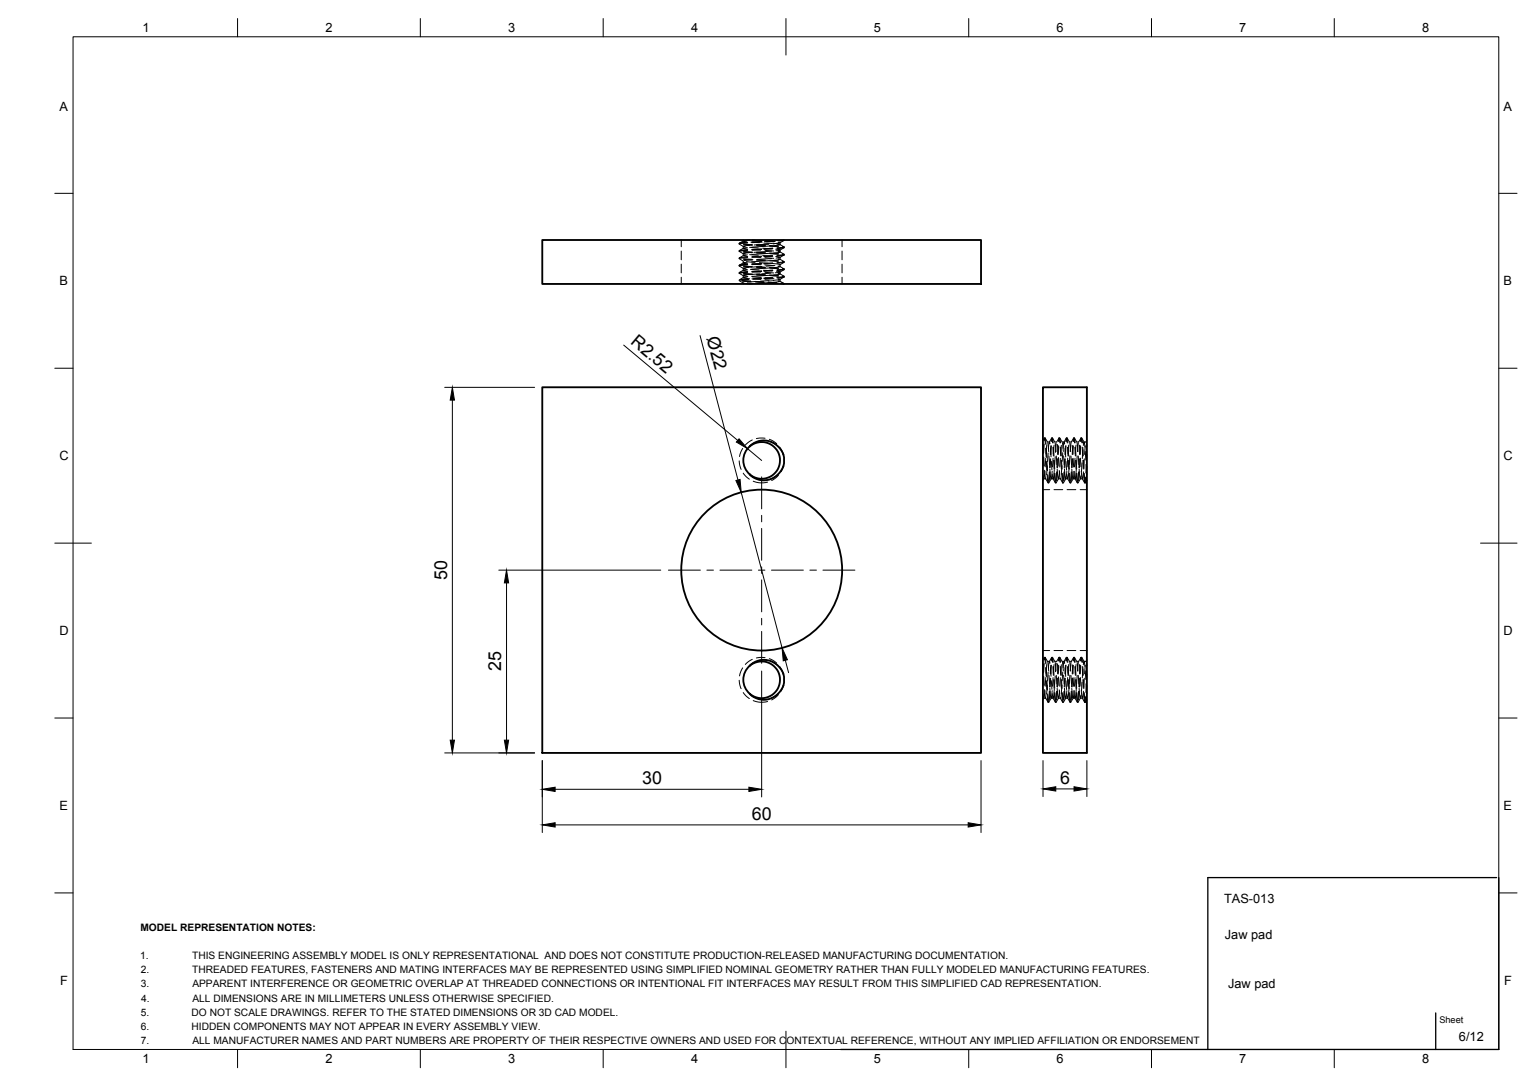
ISO-10303-21;
HEADER;
/* Generated by software containing ST-Developer
 * from STEP Tools, Inc. (www.steptools.com) 
 */

FILE_DESCRIPTION(
/* description */ (
'Independent guided parallel-jaw bracket clamp. Two12mm guide rods, re
placeable bronze sleeves, captured swiveling spindle, replaceable jaw 
pads and modeled M16x2 screw. Native slider/revolute joints linked2mm 
per revolution. Nominal opening0..122 with initial28mm. Base and two i
dentical supports welded. Standard fits, weld details and clamp load r
equire engineering selection.'),
/* implementation_level */ '2;1');

FILE_NAME(
/* name */ 'Jaw pad.step',
/* time_stamp */ '2026-11-14T09:15:44-08:00',
/* author */ (''),
/* organization */ (''),
/* preprocessor_version */ 'ST-DEVELOPER v20.2',
/* originating_system */ 'Autodesk Translation Framework v15.17.0.0',
/* authorisation */ '');

FILE_SCHEMA (('AUTOMOTIVE_DESIGN { 1 0 10303 214 3 1 1 }'));
ENDSEC;

DATA;
#10=MECHANICAL_DESIGN_GEOMETRIC_PRESENTATION_REPRESENTATION('',(#921),#105806);
#99=B_SPLINE_SURFACE_WITH_KNOTS('',3,3,((#87313,#87314,#87315,#87316,#87317,
#87318,#87319,#87320,#87321,#87322,#87323,#87324,#87325,#87326,#87327,#87328,
#87329,#87330,#87331,#87332,#87333,#87334,#87335,#87336,#87337,#87338,#87339,
#87340,#87341,#87342,#87343,#87344,#87345,#87346,#87347,#87348,#87349,#87350,
#87351,#87352,#87353,#87354,#87355),(#87356,#87357,#87358,#87359,#87360,
#87361,#87362,#87363,#87364,#87365,#87366,#87367,#87368,#87369,#87370,#87371,
#87372,#87373,#87374,#87375,#87376,#87377,#87378,#87379,#87380,#87381,#87382,
#87383,#87384,#87385,#87386,#87387,#87388,#87389,#87390,#87391,#87392,#87393,
#87394,#87395,#87396,#87397,#87398),(#87399,#87400,#87401,#87402,#87403,
#87404,#87405,#87406,#87407,#87408,#87409,#87410,#87411,#87412,#87413,#87414,
#87415,#87416,#87417,#87418,#87419,#87420,#87421,#87422,#87423,#87424,#87425,
#87426,#87427,#87428,#87429,#87430,#87431,#87432,#87433,#87434,#87435,#87436,
#87437,#87438,#87439,#87440,#87441),(#87442,#87443,#87444,#87445,#87446,
#87447,#87448,#87449,#87450,#87451,#87452,#87453,#87454,#87455,#87456,#87457,
#87458,#87459,#87460,#87461,#87462,#87463,#87464,#87465,#87466,#87467,#87468,
#87469,#87470,#87471,#87472,#87473,#87474,#87475,#87476,#87477,#87478,#87479,
#87480,#87481,#87482,#87483,#87484)),.UNSPECIFIED.,.F.,.F.,.F.,(4,4),(4,
1,1,1,1,1,1,1,1,1,1,1,1,1,1,1,1,1,1,1,1,1,1,1,1,1,1,1,1,1,1,1,1,1,1,1,1,
1,1,1,4),(-0.00051259176634298,0.0646339630657592),(11.8584762705415,12.8518902807105,
13.8447916991131,14.8376931175158,15.8305945359184,16.8234959543211,17.8163973727237,
18.8092987911264,19.802200209529,20.7951016279317,21.7880030463343,22.780904464737,
23.7738058831396,24.7667073015423,25.7596087199449,26.7525101383476,27.7454115567502,
28.7383129751529,29.7312143935555,30.7241158119582,31.7170172303608,32.7099186487635,
33.7028200671661,34.6957214855688,35.6886229039714,36.6815243223741,37.6744257407767,
38.6673271591794,39.660228577582,40.6531299959847,41.6460314143873,42.63893283279,
43.6318342511926,44.6247356695953,45.6176370879979,46.6105385064006,47.6034399248032,
48.5963413432059,49.5892427616085,50.5821441800112,51.5750455984138),
 .UNSPECIFIED.);
#100=B_SPLINE_SURFACE_WITH_KNOTS('',3,3,((#87669,#87670,#87671,#87672,#87673,
#87674,#87675,#87676,#87677,#87678,#87679,#87680,#87681,#87682,#87683,#87684,
#87685,#87686,#87687,#87688,#87689,#87690,#87691,#87692,#87693,#87694,#87695,
#87696,#87697,#87698,#87699,#87700,#87701,#87702,#87703,#87704,#87705,#87706,
#87707,#87708,#87709,#87710,#87711),(#87712,#87713,#87714,#87715,#87716,
#87717,#87718,#87719,#87720,#87721,#87722,#87723,#87724,#87725,#87726,#87727,
#87728,#87729,#87730,#87731,#87732,#87733,#87734,#87735,#87736,#87737,#87738,
#87739,#87740,#87741,#87742,#87743,#87744,#87745,#87746,#87747,#87748,#87749,
#87750,#87751,#87752,#87753,#87754),(#87755,#87756,#87757,#87758,#87759,
#87760,#87761,#87762,#87763,#87764,#87765,#87766,#87767,#87768,#87769,#87770,
#87771,#87772,#87773,#87774,#87775,#87776,#87777,#87778,#87779,#87780,#87781,
#87782,#87783,#87784,#87785,#87786,#87787,#87788,#87789,#87790,#87791,#87792,
#87793,#87794,#87795,#87796,#87797),(#87798,#87799,#87800,#87801,#87802,
#87803,#87804,#87805,#87806,#87807,#87808,#87809,#87810,#87811,#87812,#87813,
#87814,#87815,#87816,#87817,#87818,#87819,#87820,#87821,#87822,#87823,#87824,
#87825,#87826,#87827,#87828,#87829,#87830,#87831,#87832,#87833,#87834,#87835,
#87836,#87837,#87838,#87839,#87840)),.UNSPECIFIED.,.F.,.F.,.F.,(4,4),(4,
1,1,1,1,1,1,1,1,1,1,1,1,1,1,1,1,1,1,1,1,1,1,1,1,1,1,1,1,1,1,1,1,1,1,1,1,
1,1,1,4),(-0.000452026491598011,0.0646067404509306),(14.3984001269719,15.3913015453745,
16.3842029637772,17.3771043821798,18.3700058005825,19.3629072189851,20.3558086373878,
21.3487100557904,22.3416114741931,23.3345128925957,24.3274143109984,25.320315729401,
26.3132171478037,27.3061185662063,28.299019984609,29.2919214030116,30.2848228214142,
31.2777242398169,32.2706256582195,33.2635270766222,34.2564284950248,35.2493299134275,
36.2422313318301,37.2351327502328,38.2280341686354,39.2209355870381,40.2138370054407,
41.2067384238434,42.199639842246,43.1925412606487,44.1854426790513,45.178344097454,
46.1712455158566,47.1641469342593,48.1570483526619,49.1499497710646,50.1428511894672,
51.1357526078699,52.1286540262725,53.1215554446752,54.1144568630778),
 .UNSPECIFIED.);
#101=B_SPLINE_SURFACE_WITH_KNOTS('',3,3,((#88213,#88214,#88215,#88216,#88217,
#88218,#88219,#88220,#88221,#88222,#88223,#88224,#88225,#88226,#88227,#88228,
#88229,#88230,#88231,#88232,#88233,#88234,#88235,#88236,#88237,#88238,#88239,
#88240,#88241,#88242,#88243,#88244,#88245,#88246,#88247,#88248,#88249,#88250,
#88251,#88252,#88253,#88254,#88255),(#88256,#88257,#88258,#88259,#88260,
#88261,#88262,#88263,#88264,#88265,#88266,#88267,#88268,#88269,#88270,#88271,
#88272,#88273,#88274,#88275,#88276,#88277,#88278,#88279,#88280,#88281,#88282,
#88283,#88284,#88285,#88286,#88287,#88288,#88289,#88290,#88291,#88292,#88293,
#88294,#88295,#88296,#88297,#88298),(#88299,#88300,#88301,#88302,#88303,
#88304,#88305,#88306,#88307,#88308,#88309,#88310,#88311,#88312,#88313,#88314,
#88315,#88316,#88317,#88318,#88319,#88320,#88321,#88322,#88323,#88324,#88325,
#88326,#88327,#88328,#88329,#88330,#88331,#88332,#88333,#88334,#88335,#88336,
#88337,#88338,#88339,#88340,#88341),(#88342,#88343,#88344,#88345,#88346,
#88347,#88348,#88349,#88350,#88351,#88352,#88353,#88354,#88355,#88356,#88357,
#88358,#88359,#88360,#88361,#88362,#88363,#88364,#88365,#88366,#88367,#88368,
#88369,#88370,#88371,#88372,#88373,#88374,#88375,#88376,#88377,#88378,#88379,
#88380,#88381,#88382,#88383,#88384)),.UNSPECIFIED.,.F.,.F.,.F.,(4,4),(4,
1,1,1,1,1,1,1,1,1,1,1,1,1,1,1,1,1,1,1,1,1,1,1,1,1,1,1,1,1,1,1,1,1,1,1,1,
1,1,1,4),(-0.000512482261750268,0.0646339207422172),(11.858476380046,12.8518902807105,
13.8447916991131,14.8376931175158,15.8305945359184,16.8234959543211,17.8163973727237,
18.8092987911264,19.802200209529,20.7951016279317,21.7880030463343,22.780904464737,
23.7738058831396,24.7667073015423,25.7596087199449,26.7525101383476,27.7454115567502,
28.7383129751529,29.7312143935555,30.7241158119582,31.7170172303608,32.7099186487635,
33.7028200671661,34.6957214855688,35.6886229039714,36.6815243223741,37.6744257407767,
38.6673271591794,39.660228577582,40.6531299959847,41.6460314143873,42.63893283279,
43.6318342511926,44.6247356695953,45.6176370879979,46.6105385064006,47.6034399248032,
48.5963413432059,49.5892427616085,50.5821441800112,51.5750455984138),
 .UNSPECIFIED.);
#102=B_SPLINE_SURFACE_WITH_KNOTS('',3,3,((#88481,#88482,#88483,#88484,#88485,
#88486,#88487,#88488,#88489,#88490,#88491,#88492,#88493,#88494,#88495,#88496,
#88497,#88498,#88499,#88500,#88501,#88502,#88503,#88504,#88505,#88506,#88507,
#88508,#88509,#88510,#88511,#88512,#88513,#88514,#88515,#88516,#88517,#88518,
#88519,#88520,#88521,#88522,#88523),(#88524,#88525,#88526,#88527,#88528,
#88529,#88530,#88531,#88532,#88533,#88534,#88535,#88536,#88537,#88538,#88539,
#88540,#88541,#88542,#88543,#88544,#88545,#88546,#88547,#88548,#88549,#88550,
#88551,#88552,#88553,#88554,#88555,#88556,#88557,#88558,#88559,#88560,#88561,
#88562,#88563,#88564,#88565,#88566),(#88567,#88568,#88569,#88570,#88571,
#88572,#88573,#88574,#88575,#88576,#88577,#88578,#88579,#88580,#88581,#88582,
#88583,#88584,#88585,#88586,#88587,#88588,#88589,#88590,#88591,#88592,#88593,
#88594,#88595,#88596,#88597,#88598,#88599,#88600,#88601,#88602,#88603,#88604,
#88605,#88606,#88607,#88608,#88609),(#88610,#88611,#88612,#88613,#88614,
#88615,#88616,#88617,#88618,#88619,#88620,#88621,#88622,#88623,#88624,#88625,
#88626,#88627,#88628,#88629,#88630,#88631,#88632,#88633,#88634,#88635,#88636,
#88637,#88638,#88639,#88640,#88641,#88642,#88643,#88644,#88645,#88646,#88647,
#88648,#88649,#88650,#88651,#88652)),.UNSPECIFIED.,.F.,.F.,.F.,(4,4),(4,
1,1,1,1,1,1,1,1,1,1,1,1,1,1,1,1,1,1,1,1,1,1,1,1,1,1,1,1,1,1,1,1,1,1,1,1,
1,1,1,4),(-0.000452057026596796,0.0646067341429239),(14.3984001269719,15.3913015453745,
16.3842029637772,17.3771043821798,18.3700058005825,19.3629072189851,20.3558086373878,
21.3487100557904,22.3416114741931,23.3345128925957,24.3274143109984,25.320315729401,
26.3132171478037,27.3061185662063,28.299019984609,29.2919214030116,30.2848228214143,
31.2777242398169,32.2706256582196,33.2635270766222,34.2564284950248,35.2493299134275,
36.2422313318302,37.2351327502328,38.2280341686354,39.2209355870381,40.2138370054408,
41.2067384238434,42.199639842246,43.1925412606487,44.1854426790513,45.178344097454,
46.1712455158566,47.1641469342593,48.1570483526619,49.1499497710646,50.1428511894672,
51.1357526078699,52.1286540262725,53.1215554446752,54.1144568630778),
 .UNSPECIFIED.);
#646=B_SPLINE_CURVE_WITH_KNOTS('',3,(#79848,#79849,#79850,#79851,#79852,
#79853),.UNSPECIFIED.,.F.,.F.,(4,1,1,4),(49.3488291411432,49.5892427616085,
50.5821441800112,51.5750455984138),.UNSPECIFIED.);
#647=B_SPLINE_CURVE_WITH_KNOTS('',3,(#79856,#79857,#79858,#79859,#79860,
#79861,#79862,#79863,#79864,#79865,#79866,#79867,#79868,#79869,#79870,#79871,
#79872,#79873,#79874,#79875,#79876,#79877,#79878,#79879,#79880,#79881,#79882,
#79883,#79884,#79885,#79886,#79887,#79888,#79889,#79890,#79891,#79892,#79893,
#79894,#79895,#79896,#79897,#79898,#79899,#79900,#79901,#79902,#79903,#79904,
#79905,#79906,#79907,#79908,#79909,#79910,#79911,#79912,#79913,#79914,#79915,
#79916,#79917,#79918,#79919,#79920,#79921,#79922,#79923,#79924,#79925,#79926,
#79927,#79928,#79929,#79930,#79931,#79932,#79933,#79934,#79935,#79936,#79937,
#79938,#79939,#79940,#79941,#79942,#79943,#79944,#79945,#79946,#79947,#79948,
#79949),.UNSPECIFIED.,.F.,.F.,(4,3,3,3,3,3,3,3,3,3,3,3,3,3,3,3,3,3,3,3,
3,3,3,3,3,3,3,3,3,3,3,4),(49.3502889463907,49.4441975015053,49.5380445228534,
49.6318612588435,49.7256734628368,49.8195068771829,49.913444511682,50.0074415682785,
50.1015879207077,50.1428511894672,50.2372867432903,50.3315945427791,50.4258028696877,
50.5199427300037,50.6140476054246,50.7081429068457,50.8022540299028,50.896462754224,
50.9907255754947,51.0851349132109,51.1357526078699,51.2296146641935,51.3233516059659,
51.4201041343669,51.513680825887,51.6072278995691,51.700771432585,51.7943374920094,
51.888005499378,51.9817348168191,52.0756045098968,52.0973718331741),
 .UNSPECIFIED.);
#648=B_SPLINE_CURVE_WITH_KNOTS('',3,(#79955,#79956,#79957,#79958,#79959,
#79960,#79961,#79962,#79963,#79964,#79965,#79966,#79967,#79968,#79969,#79970,
#79971,#79972,#79973,#79974,#79975,#79976,#79977,#79978,#79979,#79980,#79981,
#79982,#79983,#79984,#79985,#79986,#79987,#79988,#79989,#79990,#79991,#79992,
#79993,#79994,#79995,#79996,#79997,#79998,#79999,#80000,#80001,#80002,#80003,
#80004,#80005,#80006,#80007,#80008,#80009,#80010,#80011,#80012,#80013,#80014,
#80015,#80016,#80017,#80018,#80019,#80020,#80021,#80022,#80023,#80024,#80025,
#80026,#80027,#80028,#80029,#80030,#80031,#80032,#80033,#80034,#80035,#80036,
#80037,#80038,#80039,#80040,#80041,#80042,#80043,#80044,#80045,#80046,#80047,
#80048,#80049,#80050,#80051,#80052,#80053,#80054,#80055,#80056,#80057,#80058,
#80059,#80060,#80061,#80062,#80063,#80064,#80065,#80066,#80067,#80068,#80069,
#80070,#80071,#80072,#80073,#80074,#80075,#80076,#80077,#80078,#80079,#80080,
#80081,#80082,#80083,#80084,#80085,#80086,#80087,#80088,#80089,#80090),
 .UNSPECIFIED.,.F.,.F.,(4,3,3,3,3,3,3,3,3,3,3,3,3,3,3,3,3,3,3,3,3,3,3,3,
3,3,3,3,3,3,3,3,3,3,3,3,3,3,3,3,3,3,3,3,3,4),(43.0667307346193,43.1606648282567,
43.2546046786335,43.3489120717733,43.4429916665771,43.5374129588849,43.6318342511926,
43.7260822914796,43.8202029945269,43.914224891448,44.0081800799522,44.1021014472809,
44.196014628203,44.2899452434255,44.3839769975109,44.4780646004317,44.5723031556115,
44.6247356695953,44.7190190327073,44.8131750079831,44.9072320802411,45.0012221569066,
45.0951782216785,45.1891258678985,45.2830906746415,45.3771559987717,45.4712768690749,
45.5655478938942,45.6176370879979,45.711922765816,45.806081403107,45.9001414759278,
45.9941350390331,46.0880948887982,46.1820466118188,46.2760157806679,46.3700858699236,
46.4642117401044,46.5584880801834,46.6105385064006,46.7087956950124,46.8068761968379,
46.9047435082123,47.0024820457555,47.1000741433132,47.1238898038469),
 .UNSPECIFIED.);
#649=B_SPLINE_CURVE_WITH_KNOTS('',3,(#80091,#80092,#80093,#80094,#80095,
#80096),.UNSPECIFIED.,.F.,.F.,(4,1,1,4),(47.1238910225188,47.6034399248032,
48.5963413432059,49.3488291411432),.UNSPECIFIED.);
#650=B_SPLINE_CURVE_WITH_KNOTS('',3,(#80098,#80099,#80100,#80101,#80102,
#80103,#80104,#80105,#80106,#80107,#80108,#80109,#80110,#80111,#80112,#80113,
#80114,#80115,#80116,#80117,#80118,#80119,#80120,#80121,#80122,#80123,#80124,
#80125,#80126,#80127,#80128,#80129,#80130,#80131,#80132,#80133,#80134,#80135,
#80136,#80137,#80138,#80139,#80140,#80141,#80142,#80143,#80144,#80145,#80146,
#80147,#80148,#80149,#80150,#80151,#80152,#80153,#80154,#80155,#80156,#80157,
#80158,#80159,#80160,#80161,#80162,#80163,#80164,#80165,#80166,#80167,#80168,
#80169,#80170,#80171,#80172,#80173,#80174,#80175,#80176),.UNSPECIFIED.,
 .F.,.F.,(4,3,3,3,3,3,3,3,3,3,3,3,3,3,3,3,3,3,3,3,3,3,3,3,3,3,4),(47.1238898038469,
47.1641469342593,47.2584303658851,47.3525864090342,47.4466435484464,47.5406336909398,
47.634589820696,47.728537530985,47.822502400809,47.9165677861539,48.010688716705,
48.104959799685,48.1570483526619,48.2513343067316,48.3454932219898,48.4395535740984,
48.5335474172898,48.6275075475247,48.7214595510516,48.8154290000951,48.9094993673677,
49.003625514735,49.0979021279899,49.1499497710646,49.2441083896016,49.3381288760954,
49.3502889463907),.UNSPECIFIED.);
#651=B_SPLINE_CURVE_WITH_KNOTS('',3,(#80177,#80178,#80179,#80180,#80181,
#80182,#80183,#80184,#80185,#80186,#80187,#80188,#80189,#80190,#80191,#80192,
#80193,#80194,#80195,#80196,#80197,#80198,#80199,#80200,#80201,#80202,#80203,
#80204,#80205,#80206,#80207,#80208,#80209,#80210,#80211,#80212,#80213,#80214,
#80215,#80216,#80217,#80218,#80219,#80220,#80221,#80222,#80223,#80224,#80225,
#80226,#80227,#80228,#80229,#80230,#80231,#80232,#80233,#80234,#80235,#80236,
#80237,#80238,#80239,#80240,#80241,#80242,#80243,#80244,#80245,#80246,#80247,
#80248,#80249,#80250,#80251,#80252,#80253,#80254,#80255,#80256,#80257,#80258,
#80259,#80260,#80261,#80262,#80263,#80264,#80265,#80266,#80267,#80268,#80269,
#80270,#80271,#80272,#80273,#80274,#80275,#80276,#80277,#80278,#80279,#80280,
#80281,#80282,#80283,#80284,#80285,#80286,#80287,#80288,#80289,#80290,#80291,
#80292,#80293,#80294,#80295,#80296,#80297,#80298,#80299,#80300,#80301,#80302,
#80303,#80304,#80305,#80306,#80307,#80308,#80309,#80310,#80311,#80312,#80313,
#80314,#80315),.UNSPECIFIED.,.F.,.F.,(4,3,3,3,3,3,3,3,3,3,3,3,3,3,3,3,3,
3,3,3,3,3,3,3,3,3,3,3,3,3,3,3,3,3,3,3,3,3,3,3,3,3,3,3,3,3,4),(43.066026510645,
43.1602903327225,43.1925412606487,43.2868033581566,43.3809381432706,43.474974128012,
43.5689433550273,43.6628787250892,43.7568058560264,43.8507503515564,43.9447957961315,
44.0388970021702,44.1331488907006,44.1854426790513,44.2797089639737,44.3738479257847,
44.4678880710968,44.5618614178521,44.6558008808659,44.7497320731119,44.8436805934253,
44.9377299831535,45.0318350950528,45.1260907899365,45.178344097454,45.2726125610302,
45.3667537503311,45.460796168269,45.5547718447446,45.6487136718209,45.7426472593229,
45.8365982029629,45.9306500434892,46.0247576252696,46.1190157953705,46.1712455158566,
46.2648963642522,46.3584203227472,46.4541040078507,46.5474647315296,46.6407947083202,
46.7341202531852,46.8315626407827,46.9250123202102,47.0185242448006,47.1121721912856,
47.1238898035752),.UNSPECIFIED.);
#652=B_SPLINE_CURVE_WITH_KNOTS('',3,(#80321,#80322,#80323,#80324,#80325,
#80326,#80327,#80328),.UNSPECIFIED.,.F.,.F.,(4,1,1,1,1,4),(36.7839151923342,
37.6744257407767,38.6673271591794,39.660228577582,40.6531299959847,40.8407044966673),
 .UNSPECIFIED.);
#653=B_SPLINE_CURVE_WITH_KNOTS('',3,(#80329,#80330,#80331,#80332,#80333,
#80334,#80335,#80336,#80337,#80338,#80339,#80340,#80341,#80342,#80343,#80344,
#80345,#80346,#80347,#80348,#80349,#80350,#80351,#80352,#80353,#80354,#80355,
#80356,#80357,#80358,#80359,#80360,#80361,#80362,#80363,#80364,#80365,#80366,
#80367,#80368,#80369,#80370,#80371,#80372,#80373,#80374,#80375,#80376,#80377,
#80378,#80379,#80380,#80381,#80382,#80383,#80384,#80385,#80386,#80387,#80388,
#80389,#80390,#80391,#80392,#80393,#80394,#80395,#80396,#80397,#80398,#80399,
#80400,#80401,#80402,#80403,#80404),.UNSPECIFIED.,.F.,.F.,(4,3,3,3,3,3,
3,3,3,3,3,3,3,3,3,3,3,3,3,3,3,3,3,3,3,4),(40.8407044966673,40.9334408145624,
41.0260857744486,41.1186819489494,41.2112563620308,41.3038360103078,41.3965054992974,
41.4892224724316,41.5820894658992,41.6460314143873,41.7402976892404,41.8344366411228,
41.9284767766575,42.0224501138978,42.1163895675618,42.2103207506336,42.3042692619587,
42.3983186430323,42.4924237464531,42.5866794332149,42.63893283279,42.7332102399409,
42.8273362432537,42.9213747388378,43.0153461234074,43.0667307346193),
 .UNSPECIFIED.);
#654=B_SPLINE_CURVE_WITH_KNOTS('',3,(#80406,#80407,#80408,#80409,#80410,
#80411,#80412,#80413,#80414,#80415,#80416,#80417,#80418,#80419,#80420,#80421,
#80422,#80423,#80424,#80425,#80426,#80427,#80428,#80429,#80430,#80431,#80432,
#80433,#80434,#80435,#80436,#80437,#80438,#80439,#80440,#80441,#80442,#80443,
#80444,#80445,#80446,#80447,#80448,#80449,#80450,#80451,#80452,#80453,#80454,
#80455,#80456,#80457,#80458,#80459,#80460,#80461,#80462,#80463,#80464,#80465,
#80466,#80467,#80468,#80469,#80470,#80471,#80472,#80473,#80474,#80475,#80476,
#80477,#80478,#80479,#80480,#80481),.UNSPECIFIED.,.F.,.F.,(4,3,3,3,3,3,
3,3,3,3,3,3,3,3,3,3,3,3,3,3,3,3,3,3,3,4),(40.8407044968899,40.9467955495431,
41.0533560438878,41.1605004844307,41.2067384238434,41.3010029060945,41.3951400761373,
41.4891784428115,41.5831500375655,41.6770877656947,41.7710172421922,41.8649640679288,
41.9590118053357,42.0531152864055,42.1473693999084,42.199639842246,42.2939131189821,
42.39042729294,42.4844558453375,42.57842255729,42.6723530801146,42.7707714377472,
42.8647438450981,42.9587494742861,43.0528504703067,43.066026510645),
 .UNSPECIFIED.);
#655=B_SPLINE_CURVE_WITH_KNOTS('',3,(#80482,#80483,#80484,#80485,#80486,
#80487,#80488,#80489,#80490,#80491,#80492,#80493,#80494,#80495,#80496,#80497,
#80498,#80499,#80500,#80501,#80502,#80503,#80504,#80505,#80506,#80507,#80508,
#80509,#80510,#80511,#80512,#80513,#80514,#80515,#80516,#80517,#80518,#80519,
#80520,#80521,#80522,#80523,#80524,#80525,#80526,#80527,#80528,#80529,#80530,
#80531,#80532,#80533,#80534,#80535,#80536,#80537,#80538,#80539,#80540,#80541,
#80542,#80543,#80544,#80545,#80546,#80547,#80548,#80549,#80550,#80551,#80552,
#80553,#80554,#80555,#80556,#80557,#80558,#80559,#80560,#80561,#80562,#80563,
#80564,#80565,#80566,#80567,#80568,#80569,#80570,#80571,#80572,#80573,#80574,
#80575,#80576,#80577,#80578,#80579,#80580,#80581,#80582,#80583,#80584,#80585,
#80586,#80587,#80588,#80589,#80590,#80591,#80592,#80593,#80594,#80595,#80596,
#80597,#80598,#80599,#80600,#80601,#80602,#80603,#80604,#80605,#80606,#80607,
#80608,#80609,#80610,#80611,#80612,#80613,#80614,#80615,#80616,#80617),
 .UNSPECIFIED.,.F.,.F.,(4,3,3,3,3,3,3,3,3,3,3,3,3,3,3,3,3,3,3,3,3,3,3,3,
3,3,3,3,3,3,3,3,3,3,3,3,3,3,3,3,3,3,3,3,3,4),(36.7832060675778,36.8771460542011,
36.9711833912529,37.0652707662042,37.159515690071,37.2351327502328,37.3293970162946,
37.423533972185,37.5175721269988,37.6115435141369,37.7054810373499,37.7994103118647,
37.8933569387886,37.987404483374,38.0815077747294,38.1757617052137,38.2280341686354,
38.3222984827916,38.4164354864537,38.5104736886573,38.6044451224285,38.6983826917895,
38.7923120119137,38.8862586838546,38.980306272289,39.0744096068966,39.1686635792801,
39.2209355870381,39.3152000037845,39.4093371109173,39.5033754173212,39.5973469559382,
39.6912846305034,39.785214056058,39.8791608335229,39.9732085269791,40.0673119664767,
40.1615660425125,40.2138370054407,40.3087260587235,40.4034841190128,40.498136016373,
40.5927004180163,40.6872130009825,40.7817120507751,40.8407044966673),
 .UNSPECIFIED.);
#656=B_SPLINE_CURVE_WITH_KNOTS('',3,(#80623,#80624,#80625,#80626,#80627,
#80628,#80629,#80630,#80631,#80632,#80633,#80634,#80635,#80636,#80637,#80638,
#80639,#80640,#80641,#80642,#80643,#80644,#80645,#80646,#80647,#80648,#80649,
#80650,#80651,#80652,#80653,#80654,#80655,#80656,#80657,#80658,#80659,#80660,
#80661,#80662,#80663,#80664,#80665,#80666,#80667,#80668,#80669,#80670,#80671,
#80672,#80673,#80674,#80675,#80676,#80677,#80678,#80679,#80680,#80681,#80682,
#80683,#80684,#80685,#80686,#80687,#80688,#80689,#80690,#80691,#80692,#80693,
#80694,#80695,#80696,#80697,#80698,#80699,#80700,#80701,#80702,#80703,#80704,
#80705,#80706,#80707,#80708,#80709,#80710,#80711,#80712,#80713,#80714,#80715,
#80716,#80717,#80718,#80719,#80720,#80721,#80722,#80723,#80724,#80725,#80726,
#80727,#80728,#80729,#80730,#80731,#80732,#80733,#80734,#80735,#80736,#80737,
#80738,#80739,#80740,#80741,#80742,#80743,#80744,#80745,#80746,#80747,#80748,
#80749,#80750,#80751,#80752,#80753,#80754,#80755,#80756,#80757,#80758,#80759,
#80760,#80761),.UNSPECIFIED.,.F.,.F.,(4,3,3,3,3,3,3,3,3,3,3,3,3,3,3,3,3,
3,3,3,3,3,3,3,3,3,3,3,3,3,3,3,3,3,3,3,3,3,3,3,3,3,3,3,3,3,4),(30.4995771796439,
30.5936923469732,30.6879535757028,30.7241158119582,30.8183801128246,30.9125171034347,
31.0065552928383,31.1005267142311,31.1944642714788,31.2883935797674,31.382340240163,
31.4763878175595,31.5704911414002,31.6647451035425,31.7170172303608,31.8112815307376,
31.9054185209583,31.999456710072,32.0934281313241,32.1873656885236,32.2812949968564,
32.3752416573885,32.4692892350613,32.5633925592575,32.6576465218765,32.7099186487635,
32.8041829508008,32.8983199426043,32.9923581332224,33.0863295558569,33.1802671143628,
33.2741964239248,33.3681430856079,33.4621906643065,33.5562939894593,33.6505479529175,
33.7028200671661,33.7957345289545,33.8909576115212,33.983639100071,34.0762648437623,
34.1688618579209,34.2660261908126,34.358690879243,34.4513987244999,34.5442184709287,
34.5575191894877),.UNSPECIFIED.);
#657=B_SPLINE_CURVE_WITH_KNOTS('',3,(#80762,#80763,#80764,#80765,#80766,
#80767,#80768),.UNSPECIFIED.,.F.,.F.,(4,1,1,1,4),(34.5575191894877,34.6957214855688,
35.6886229039714,36.6815243223741,36.7839151923342),.UNSPECIFIED.);
#658=B_SPLINE_CURVE_WITH_KNOTS('',3,(#80770,#80771,#80772,#80773,#80774,
#80775,#80776,#80777,#80778,#80779,#80780,#80781,#80782,#80783,#80784,#80785,
#80786,#80787,#80788,#80789,#80790,#80791,#80792,#80793,#80794,#80795,#80796,
#80797,#80798,#80799,#80800,#80801,#80802,#80803,#80804,#80805,#80806,#80807,
#80808,#80809,#80810,#80811,#80812,#80813,#80814,#80815,#80816,#80817,#80818,
#80819,#80820,#80821,#80822,#80823,#80824,#80825,#80826,#80827,#80828,#80829,
#80830,#80831,#80832,#80833,#80834,#80835,#80836,#80837,#80838,#80839,#80840,
#80841,#80842,#80843,#80844,#80845),.UNSPECIFIED.,.F.,.F.,(4,3,3,3,3,3,
3,3,3,3,3,3,3,3,3,3,3,3,3,3,3,3,3,3,3,4),(34.5575191894877,34.6509762726237,
34.7444023855498,34.8378236978267,34.9312663680164,35.024813540936,35.1184210075462,
35.2121773967878,35.2493299134275,35.3435942154267,35.4377312071913,35.5317693977697,
35.6257408203635,35.7196783788279,35.8136076883481,35.907554349989,36.0016019286447,
36.0957052537543,36.1899592171693,36.2422313318301,36.3364903162625,36.4306275703372,
36.5246573126976,36.6186236502166,36.7125643032859,36.7832060675778),
 .UNSPECIFIED.);
#659=B_SPLINE_CURVE_WITH_KNOTS('',3,(#80846,#80847,#80848,#80849,#80850,
#80851,#80852,#80853,#80854,#80855,#80856,#80857,#80858,#80859,#80860,#80861,
#80862,#80863,#80864,#80865,#80866,#80867,#80868,#80869,#80870,#80871,#80872,
#80873,#80874,#80875,#80876,#80877,#80878,#80879,#80880,#80881,#80882,#80883,
#80884,#80885,#80886,#80887,#80888,#80889,#80890,#80891,#80892,#80893,#80894,
#80895,#80896,#80897,#80898,#80899,#80900,#80901,#80902,#80903,#80904,#80905,
#80906,#80907,#80908,#80909,#80910,#80911,#80912,#80913,#80914,#80915,#80916,
#80917,#80918,#80919,#80920,#80921,#80922,#80923,#80924,#80925,#80926,#80927,
#80928,#80929,#80930,#80931,#80932,#80933,#80934,#80935,#80936,#80937,#80938,
#80939,#80940,#80941,#80942,#80943,#80944,#80945,#80946,#80947,#80948,#80949,
#80950,#80951,#80952,#80953,#80954,#80955,#80956,#80957,#80958,#80959,#80960,
#80961,#80962,#80963,#80964,#80965,#80966,#80967,#80968,#80969,#80970,#80971,
#80972,#80973,#80974,#80975,#80976,#80977,#80978,#80979,#80980,#80981),
 .UNSPECIFIED.,.F.,.F.,(4,3,3,3,3,3,3,3,3,3,3,3,3,3,3,3,3,3,3,3,3,3,3,3,
3,3,3,3,3,3,3,3,3,3,3,3,3,3,3,3,3,3,3,3,3,4),(30.5007342570418,30.5978580048887,
30.6918155551803,30.7857475823672,30.8796796947812,30.9736374934577,31.0677006444832,
31.1618270355242,31.2560954931774,31.2777242398169,31.37198855852,31.4661255672314,
31.5601637749738,31.6541352149827,31.748072791011,31.8420021182216,31.9359487976573,
32.0299963941584,32.1240997371679,32.2183537183927,32.2706256582195,32.3648899598653,
32.4590269513488,32.5530651417179,32.6470365642101,32.7409741226399,32.834903432192,
32.9288500939313,33.0228976727864,33.1170009981526,33.2112549619117,33.2635270766222,
33.3577913774699,33.4519283680602,33.5459665574427,33.6399379788128,33.733875536037,
33.8278048443011,33.9217515046713,34.0157990820411,34.1099024058543,34.2041563679683,
34.2564284950248,34.3705294643042,34.483246885964,34.5575191893194),
 .UNSPECIFIED.);
#660=B_SPLINE_CURVE_WITH_KNOTS('',3,(#80987,#80988,#80989,#80990,#80991,
#80992,#80993,#80994,#80995,#80996,#80997,#80998,#80999,#81000,#81001,#81002,
#81003,#81004,#81005,#81006,#81007,#81008,#81009,#81010,#81011,#81012,#81013,
#81014,#81015,#81016,#81017,#81018,#81019,#81020,#81021,#81022,#81023,#81024,
#81025,#81026,#81027,#81028,#81029,#81030,#81031,#81032,#81033,#81034,#81035,
#81036,#81037,#81038,#81039,#81040,#81041,#81042,#81043,#81044,#81045,#81046,
#81047,#81048,#81049,#81050,#81051,#81052,#81053,#81054,#81055,#81056,#81057,
#81058,#81059,#81060,#81061,#81062,#81063,#81064,#81065,#81066,#81067,#81068,
#81069,#81070,#81071,#81072,#81073,#81074,#81075,#81076,#81077,#81078,#81079,
#81080,#81081,#81082,#81083,#81084,#81085,#81086,#81087,#81088,#81089,#81090,
#81091,#81092,#81093,#81094,#81095,#81096,#81097,#81098,#81099,#81100,#81101,
#81102,#81103,#81104,#81105,#81106,#81107,#81108,#81109,#81110,#81111,#81112,
#81113,#81114,#81115,#81116,#81117,#81118,#81119,#81120,#81121,#81122),
 .UNSPECIFIED.,.F.,.F.,(4,3,3,3,3,3,3,3,3,3,3,3,3,3,3,3,3,3,3,3,3,3,3,3,
3,3,3,3,3,3,3,3,3,3,3,3,3,3,3,3,3,3,3,3,3,4),(24.2171287697742,24.3110579972788,
24.4049972141539,24.4990332006161,24.5931183154433,24.6873621161442,24.7667073015423,
24.8609713392762,24.9551080626337,25.0491459810612,25.1431171270508,25.2370544062596,
25.3309834342141,25.4249298123192,25.5189771061484,25.6130801452853,25.7073338237151,
25.7596087199449,25.8538731317554,25.948010234554,26.0420485372264,26.1360200730218,
26.2299577453297,26.3238871691935,26.4178339455366,26.5118816387426,26.605985078483,
26.7002391555322,26.7525101383476,26.8467744489231,26.9409114497427,27.0349496498394,
27.1289210826045,27.2228586516417,27.3167879721236,27.4107346451031,27.5047822356061,
27.598885572868,27.6931395487985,27.7454115567502,27.8431501300116,27.9407221181963,
28.0380986592781,28.1353586621332,28.2324911809566,28.2743338823081),
 .UNSPECIFIED.);
#661=B_SPLINE_CURVE_WITH_KNOTS('',3,(#81123,#81124,#81125,#81126,#81127,
#81128,#81129,#81130,#81131,#81132,#81133,#81134,#81135,#81136,#81137,#81138,
#81139,#81140,#81141,#81142,#81143,#81144,#81145,#81146,#81147,#81148,#81149,
#81150,#81151,#81152,#81153,#81154,#81155,#81156,#81157,#81158,#81159,#81160,
#81161,#81162,#81163,#81164,#81165,#81166,#81167,#81168,#81169,#81170,#81171,
#81172,#81173,#81174,#81175,#81176,#81177,#81178,#81179,#81180,#81181,#81182,
#81183,#81184,#81185,#81186,#81187,#81188,#81189,#81190,#81191,#81192,#81193,
#81194,#81195,#81196,#81197,#81198),.UNSPECIFIED.,.F.,.F.,(4,3,3,3,3,3,
3,3,3,3,3,3,3,3,3,3,3,3,3,3,3,3,3,3,3,4),(28.2743338824719,28.3741025974733,
28.4742017672452,28.5744720132341,28.6750305538962,28.7383129751529,28.8325772935425,
28.9267143019364,29.0207525093578,29.1147239490417,29.2086615247428,29.3025908516243,
29.3965375307294,29.4905851268997,29.5846884695777,29.6789424504733,29.7312143935555,
29.8272597418166,29.9213793242568,30.0154088681281,30.1093740916754,30.2069248636675,
30.3008613502571,30.3948068071614,30.4888131270942,30.4995771796439),
 .UNSPECIFIED.);
#662=B_SPLINE_CURVE_WITH_KNOTS('',3,(#81200,#81201,#81202,#81203,#81204,
#81205,#81206,#81207,#81208,#81209,#81210,#81211,#81212,#81213,#81214,#81215,
#81216,#81217,#81218,#81219,#81220,#81221,#81222,#81223,#81224,#81225,#81226,
#81227,#81228,#81229,#81230,#81231,#81232,#81233,#81234,#81235,#81236,#81237,
#81238,#81239,#81240,#81241,#81242,#81243,#81244,#81245,#81246,#81247,#81248,
#81249,#81250,#81251,#81252,#81253,#81254,#81255,#81256,#81257,#81258,#81259,
#81260,#81261,#81262,#81263,#81264,#81265,#81266,#81267,#81268,#81269,#81270,
#81271,#81272,#81273,#81274,#81275,#81276,#81277,#81278),.UNSPECIFIED.,
 .F.,.F.,(4,3,3,3,3,3,3,3,3,3,3,3,3,3,3,3,3,3,3,3,3,3,3,3,3,3,4),(28.2743338823081,
28.299019984609,28.3932843983051,28.4874215030106,28.5814598076082,28.675431345349,
28.7693690196139,28.8632984454436,28.9572452237596,29.0512929189365,29.1453963606499,
29.2396504396559,29.2919214030116,29.386185713534,29.4803227143046,29.5743609143565,
29.6683323470838,29.7622699160872,29.8561992365394,29.9501459094934,30.0441934999777,
30.138296837225,30.2325508131468,30.2848228214142,30.3790955387993,30.4732292275596,
30.5007342570418),.UNSPECIFIED.);
#663=B_SPLINE_CURVE_WITH_KNOTS('',3,(#81279,#81280,#81281,#81282,#81283,
#81284,#81285,#81286),.UNSPECIFIED.,.F.,.F.,(4,1,1,1,1,4),(24.2163565526082,
24.3274143109984,25.320315729401,26.3132171478037,27.3061185662063,28.2743305212408),
 .UNSPECIFIED.);
#664=B_SPLINE_CURVE_WITH_KNOTS('',3,(#81292,#81293,#81294,#81295,#81296,
#81297,#81298,#81299,#81300,#81301,#81302,#81303,#81304,#81305,#81306,#81307,
#81308,#81309,#81310,#81311,#81312,#81313,#81314,#81315,#81316,#81317,#81318,
#81319,#81320,#81321,#81322,#81323,#81324,#81325,#81326,#81327,#81328,#81329,
#81330,#81331,#81332,#81333,#81334,#81335,#81336,#81337,#81338,#81339,#81340,
#81341,#81342,#81343,#81344,#81345,#81346,#81347,#81348,#81349,#81350,#81351,
#81352,#81353,#81354,#81355,#81356,#81357,#81358,#81359,#81360,#81361,#81362,
#81363,#81364,#81365,#81366,#81367),.UNSPECIFIED.,.F.,.F.,(4,3,3,3,3,3,
3,3,3,3,3,3,3,3,3,3,3,3,3,3,3,3,3,3,3,4),(15.7079632679489,15.8009237578477,
15.893857092563,15.9867898679795,16.0797486734675,16.1728168231926,16.2659501333692,
16.3592325081837,16.3842029637772,16.4785800153725,16.5728296354092,16.6669801677573,
16.7610630054697,16.8551113545885,16.9491506824622,17.0432064416485,17.1373610257028,
17.2315703227792,17.3259275836065,17.3771043821798,17.4715162278345,17.5658095311508,
17.6600005887434,17.7541304460648,17.8482419729085,17.9335626655157),
 .UNSPECIFIED.);
#665=B_SPLINE_CURVE_WITH_KNOTS('',3,(#81369,#81370,#81371,#81372,#81373),
 .UNSPECIFIED.,.F.,.F.,(4,1,4),(14.3984001269719,15.3913015453745,15.7079549076759),
 .UNSPECIFIED.);
#666=B_SPLINE_CURVE_WITH_KNOTS('',3,(#81377,#81378,#81379,#81380,#81381,
#81382,#81383,#81384,#81385,#81386,#81387,#81388,#81389,#81390,#81391,#81392,
#81393,#81394,#81395,#81396,#81397,#81398,#81399,#81400,#81401,#81402,#81403,
#81404,#81405,#81406,#81407,#81408,#81409,#81410,#81411,#81412,#81413,#81414,
#81415,#81416,#81417,#81418,#81419,#81420,#81421,#81422,#81423,#81424,#81425,
#81426,#81427,#81428,#81429,#81430,#81431,#81432,#81433,#81434,#81435,#81436,
#81437,#81438,#81439,#81440),.UNSPECIFIED.,.F.,.F.,(4,3,3,3,3,3,3,3,3,3,
3,3,3,3,3,3,3,3,3,3,3,4),(13.8759339789434,13.969800122518,14.0635399756423,
14.1603091183765,14.2538857926958,14.3474317737851,14.4409731412004,14.5345359634685,
14.6281992027686,14.721922831302,14.8157856207819,14.8376931175158,14.9307866091373,
15.0279336914888,15.1207996479157,15.213612609684,15.306399441868,15.3991869778596,
15.4920484539258,15.5849536355179,15.6779807201868,15.7079632679489),
 .UNSPECIFIED.);
#667=B_SPLINE_CURVE_WITH_KNOTS('',3,(#81441,#81442,#81443,#81444,#81445,
#81446,#81447),.UNSPECIFIED.,.F.,.F.,(4,1,1,1,4),(15.7079632679489,15.8305945359184,
16.8234959543211,17.8163973727237,17.9344169320433),.UNSPECIFIED.);
#668=B_SPLINE_CURVE_WITH_KNOTS('',3,(#81453,#81454,#81455,#81456,#81457,
#81458),.UNSPECIFIED.,.F.,.F.,(4,1,1,4),(49.348829680871,49.5892427616085,
50.5821441800112,51.5750455984138),.UNSPECIFIED.);
#669=B_SPLINE_CURVE_WITH_KNOTS('',3,(#81461,#81462,#81463,#81464,#81465,
#81466,#81467,#81468,#81469,#81470,#81471,#81472,#81473,#81474,#81475,#81476,
#81477,#81478,#81479,#81480,#81481,#81482,#81483,#81484,#81485,#81486,#81487,
#81488,#81489,#81490,#81491,#81492,#81493,#81494,#81495,#81496,#81497,#81498,
#81499,#81500,#81501,#81502,#81503,#81504,#81505,#81506,#81507,#81508,#81509,
#81510,#81511,#81512,#81513,#81514,#81515,#81516,#81517,#81518,#81519,#81520,
#81521,#81522,#81523,#81524,#81525,#81526,#81527,#81528,#81529,#81530,#81531,
#81532,#81533,#81534,#81535,#81536,#81537,#81538,#81539,#81540,#81541,#81542,
#81543,#81544,#81545,#81546,#81547,#81548,#81549,#81550,#81551,#81552,#81553,
#81554),.UNSPECIFIED.,.F.,.F.,(4,3,3,3,3,3,3,3,3,3,3,3,3,3,3,3,3,3,3,3,
3,3,3,3,3,3,3,3,3,3,3,4),(49.3502890643105,49.4441980075936,49.5380454154391,
49.6318625367458,49.7256751244353,49.8195089204159,49.9134469314248,50.0074443620431,
50.1015910816633,50.1428511894672,50.2372865866975,50.3315942311916,50.4258024048822,
50.5199421152025,50.6140468426817,50.7081419983793,50.8022529780978,50.8964615635168,
50.9907242482063,51.0851334542348,51.1357526078699,51.2296137933982,51.3233498604106,
51.4201025481234,51.513678360408,51.6072245547518,51.7007672092646,51.7943323919603,
51.8879995295073,51.9817279801555,52.0755968171824,52.0973713621133),
 .UNSPECIFIED.);
#670=B_SPLINE_CURVE_WITH_KNOTS('',3,(#81560,#81561,#81562,#81563,#81564,
#81565,#81566,#81567,#81568,#81569,#81570,#81571,#81572,#81573,#81574,#81575,
#81576,#81577,#81578,#81579,#81580,#81581,#81582,#81583,#81584,#81585,#81586,
#81587,#81588,#81589,#81590,#81591,#81592,#81593,#81594,#81595,#81596,#81597,
#81598,#81599,#81600,#81601,#81602,#81603,#81604,#81605,#81606,#81607,#81608,
#81609,#81610,#81611,#81612,#81613,#81614,#81615,#81616,#81617,#81618,#81619,
#81620,#81621,#81622,#81623,#81624,#81625,#81626,#81627,#81628,#81629,#81630,
#81631,#81632,#81633,#81634,#81635,#81636,#81637,#81638,#81639,#81640,#81641,
#81642,#81643,#81644,#81645,#81646,#81647,#81648,#81649,#81650,#81651,#81652,
#81653,#81654,#81655,#81656,#81657,#81658,#81659,#81660,#81661,#81662,#81663,
#81664,#81665,#81666,#81667,#81668,#81669,#81670,#81671,#81672,#81673,#81674,
#81675,#81676,#81677,#81678,#81679,#81680,#81681,#81682,#81683,#81684,#81685,
#81686,#81687,#81688,#81689,#81690,#81691,#81692,#81693,#81694,#81695),
 .UNSPECIFIED.,.F.,.F.,(4,3,3,3,3,3,3,3,3,3,3,3,3,3,3,3,3,3,3,3,3,3,3,3,
3,3,3,3,3,3,3,3,3,3,3,3,3,3,3,3,3,3,3,3,3,4),(43.0667308900299,43.1606650120045,
43.2546048907049,43.3489122308268,43.4429918536228,43.5374130524077,43.6318342511926,
43.7260822246237,43.820202860722,43.9142246906894,44.0081798125043,44.102101113331,
44.1960142280177,44.2899447773498,44.3839764664652,44.4780640048411,44.5723024967692,
44.6247356695953,44.7190190673005,44.8131750768461,44.9072321830112,45.0012222929145,
45.0951783904985,45.1891260690686,45.2830909076629,45.3771562627026,45.4712771634273,
45.5655482176145,45.6176370879979,45.7119229052218,45.8060816827838,45.9001418965429,
45.994135600988,46.0880955922864,46.1820474568586,46.2760167671013,46.3700869966516,
46.4642130067074,46.5584894846377,46.6105385064006,46.708795281591,46.8068753700284,
46.9047422712377,47.0024804016383,47.1000720984711,47.1238898038469),
 .UNSPECIFIED.);
#671=B_SPLINE_CURVE_WITH_KNOTS('',3,(#81696,#81697,#81698,#81699,#81700,
#81701),.UNSPECIFIED.,.F.,.F.,(4,1,1,4),(47.1238910227372,47.6034399248032,
48.5963413432059,49.348829680871),.UNSPECIFIED.);
#672=B_SPLINE_CURVE_WITH_KNOTS('',3,(#81703,#81704,#81705,#81706,#81707,
#81708,#81709,#81710,#81711,#81712,#81713,#81714,#81715,#81716,#81717,#81718,
#81719,#81720,#81721,#81722,#81723,#81724,#81725,#81726,#81727,#81728,#81729,
#81730,#81731,#81732,#81733,#81734,#81735,#81736,#81737,#81738,#81739,#81740,
#81741,#81742,#81743,#81744,#81745,#81746,#81747,#81748,#81749,#81750,#81751,
#81752,#81753,#81754,#81755,#81756,#81757,#81758,#81759,#81760,#81761,#81762,
#81763,#81764,#81765,#81766,#81767,#81768,#81769,#81770,#81771,#81772,#81773,
#81774,#81775,#81776,#81777,#81778,#81779,#81780,#81781),.UNSPECIFIED.,
 .F.,.F.,(4,3,3,3,3,3,3,3,3,3,3,3,3,3,3,3,3,3,3,3,3,3,3,3,3,3,4),(47.1238898038469,
47.1641469342593,47.2584303255499,47.3525863287413,47.4466434286191,47.5406335323594,
47.6345896238593,47.728537296431,47.8225021291195,47.9165674784281,48.010688373512,
48.1049594222539,48.1570483526619,48.2513341440243,48.3454928955643,48.439553083177,
48.5335467614017,48.6275067264437,48.721458564756,48.8154278487685,48.9094980522921,
49.0036240363993,49.097900488756,49.1499497710646,49.2441087762897,49.3381296503042,
49.3502890643105),.UNSPECIFIED.);
#673=B_SPLINE_CURVE_WITH_KNOTS('',3,(#81782,#81783,#81784,#81785,#81786,
#81787,#81788,#81789,#81790,#81791,#81792,#81793,#81794,#81795,#81796,#81797,
#81798,#81799,#81800,#81801,#81802,#81803,#81804,#81805,#81806,#81807,#81808,
#81809,#81810,#81811,#81812,#81813,#81814,#81815,#81816,#81817,#81818,#81819,
#81820,#81821,#81822,#81823,#81824,#81825,#81826,#81827,#81828,#81829,#81830,
#81831,#81832,#81833,#81834,#81835,#81836,#81837,#81838,#81839,#81840,#81841,
#81842,#81843,#81844,#81845,#81846,#81847,#81848,#81849,#81850,#81851,#81852,
#81853,#81854,#81855,#81856,#81857,#81858,#81859,#81860,#81861,#81862,#81863,
#81864,#81865,#81866,#81867,#81868,#81869,#81870,#81871,#81872,#81873,#81874,
#81875,#81876,#81877,#81878,#81879,#81880,#81881,#81882,#81883,#81884,#81885,
#81886,#81887,#81888,#81889,#81890,#81891,#81892,#81893,#81894,#81895,#81896,
#81897,#81898,#81899,#81900,#81901,#81902,#81903,#81904,#81905,#81906,#81907,
#81908,#81909,#81910,#81911,#81912,#81913,#81914,#81915,#81916,#81917,#81918,
#81919,#81920),.UNSPECIFIED.,.F.,.F.,(4,3,3,3,3,3,3,3,3,3,3,3,3,3,3,3,3,
3,3,3,3,3,3,3,3,3,3,3,3,3,3,3,3,3,3,3,3,3,3,3,3,3,3,3,3,3,4),(43.0660266561136,
43.1602904721168,43.1925412606487,43.2868033719875,43.3809381709436,43.4749741695202,
43.5689434103037,43.6628787940877,43.7568059386841,43.8507504477941,43.9447959057476,
44.0388971250699,44.1331490266067,44.1854426790513,44.2797089580453,44.3738479140106,
44.4678880535664,44.56186139472,44.6558008522294,44.7497320390745,44.8436805540964,
44.9377299387299,45.0318350456382,45.1260907357409,45.178344097454,45.2726125283646,
45.3667536848057,45.4607960697361,45.5547717131217,45.6487135070695,45.7426470614455,
45.8365979720026,45.9306497797122,46.0247573287788,46.1190154666471,46.1712455158566,
46.2648964418328,46.3584204779971,46.4541041436943,46.5474649448372,46.6407949988889,
46.7341206207388,46.8315629164479,46.9250126715277,47.0185246713068,47.1121726918931,
47.1238898035752),.UNSPECIFIED.);
#674=B_SPLINE_CURVE_WITH_KNOTS('',3,(#81926,#81927,#81928,#81929,#81930,
#81931,#81932,#81933),.UNSPECIFIED.,.F.,.F.,(4,1,1,1,1,4),(36.7839153402381,
37.6744257407767,38.6673271591794,39.660228577582,40.6531299959847,40.8407044966673),
 .UNSPECIFIED.);
#675=B_SPLINE_CURVE_WITH_KNOTS('',3,(#81934,#81935,#81936,#81937,#81938,
#81939,#81940,#81941,#81942,#81943,#81944,#81945,#81946,#81947,#81948,#81949,
#81950,#81951,#81952,#81953,#81954,#81955,#81956,#81957,#81958,#81959,#81960,
#81961,#81962,#81963,#81964,#81965,#81966,#81967,#81968,#81969,#81970,#81971,
#81972,#81973,#81974,#81975,#81976,#81977,#81978,#81979,#81980,#81981,#81982,
#81983,#81984,#81985,#81986,#81987,#81988,#81989,#81990,#81991,#81992,#81993,
#81994,#81995,#81996,#81997,#81998,#81999,#82000,#82001,#82002,#82003,#82004,
#82005,#82006,#82007,#82008,#82009),.UNSPECIFIED.,.F.,.F.,(4,3,3,3,3,3,
3,3,3,3,3,3,3,3,3,3,3,3,3,3,3,3,3,3,3,4),(40.8407044966673,40.9334408037622,
41.0260857529454,41.1186819168029,41.2112563193078,41.3038359570828,41.3965054357324,
41.4892223986014,41.5820893820075,41.6460314143873,41.740297694324,41.8344366512188,
41.9284767916903,42.0224501337347,42.1163895921195,42.2103207798235,42.3042692956868,
42.3983186811306,42.4924237888327,42.5866794796959,42.63893283279,42.7332102678453,
42.8273362992733,42.9213748230855,43.0153462359771,43.0667308900299),
 .UNSPECIFIED.);
#676=B_SPLINE_CURVE_WITH_KNOTS('',3,(#82011,#82012,#82013,#82014,#82015,
#82016,#82017,#82018,#82019,#82020,#82021,#82022,#82023,#82024,#82025,#82026,
#82027,#82028,#82029,#82030,#82031,#82032,#82033,#82034,#82035,#82036,#82037,
#82038,#82039,#82040,#82041,#82042,#82043,#82044,#82045,#82046,#82047,#82048,
#82049,#82050,#82051,#82052,#82053,#82054,#82055,#82056,#82057,#82058,#82059,
#82060,#82061,#82062,#82063,#82064,#82065,#82066,#82067,#82068,#82069,#82070,
#82071,#82072,#82073,#82074,#82075,#82076,#82077,#82078,#82079,#82080,#82081,
#82082,#82083,#82084,#82085,#82086),.UNSPECIFIED.,.F.,.F.,(4,3,3,3,3,3,
3,3,3,3,3,3,3,3,3,3,3,3,3,3,3,3,3,3,3,4),(40.8407044968899,40.9467955512976,
41.0533560472971,41.1605004892804,41.2067384238434,41.3010029055445,41.3951400750534,
41.4891784412107,41.5831500354742,41.6770877631296,41.7710172391702,41.8649640644675,
41.9590118014643,42.0531152821399,42.147369395277,42.199639842246,42.2939131126729,
42.390427305603,42.4844558516208,42.5784225571918,42.6723530736409,42.7707714692591,
42.8647438703345,42.9587494932815,43.0528504831882,43.0660266561136),
 .UNSPECIFIED.);
#677=B_SPLINE_CURVE_WITH_KNOTS('',3,(#82087,#82088,#82089,#82090,#82091,
#82092,#82093,#82094,#82095,#82096,#82097,#82098,#82099,#82100,#82101,#82102,
#82103,#82104,#82105,#82106,#82107,#82108,#82109,#82110,#82111,#82112,#82113,
#82114,#82115,#82116,#82117,#82118,#82119,#82120,#82121,#82122,#82123,#82124,
#82125,#82126,#82127,#82128,#82129,#82130,#82131,#82132,#82133,#82134,#82135,
#82136,#82137,#82138,#82139,#82140,#82141,#82142,#82143,#82144,#82145,#82146,
#82147,#82148,#82149,#82150,#82151,#82152,#82153,#82154,#82155,#82156,#82157,
#82158,#82159,#82160,#82161,#82162,#82163,#82164,#82165,#82166,#82167,#82168,
#82169,#82170,#82171,#82172,#82173,#82174,#82175,#82176,#82177,#82178,#82179,
#82180,#82181,#82182,#82183,#82184,#82185,#82186,#82187,#82188,#82189,#82190,
#82191,#82192,#82193,#82194,#82195,#82196,#82197,#82198,#82199,#82200,#82201,
#82202,#82203,#82204,#82205,#82206,#82207,#82208,#82209,#82210,#82211,#82212,
#82213,#82214,#82215,#82216,#82217,#82218,#82219,#82220,#82221,#82222),
 .UNSPECIFIED.,.F.,.F.,(4,3,3,3,3,3,3,3,3,3,3,3,3,3,3,3,3,3,3,3,3,3,3,3,
3,3,3,3,3,3,3,3,3,3,3,3,3,3,3,3,3,3,3,3,3,4),(36.7832062156987,36.8771462021669,
36.9711835390891,37.0652709139485,37.1595158376815,37.2351327502328,37.3293970166289,
37.4235339728533,37.5175721280006,37.6115435154695,37.7054810390119,37.7994103138541,
37.8933569411026,37.9874044860071,38.0815077776789,38.1757617084725,38.2280341686354,
38.3222984827967,38.4164354864664,38.5104736886812,38.6044451224672,38.6983826918458,
38.7923120119903,38.8862586839539,38.9803062724145,39.0744096070503,39.1686635794652,
39.2209355870381,39.3152000026346,39.4093371086122,39.5033754138575,39.5973469513155,
39.691284624722,39.7852140491199,39.8791608254314,39.9732085177452,40.0673119561054,
40.1615660310226,40.2138370054408,40.3087260615032,40.4034841245682,40.4981360246953,
40.5927004290814,40.6872130147763,40.7817120672609,40.8407044966673),
 .UNSPECIFIED.);
#678=B_SPLINE_CURVE_WITH_KNOTS('',3,(#82228,#82229,#82230,#82231,#82232,
#82233,#82234,#82235,#82236,#82237,#82238,#82239,#82240,#82241,#82242,#82243,
#82244,#82245,#82246,#82247,#82248,#82249,#82250,#82251,#82252,#82253,#82254,
#82255,#82256,#82257,#82258,#82259,#82260,#82261,#82262,#82263,#82264,#82265,
#82266,#82267,#82268,#82269,#82270,#82271,#82272,#82273,#82274,#82275,#82276,
#82277,#82278,#82279,#82280,#82281,#82282,#82283,#82284,#82285,#82286,#82287,
#82288,#82289,#82290,#82291,#82292,#82293,#82294,#82295,#82296,#82297,#82298,
#82299,#82300,#82301,#82302,#82303,#82304,#82305,#82306,#82307,#82308,#82309,
#82310,#82311,#82312,#82313,#82314,#82315,#82316,#82317,#82318,#82319,#82320,
#82321,#82322,#82323,#82324,#82325,#82326,#82327,#82328,#82329,#82330,#82331,
#82332,#82333,#82334,#82335,#82336,#82337,#82338,#82339,#82340,#82341,#82342,
#82343,#82344,#82345,#82346,#82347,#82348,#82349,#82350,#82351,#82352,#82353,
#82354,#82355,#82356,#82357,#82358,#82359,#82360,#82361,#82362,#82363,#82364,
#82365,#82366),.UNSPECIFIED.,.F.,.F.,(4,3,3,3,3,3,3,3,3,3,3,3,3,3,3,3,3,
3,3,3,3,3,3,3,3,3,3,3,3,3,3,3,3,3,3,3,3,3,3,3,3,3,3,3,3,3,4),(30.4995773282354,
30.5936924956574,30.6879537244389,30.7241158119582,30.8183801128151,30.9125171034153,
31.0065552928083,31.1005267141897,31.1944642714255,31.2883935797018,31.3823402400845,
31.4763878174676,31.5704911412944,31.6647451034225,31.7170172303608,31.8112815307233,
31.90541852093,31.9994567100302,32.0934281312696,32.1873656884567,32.2812949967776,
32.3752416572982,32.4692892349602,32.5633925591461,32.6576465217556,32.7099186487635,
32.8041829507817,32.8983199425657,32.9923581331637,33.0863295557777,33.1802671142629,
33.274196423804,33.368143085466,33.462190664143,33.5562939892742,33.6505479527108,
33.7028200671661,33.7957345290918,33.8909576116413,33.9836391003293,34.0762648441589,
34.1688618584558,34.2660261912138,34.3586908797819,34.4513987251761,34.544218471741,
34.5575191894877),.UNSPECIFIED.);
#679=B_SPLINE_CURVE_WITH_KNOTS('',3,(#82367,#82368,#82369,#82370,#82371,
#82372,#82373),.UNSPECIFIED.,.F.,.F.,(4,1,1,1,4),(34.5575191894877,34.6957214855688,
35.6886229039714,36.6815243223741,36.7839153402381),.UNSPECIFIED.);
#680=B_SPLINE_CURVE_WITH_KNOTS('',3,(#82375,#82376,#82377,#82378,#82379,
#82380,#82381,#82382,#82383,#82384,#82385,#82386,#82387,#82388,#82389,#82390,
#82391,#82392,#82393,#82394,#82395,#82396,#82397,#82398,#82399,#82400,#82401,
#82402,#82403,#82404,#82405,#82406,#82407,#82408,#82409,#82410,#82411,#82412,
#82413,#82414,#82415,#82416,#82417,#82418,#82419,#82420,#82421,#82422,#82423,
#82424,#82425,#82426,#82427,#82428,#82429,#82430,#82431,#82432,#82433,#82434,
#82435,#82436,#82437,#82438,#82439,#82440,#82441,#82442,#82443,#82444,#82445,
#82446,#82447,#82448,#82449,#82450),.UNSPECIFIED.,.F.,.F.,(4,3,3,3,3,3,
3,3,3,3,3,3,3,3,3,3,3,3,3,3,3,3,3,3,3,4),(34.5575191894877,34.6509762726285,
34.7444023855589,34.8378236978393,34.9312663680321,35.0248135409537,35.1184210075654,
35.2121773968077,35.2493299134275,35.3435942154491,35.4377312072367,35.5317693978386,
35.6257408204563,35.7196783789453,35.8136076884902,35.9075543501558,36.0016019288369,
36.0957052539719,36.1899592174124,36.2422313318302,36.3364903160518,36.4306275699184,
36.5246573120852,36.618623649412,36.7125643023337,36.7832062156987),
 .UNSPECIFIED.);
#681=B_SPLINE_CURVE_WITH_KNOTS('',3,(#82451,#82452,#82453,#82454,#82455,
#82456,#82457,#82458,#82459,#82460,#82461,#82462,#82463,#82464,#82465,#82466,
#82467,#82468,#82469,#82470,#82471,#82472,#82473,#82474,#82475,#82476,#82477,
#82478,#82479,#82480,#82481,#82482,#82483,#82484,#82485,#82486,#82487,#82488,
#82489,#82490,#82491,#82492,#82493,#82494,#82495,#82496,#82497,#82498,#82499,
#82500,#82501,#82502,#82503,#82504,#82505,#82506,#82507,#82508,#82509,#82510,
#82511,#82512,#82513,#82514,#82515,#82516,#82517,#82518,#82519,#82520,#82521,
#82522,#82523,#82524,#82525,#82526,#82527,#82528,#82529,#82530,#82531,#82532,
#82533,#82534,#82535,#82536,#82537,#82538,#82539,#82540,#82541,#82542,#82543,
#82544,#82545,#82546,#82547,#82548,#82549,#82550,#82551,#82552,#82553,#82554,
#82555,#82556,#82557,#82558,#82559,#82560,#82561,#82562,#82563,#82564,#82565,
#82566,#82567,#82568,#82569,#82570,#82571,#82572,#82573,#82574,#82575,#82576,
#82577,#82578,#82579,#82580,#82581,#82582,#82583,#82584,#82585,#82586),
 .UNSPECIFIED.,.F.,.F.,(4,3,3,3,3,3,3,3,3,3,3,3,3,3,3,3,3,3,3,3,3,3,3,3,
3,3,3,3,3,3,3,3,3,3,3,3,3,3,3,3,3,3,3,3,3,4),(30.5007344054827,30.5978581347745,
30.6918156853378,30.7857477128349,30.8796798255972,30.9736376246596,31.067700776091,
31.161827167571,31.2560956256276,31.2777242398169,31.3719885583348,31.4661255668587,
31.5601637744116,31.6541352142286,31.7480727900637,31.8420021170799,31.9359487963204,
32.0299963926262,32.1240997354399,32.2183537164704,32.2706256582196,32.3648899598909,
32.4590269513998,32.5530651417941,32.6470365643113,32.7409741227658,32.8349034323424,
32.928850094106,33.0228976729848,33.1170009983745,33.2112549621563,33.2635270766222,
33.3577913774809,33.4519283680829,33.5459665574779,33.6399379788614,33.7338755360994,
33.8278048443779,33.9217515047631,34.0157990821487,34.109902405978,34.2041563681087,
34.2564284950248,34.3705294643833,34.48324688611,34.5575191893195),
 .UNSPECIFIED.);
#682=B_SPLINE_CURVE_WITH_KNOTS('',3,(#82592,#82593,#82594,#82595,#82596,
#82597,#82598,#82599,#82600,#82601,#82602,#82603,#82604,#82605,#82606,#82607,
#82608,#82609,#82610,#82611,#82612,#82613,#82614,#82615,#82616,#82617,#82618,
#82619,#82620,#82621,#82622,#82623,#82624,#82625,#82626,#82627,#82628,#82629,
#82630,#82631,#82632,#82633,#82634,#82635,#82636,#82637,#82638,#82639,#82640,
#82641,#82642,#82643,#82644,#82645,#82646,#82647,#82648,#82649,#82650,#82651,
#82652,#82653,#82654,#82655,#82656,#82657,#82658,#82659,#82660,#82661,#82662,
#82663,#82664,#82665,#82666,#82667,#82668,#82669,#82670,#82671,#82672,#82673,
#82674,#82675,#82676,#82677,#82678,#82679,#82680,#82681,#82682,#82683,#82684,
#82685,#82686,#82687,#82688,#82689,#82690,#82691,#82692,#82693,#82694,#82695,
#82696,#82697,#82698,#82699,#82700,#82701,#82702,#82703,#82704,#82705,#82706,
#82707,#82708,#82709,#82710,#82711,#82712,#82713,#82714,#82715,#82716,#82717,
#82718,#82719,#82720,#82721,#82722,#82723,#82724,#82725,#82726,#82727),
 .UNSPECIFIED.,.F.,.F.,(4,3,3,3,3,3,3,3,3,3,3,3,3,3,3,3,3,3,3,3,3,3,3,3,
3,3,3,3,3,3,3,3,3,3,3,3,3,3,3,3,3,3,3,3,3,4),(24.2171289178558,24.3110581457589,
24.4049973630879,24.4990333500489,24.5931184654238,24.687362266644,24.7667073015423,
24.8609713374983,24.9551080590497,25.0491459756451,25.1431171197724,25.2370543971007,
25.3309834231588,25.4249297993533,25.5189770912628,25.6130801284721,25.7073338049799,
25.7596087199449,25.8538731327047,25.9480102364635,26.042048540105,26.1360200768798,
26.2299577501729,26.3238871750263,26.4178339523628,26.511881646561,26.6059850872946,
26.7002391653289,26.7525101383476,26.8467744488966,26.9409114496918,27.0349496497661,
27.1289210825126,27.2228586515332,27.3167879720004,27.4107346449676,27.5047822354614,
27.5988855727163,27.6931395486428,27.7454115567502,27.8431501298669,27.9407221178994,
28.0380986588194,28.135358661508,28.2324911801573,28.2743338823081),
 .UNSPECIFIED.);
#683=B_SPLINE_CURVE_WITH_KNOTS('',3,(#82728,#82729,#82730,#82731,#82732,
#82733,#82734,#82735,#82736,#82737,#82738,#82739,#82740,#82741,#82742,#82743,
#82744,#82745,#82746,#82747,#82748,#82749,#82750,#82751,#82752,#82753,#82754,
#82755,#82756,#82757,#82758,#82759,#82760,#82761,#82762,#82763,#82764,#82765,
#82766,#82767,#82768,#82769,#82770,#82771,#82772,#82773,#82774,#82775,#82776,
#82777,#82778,#82779,#82780,#82781,#82782,#82783,#82784,#82785,#82786,#82787,
#82788,#82789,#82790,#82791,#82792,#82793,#82794,#82795,#82796,#82797,#82798,
#82799,#82800,#82801,#82802,#82803),.UNSPECIFIED.,.F.,.F.,(4,3,3,3,3,3,
3,3,3,3,3,3,3,3,3,3,3,3,3,3,3,3,3,3,3,4),(28.2743338824719,28.3741025969876,
28.4742017662569,28.574472011735,28.6750305518817,28.7383129751529,28.8325772937002,
28.9267143022538,29.0207525098367,29.1147239496841,29.2086615255499,29.3025908525969,
29.3965375318683,29.490585128205,29.5846884710498,29.678942452111,29.7312143935555,
29.8272597603905,29.9213793427822,30.0154088866135,30.1093741101295,30.2069249146559,
30.3008614012555,30.3948068581838,30.4888131781989,30.4995773282354),
 .UNSPECIFIED.);
#684=B_SPLINE_CURVE_WITH_KNOTS('',3,(#82805,#82806,#82807,#82808,#82809,
#82810,#82811,#82812,#82813,#82814,#82815,#82816,#82817,#82818,#82819,#82820,
#82821,#82822,#82823,#82824,#82825,#82826,#82827,#82828,#82829,#82830,#82831,
#82832,#82833,#82834,#82835,#82836,#82837,#82838,#82839,#82840,#82841,#82842,
#82843,#82844,#82845,#82846,#82847,#82848,#82849,#82850,#82851,#82852,#82853,
#82854,#82855,#82856,#82857,#82858,#82859,#82860,#82861,#82862,#82863,#82864,
#82865,#82866,#82867,#82868,#82869,#82870,#82871,#82872,#82873,#82874,#82875,
#82876,#82877,#82878,#82879,#82880,#82881,#82882,#82883),.UNSPECIFIED.,
 .F.,.F.,(4,3,3,3,3,3,3,3,3,3,3,3,3,3,3,3,3,3,3,3,3,3,3,3,3,3,4),(28.2743338823081,
28.299019984609,28.3932843971923,28.4874215007725,28.5814598042337,28.6754313408263,
28.7693690139363,28.8632984386057,28.9572452157574,29.0512929097711,29.14539635032,
29.2396504281712,29.2919214030116,29.3861857135655,29.4803227143652,29.5743609144437,
29.6683323471937,29.7622699162173,29.8561992366871,29.9501459096564,30.044193500152,
30.1382968374083,30.2325508133356,30.2848228214143,30.3790955390654,30.4732292280887,
30.5007344054827),.UNSPECIFIED.);
#685=B_SPLINE_CURVE_WITH_KNOTS('',3,(#82884,#82885,#82886,#82887,#82888,
#82889,#82890,#82891),.UNSPECIFIED.,.F.,.F.,(4,1,1,1,1,4),(24.2163566964775,
24.3274143109984,25.320315729401,26.3132171478037,27.3061185662063,28.2743305207902),
 .UNSPECIFIED.);
#686=B_SPLINE_CURVE_WITH_KNOTS('',3,(#82897,#82898,#82899,#82900,#82901,
#82902,#82903,#82904,#82905,#82906,#82907,#82908,#82909,#82910,#82911,#82912,
#82913,#82914,#82915,#82916,#82917,#82918,#82919,#82920,#82921,#82922,#82923,
#82924,#82925,#82926,#82927,#82928,#82929,#82930,#82931,#82932,#82933,#82934,
#82935,#82936,#82937,#82938,#82939,#82940,#82941,#82942,#82943,#82944,#82945,
#82946,#82947,#82948,#82949,#82950,#82951,#82952,#82953,#82954,#82955,#82956,
#82957,#82958,#82959,#82960,#82961,#82962,#82963,#82964,#82965,#82966,#82967,
#82968,#82969,#82970,#82971,#82972),.UNSPECIFIED.,.F.,.F.,(4,3,3,3,3,3,
3,3,3,3,3,3,3,3,3,3,3,3,3,3,3,3,3,3,3,4),(15.707963267949,15.8009257619914,
15.8938611105031,15.9867959077331,16.0797567414188,16.1728269203555,16.2659622627033,
16.3592466607815,16.3842029637772,16.4785791144072,16.5728278228513,16.66697743437,
16.7610593414545,16.8551067542938,16.9491451414462,17.043199956675,17.1373535976475,
17.2315619508221,17.3259182756567,17.3771043821798,17.4715160967997,17.565809265615,
17.6600001838905,17.7541298992212,17.8482412804839,17.933562797591),
 .UNSPECIFIED.);
#687=B_SPLINE_CURVE_WITH_KNOTS('',3,(#82974,#82975,#82976,#82977,#82978),
 .UNSPECIFIED.,.F.,.F.,(4,1,4),(14.3984001269719,15.3913015453745,15.7079549083771),
 .UNSPECIFIED.);
#688=B_SPLINE_CURVE_WITH_KNOTS('',3,(#82982,#82983,#82984,#82985,#82986,
#82987,#82988,#82989,#82990,#82991,#82992,#82993,#82994,#82995,#82996,#82997,
#82998,#82999,#83000,#83001,#83002,#83003,#83004,#83005,#83006,#83007,#83008,
#83009,#83010,#83011,#83012,#83013,#83014,#83015,#83016,#83017,#83018,#83019,
#83020,#83021,#83022,#83023,#83024,#83025,#83026,#83027,#83028,#83029,#83030,
#83031,#83032,#83033,#83034,#83035,#83036,#83037,#83038,#83039,#83040,#83041,
#83042,#83043,#83044,#83045),.UNSPECIFIED.,.F.,.F.,(4,3,3,3,3,3,3,3,3,3,
3,3,3,3,3,3,3,3,3,3,3,4),(13.8759339770166,13.969800853008,14.063541445323,
14.1603104043471,14.2538878301271,14.3474345658592,14.4409766902909,14.534540271142,
14.6282042675365,14.7219286532259,14.8157921941949,14.8376931175158,14.9307866091952,
15.0279336915394,15.1207996554847,15.2136126275113,15.3063994726962,15.3991870244372,
15.4920485203054,15.5849537240745,15.677980834301,15.707963267949),
 .UNSPECIFIED.);
#689=B_SPLINE_CURVE_WITH_KNOTS('',3,(#83046,#83047,#83048,#83049,#83050,
#83051,#83052),.UNSPECIFIED.,.F.,.F.,(4,1,1,1,4),(15.707963267949,15.8305945359184,
16.8234959543211,17.8163973727237,17.934417062947),.UNSPECIFIED.);
#690=B_SPLINE_CURVE_WITH_KNOTS('',3,(#83058,#83059,#83060,#83061,#83062,
#83063,#83064,#83065,#83066,#83067),.UNSPECIFIED.,.F.,.F.,(4,2,2,2,4),(-0.0891794197387037,
-0.0404384534220769,-0.012183279177373,-0.0054070073603356,0.),
 .UNSPECIFIED.);
#691=B_SPLINE_CURVE_WITH_KNOTS('',3,(#83070,#83071,#83072,#83073,#83074,
#83075,#83076,#83077,#83078,#83079,#83080,#83081,#83082,#83083,#83084,#83085,
#83086,#83087,#83088,#83089,#83090,#83091,#83092,#83093,#83094,#83095,#83096,
#83097,#83098,#83099,#83100,#83101,#83102,#83103,#83104,#83105,#83106,#83107,
#83108,#83109,#83110,#83111,#83112,#83113,#83114,#83115,#83116,#83117,#83118,
#83119,#83120,#83121,#83122,#83123,#83124,#83125),.UNSPECIFIED.,.F.,.F.,
(4,2,2,2,2,2,2,2,2,2,2,2,2,2,2,2,2,2,2,2,2,2,2,2,2,2,2,4),(-2.19718104682751,
-2.19645858152794,-2.18932165309502,-2.15032845111742,-2.11832204261695,
-2.09604578914239,-2.08390596653947,-2.07287258854925,-2.05759738399719,
-2.01446578143502,-1.98527138501252,-1.96806044418142,-1.96043522719183,
-1.95409249138337,-1.94439702344743,-1.89993652966697,-1.86954642289234,
-1.8480399631896,-1.83610215377107,-1.82515811572939,-1.80990179286441,
-1.75224698036085,-1.73058071279881,-1.71614874303442,-1.70904218146749,
-1.70280042621923,-1.69271885646605,-1.67608637462986),.UNSPECIFIED.);
#692=B_SPLINE_CURVE_WITH_KNOTS('',3,(#83131,#83132,#83133,#83134,#83135,
#83136,#83137,#83138,#83139,#83140,#83141,#83142,#83143,#83144,#83145,#83146,
#83147,#83148,#83149,#83150,#83151,#83152,#83153,#83154,#83155,#83156,#83157,
#83158,#83159,#83160,#83161,#83162,#83163,#83164,#83165,#83166,#83167,#83168,
#83169,#83170,#83171,#83172,#83173,#83174,#83175,#83176,#83177,#83178,#83179,
#83180,#83181,#83182,#83183,#83184,#83185,#83186,#83187,#83188,#83189,#83190,
#83191,#83192,#83193,#83194,#83195,#83196,#83197,#83198,#83199,#83200,#83201,
#83202,#83203,#83204,#83205,#83206,#83207,#83208,#83209,#83210,#83211,#83212,
#83213,#83214,#83215,#83216,#83217,#83218,#83219,#83220,#83221,#83222,#83223,
#83224,#83225,#83226,#83227,#83228,#83229,#83230,#83231,#83232,#83233,#83234,
#83235,#83236,#83237,#83238,#83239,#83240,#83241,#83242,#83243,#83244,#83245,
#83246,#83247,#83248,#83249,#83250,#83251,#83252,#83253,#83254,#83255,#83256,
#83257,#83258,#83259,#83260,#83261,#83262,#83263,#83264,#83265,#83266,#83267,
#83268,#83269,#83270,#83271,#83272,#83273,#83274,#83275,#83276,#83277,#83278,
#83279,#83280,#83281,#83282,#83283,#83284,#83285,#83286,#83287,#83288,#83289,
#83290,#83291,#83292,#83293,#83294,#83295,#83296,#83297,#83298,#83299,#83300,
#83301,#83302,#83303,#83304,#83305,#83306,#83307,#83308,#83309,#83310,#83311),
 .UNSPECIFIED.,.F.,.F.,(4,3,3,3,3,3,3,3,3,3,3,3,3,3,3,3,3,3,3,3,3,3,3,3,
3,3,3,3,3,3,3,3,3,3,3,3,3,3,3,3,3,3,3,3,3,3,3,3,3,3,3,3,3,3,3,3,3,3,3,3,
4),(33.079934870469,33.1787177894596,33.2774733872199,33.3762313802265,
33.4750880185667,33.5739937416401,33.6730724278617,33.7586482256901,33.8577570182368,
33.9567262428988,34.0560791680481,34.1548734814301,34.253635757772,34.3523957095728,
34.4521841932028,34.5510854562345,34.6513175501636,34.7515496440927,34.8505116619609,
34.9493335207729,35.0487232134882,35.1473697968322,35.2459845308404,35.3445973248064,
35.4445607592287,35.5433172973594,35.6438841799274,35.7444510624954,35.8437171136992,
35.9428428037689,36.0421565134101,36.1411042244635,36.2400184017015,36.3389285537144,
36.4385345355103,36.5375803171594,36.6374663990287,36.737352480898,36.83654561436,
36.9356010198157,37.0349326297513,37.1338168838387,37.2326702948661,37.3315224367231,
37.4312053023675,37.5302003418486,37.6302271205746,37.7302538993007,37.8283438241589,
37.9262933983847,38.0259011382996,38.1236806968838,38.2214320150539,38.3191859967539,
38.4201783269913,38.518095715075,38.6206255163892,38.7231553177033,38.8550550269612,
38.9837128251521,39.0086643481542),.UNSPECIFIED.);
#693=B_SPLINE_CURVE_WITH_KNOTS('',3,(#83312,#83313,#83314,#83315,#83316,
#83317,#83318,#83319,#83320,#83321,#83322,#83323,#83324,#83325),
 .UNSPECIFIED.,.F.,.F.,(4,2,2,2,2,2,4),(-0.178828740417439,-0.148696555674604,
-0.131054670705411,-0.117602908728372,-0.105711018511371,-0.0894577948770551,
-0.0891794197387037),.UNSPECIFIED.);
#694=B_SPLINE_CURVE_WITH_KNOTS('',3,(#83326,#83327,#83328,#83329,#83330,
#83331,#83332,#83333,#83334,#83335,#83336,#83337,#83338,#83339,#83340,#83341,
#83342,#83343,#83344,#83345,#83346,#83347,#83348,#83349,#83350,#83351,#83352,
#83353,#83354,#83355,#83356,#83357,#83358,#83359,#83360,#83361,#83362,#83363,
#83364,#83365,#83366,#83367,#83368,#83369,#83370,#83371,#83372,#83373,#83374,
#83375,#83376,#83377,#83378,#83379,#83380,#83381,#83382,#83383,#83384,#83385,
#83386,#83387,#83388,#83389,#83390,#83391,#83392,#83393,#83394,#83395,#83396,
#83397,#83398,#83399,#83400,#83401,#83402,#83403,#83404,#83405,#83406,#83407,
#83408,#83409,#83410,#83411,#83412,#83413,#83414,#83415,#83416,#83417,#83418,
#83419,#83420,#83421,#83422,#83423,#83424,#83425,#83426,#83427,#83428,#83429,
#83430,#83431,#83432,#83433,#83434,#83435,#83436,#83437,#83438,#83439,#83440,
#83441,#83442,#83443,#83444,#83445,#83446,#83447,#83448,#83449,#83450,#83451,
#83452,#83453,#83454,#83455,#83456,#83457,#83458,#83459,#83460,#83461,#83462,
#83463,#83464,#83465,#83466,#83467,#83468,#83469,#83470,#83471,#83472,#83473,
#83474,#83475,#83476,#83477),.UNSPECIFIED.,.F.,.F.,(4,2,2,2,2,2,2,2,2,2,
2,2,2,2,2,2,2,2,2,2,2,2,2,2,2,2,2,2,2,2,2,2,2,2,2,2,2,2,2,2,2,2,2,2,2,2,
2,2,2,2,2,2,2,2,2,2,2,2,2,2,2,2,2,2,2,2,2,2,2,2,2,2,2,2,2,4),(-1.67608637462986,
-1.65687732929873,-1.62150669571193,-1.59809880019172,-1.58595568834587,
-1.57523193825967,-1.56120312823587,-1.50340369105419,-1.4804032775575,
-1.46544522879122,-1.45828994231978,-1.45207772281957,-1.44223763959186,
-1.39973102571514,-1.36815220530213,-1.3461400200849,-1.33414089633424,
-1.32325608559398,-1.30827425353094,-1.27361347699094,-1.24298186377057,
-1.22589234207498,-1.21355300420792,-1.20681156948572,-1.20020487396986,
-1.18853404833856,-1.13693688228772,-1.10104754529816,-1.08748866548457,
-1.07675204196991,-1.06397420315739,-1.03626793101884,-0.985730691755481,
-0.96646465694695,-0.9585409114734,-0.95239260804874,-0.943735945622945,
-0.914830519314583,-0.852511535606085,-0.839536044514228,-0.828619201443956,
-0.816856476100891,-0.796170252696613,-0.767688481950534,-0.718690361686391,
-0.70950920017578,-0.703315870755706,-0.695744660943167,-0.678234129685828,
-0.648195237002004,-0.604153246978942,-0.588788611265734,-0.577871755610879,
-0.566061605072287,-0.545134452920513,-0.516104985097223,-0.468429542707585,
-0.459108393407661,-0.45289439172849,-0.445391289165089,-0.428359750747527,
-0.399772116764656,-0.353548048375749,-0.338224087500789,-0.32731626767606,
-0.315499073747651,-0.294510667550791,-0.265342259784795,-0.217920436646892,
-0.208570811893949,-0.202356109969582,-0.194876006641539,-0.177994331427986,
-0.149845137636229,-0.102902361229971,-0.0902464959671978),
 .UNSPECIFIED.);
#695=B_SPLINE_CURVE_WITH_KNOTS('',3,(#83483,#83484,#83485,#83486,#83487,
#83488,#83489,#83490,#83491,#83492,#83493,#83494,#83495,#83496,#83497,#83498,
#83499,#83500,#83501,#83502,#83503,#83504,#83505,#83506,#83507,#83508,#83509,
#83510,#83511,#83512,#83513,#83514,#83515,#83516,#83517,#83518,#83519,#83520,
#83521,#83522,#83523,#83524,#83525,#83526,#83527,#83528,#83529,#83530,#83531,
#83532,#83533,#83534,#83535,#83536,#83537,#83538,#83539,#83540,#83541,#83542,
#83543,#83544,#83545,#83546,#83547,#83548,#83549,#83550,#83551,#83552,#83553,
#83554,#83555,#83556,#83557,#83558,#83559,#83560,#83561,#83562,#83563,#83564,
#83565,#83566,#83567,#83568,#83569,#83570,#83571,#83572,#83573,#83574,#83575,
#83576,#83577,#83578,#83579,#83580,#83581,#83582,#83583,#83584,#83585,#83586,
#83587,#83588,#83589,#83590,#83591,#83592,#83593,#83594,#83595,#83596,#83597,
#83598,#83599,#83600,#83601,#83602,#83603,#83604,#83605,#83606,#83607,#83608,
#83609,#83610,#83611,#83612,#83613,#83614,#83615,#83616,#83617,#83618,#83619,
#83620,#83621,#83622,#83623,#83624,#83625,#83626,#83627,#83628,#83629,#83630,
#83631,#83632,#83633,#83634,#83635,#83636,#83637,#83638,#83639,#83640,#83641,
#83642,#83643,#83644,#83645,#83646,#83647,#83648,#83649,#83650,#83651,#83652,
#83653,#83654,#83655,#83656,#83657,#83658,#83659,#83660,#83661,#83662,#83663,
#83664,#83665,#83666),.UNSPECIFIED.,.F.,.F.,(4,3,3,3,3,3,3,3,3,3,3,3,3,
3,3,3,3,3,3,3,3,3,3,3,3,3,3,3,3,3,3,3,3,3,3,3,3,3,3,3,3,3,3,3,3,3,3,3,3,
3,3,3,3,3,3,3,3,3,3,3,3,4),(26.7961971418499,26.8083382968715,26.9074246897037,
27.0063712146189,27.1057297772008,27.2045008356489,27.3032397020132,27.4019761219099,
27.501792020251,27.6006696972515,27.7009547062628,27.8012397152742,27.9003266636363,
27.9992737513498,28.0986321741407,28.1974038087594,28.296143254997,28.3948802576534,
28.4946954766592,28.5935737374497,28.6938574355633,28.7941411336768,28.8932250348956,
28.9921690680764,29.0915282535767,29.1902968380783,29.2890332426283,29.3877672161178,
29.4875860501082,29.5864613431686,29.6867519476241,29.7870425520795,29.8861308341416,
29.9850792362496,30.0844373280286,30.1832102211334,30.2819509022162,30.3806891145515,
30.4805028285342,30.5793822255267,30.6796630980044,30.7799439704821,30.8790345145378,
30.977985232193,31.0773427517795,31.1761180722291,31.2748612169249,31.3736019255314,
31.4734127913698,31.5722947382858,31.6725700635853,31.7728453888848,31.8712868407757,
31.9695889139027,32.0677797276253,32.1659104762213,32.2640117568114,32.3621141291314,
32.4603109955813,32.558557434612,32.6569676584442,32.7254896765486),
 .UNSPECIFIED.);
#696=B_SPLINE_CURVE_WITH_KNOTS('',3,(#83667,#83668,#83669,#83670,#83671,
#83672,#83673,#83674,#83675,#83676,#83677,#83678,#83679,#83680,#83681,#83682),
 .UNSPECIFIED.,.F.,.F.,(4,3,3,3,3,4),(32.725489676875,32.7657468072874,
32.8648376513885,32.9638055933405,33.0626616366559,33.079934870469),
 .UNSPECIFIED.);
#697=B_SPLINE_CURVE_WITH_KNOTS('',3,(#83684,#83685,#83686,#83687,#83688,
#83689,#83690,#83691,#83692,#83693,#83694,#83695),.UNSPECIFIED.,.F.,.F.,
(4,2,2,2,2,4),(-0.0902464959671978,-0.0876094181756293,-0.0767074401332747,
-0.0648824535281501,-0.0438358835002987,-0.000729091238856221),
 .UNSPECIFIED.);
#698=B_SPLINE_CURVE_WITH_KNOTS('',3,(#83696,#83697,#83698,#83699,#83700,
#83701,#83702,#83703,#83704,#83705,#83706,#83707,#83708,#83709,#83710,#83711,
#83712,#83713,#83714,#83715,#83716,#83717,#83718,#83719,#83720,#83721,#83722,
#83723,#83724,#83725,#83726,#83727,#83728,#83729,#83730,#83731,#83732,#83733,
#83734,#83735,#83736,#83737,#83738,#83739,#83740,#83741,#83742,#83743,#83744,
#83745,#83746,#83747,#83748,#83749,#83750,#83751,#83752,#83753,#83754,#83755,
#83756,#83757,#83758,#83759,#83760,#83761,#83762,#83763,#83764,#83765,#83766,
#83767,#83768,#83769,#83770,#83771,#83772,#83773,#83774,#83775,#83776,#83777,
#83778,#83779,#83780,#83781,#83782,#83783,#83784,#83785,#83786,#83787,#83788,
#83789,#83790,#83791,#83792,#83793,#83794,#83795,#83796,#83797,#83798,#83799,
#83800,#83801,#83802,#83803,#83804,#83805,#83806,#83807,#83808,#83809,#83810,
#83811,#83812,#83813,#83814,#83815,#83816,#83817,#83818,#83819,#83820,#83821,
#83822,#83823,#83824,#83825,#83826,#83827,#83828,#83829,#83830,#83831,#83832,
#83833,#83834,#83835,#83836,#83837,#83838,#83839,#83840,#83841,#83842,#83843),
 .UNSPECIFIED.,.F.,.F.,(4,2,2,2,2,2,2,2,2,2,2,2,2,2,2,2,2,2,2,2,2,2,2,2,
2,2,2,2,2,2,2,2,2,2,2,2,2,2,2,2,2,2,2,2,2,2,2,2,2,2,2,2,2,2,2,2,2,2,2,2,
2,2,2,2,2,2,2,2,2,2,2,2,2,4),(-3.17275100264301,-3.14186154461218,-3.13391409134658,
-3.12678168783638,-3.12052738437692,-3.11046928271894,-3.0731019603304,
-3.03864936246736,-3.01554524537885,-3.00339627109982,-2.99258199427153,
-2.97803186410277,-2.92311059284616,-2.89904747261095,-2.88365703590017,
-2.87640159181438,-2.87019111156838,-2.86042990399181,-2.81692426495564,
-2.78589648558406,-2.76412306997584,-2.75217855489811,-2.74131031810344,
-2.72630553692097,-2.69124774359334,-2.65418066394503,-2.63464265155557,
-2.62680585721525,-2.62064554179685,-2.61185961982967,-2.58205337124216,
-2.54078613948644,-2.51542872926686,-2.50295632111094,-2.49219628449891,
-2.47845711696807,-2.41843773622056,-2.39648021659992,-2.38193940820278,
-2.37482226251611,-2.3685595639494,-2.35845362519604,-2.32212341401948,
-2.28705579500856,-2.26372576792335,-2.25154177326307,-2.24073318534329,
-2.22624767424738,-2.17077305608563,-2.14694101379957,-2.13163998576844,
-2.12439815366644,-2.11818188436821,-2.10838569704584,-2.06526937981979,
-2.01895781217817,-2.00479172184713,-1.99401417590832,-1.98165464286044,
-1.95711580672057,-1.94344505849879,-1.90317670897896,-1.88285251345712,
-1.8749212517719,-1.86876804610265,-1.86010430858303,-1.83300238482102,
-1.7958737414637,-1.7653517346366,-1.75225782536403,-1.74153208370379,-1.72833682184749,
-1.69978587912751,-1.67614713822004),.UNSPECIFIED.);
#699=B_SPLINE_CURVE_WITH_KNOTS('',3,(#83849,#83850,#83851,#83852,#83853,
#83854,#83855,#83856,#83857,#83858),.UNSPECIFIED.,.F.,.F.,(4,1,1,1,1,1,
1,4),(20.5123630354388,20.8509297864556,21.8438312048583,22.8367326232609,
23.8296340416636,24.8225354600662,25.8154368784689,26.4423043696954),
 .UNSPECIFIED.);
#700=B_SPLINE_CURVE_WITH_KNOTS('',3,(#83859,#83860,#83861,#83862,#83863,
#83864,#83865,#83866,#83867,#83868,#83869,#83870,#83871),.UNSPECIFIED.,
 .F.,.F.,(4,3,3,3,4),(26.4423043696954,26.5538023218569,26.665819695498,
26.778442329872,26.7961971418499),.UNSPECIFIED.);
#701=B_SPLINE_CURVE_WITH_KNOTS('',3,(#83872,#83873,#83874,#83875,#83876,
#83877,#83878,#83879,#83880,#83881,#83882,#83883,#83884,#83885,#83886,#83887,
#83888,#83889,#83890,#83891,#83892,#83893,#83894,#83895,#83896,#83897,#83898,
#83899,#83900,#83901,#83902,#83903,#83904,#83905,#83906,#83907,#83908,#83909,
#83910,#83911,#83912,#83913,#83914,#83915,#83916,#83917,#83918,#83919,#83920,
#83921,#83922,#83923,#83924,#83925,#83926,#83927,#83928,#83929,#83930,#83931,
#83932,#83933,#83934,#83935,#83936,#83937,#83938,#83939,#83940,#83941,#83942,
#83943,#83944,#83945,#83946,#83947,#83948,#83949,#83950,#83951,#83952,#83953,
#83954,#83955,#83956,#83957,#83958,#83959,#83960,#83961,#83962,#83963,#83964,
#83965,#83966,#83967,#83968,#83969,#83970,#83971,#83972,#83973,#83974,#83975,
#83976,#83977,#83978,#83979,#83980,#83981,#83982,#83983,#83984,#83985,#83986,
#83987,#83988,#83989,#83990,#83991,#83992,#83993,#83994,#83995,#83996,#83997,
#83998,#83999,#84000,#84001,#84002,#84003,#84004,#84005,#84006,#84007,#84008,
#84009,#84010,#84011,#84012,#84013,#84014,#84015,#84016,#84017,#84018,#84019,
#84020,#84021,#84022,#84023,#84024,#84025,#84026,#84027,#84028,#84029,#84030,
#84031),.UNSPECIFIED.,.F.,.F.,(4,2,2,2,2,2,2,2,2,2,2,2,2,2,2,2,2,2,2,2,
2,2,2,2,2,2,2,2,2,2,2,2,2,2,2,2,2,2,2,2,2,2,2,2,2,2,2,2,2,2,2,2,2,2,2,2,
2,2,2,2,2,2,2,2,2,2,2,2,2,2,2,2,2,2,2,2,2,2,2,4),(-1.67614713822004,-1.65401491148783,
-1.63251175695329,-1.62444928224132,-1.61830360713468,-1.60979944321575,
-1.58696249204113,-1.52960393139486,-1.50957186701517,-1.49790654268451,
-1.48692695737201,-1.47112058969116,-1.45223197297707,-1.40489495726156,
-1.38255085293624,-1.37499654555521,-1.36881635347511,-1.3611306407341,
-1.34278704356159,-1.31005547939534,-1.26959246473498,-1.25432849237837,
-1.24342545598734,-1.23157987920752,-1.2104338861163,-1.18090569021946,
-1.1342505763082,-1.1248144059171,-1.11858647777933,-1.1111452773009,-1.09454553617311,
-1.0672186360059,-1.01882421882921,-1.00360804187264,-0.99271197540947,
-0.980849747096349,-0.959596069961657,-0.929814359854932,-0.883722915131605,
-0.874227544364716,-0.867992282891039,-0.860581824198139,-0.844186378574769,
-0.817434397532054,-0.767999114531816,-0.752862232035203,-0.741977246487827,
-0.730085985061274,-0.708646138072557,-0.678422330470221,-0.633297614617569,
-0.623701010386046,-0.617452516392324,-0.61009212944287,-0.594025323639252,
-0.568177210783094,-0.517003661116067,-0.502025530146775,-0.491161609799766,
-0.479208204462634,-0.45737031425613,-0.426182182130144,-0.38306916999317,
-0.373281596103964,-0.367068071226507,-0.359826373340644,-0.344516644135123,
-0.32065728539347,-0.265219811356024,-0.250729590978973,-0.239923545802512,
-0.227748504194372,-0.204456692528434,-0.169482548134206,-0.133092781942825,
-0.122991718627395,-0.116731300983826,-0.109616022657332,-0.0950772289438299,
-0.0900798583104094),.UNSPECIFIED.);
#702=B_SPLINE_CURVE_WITH_KNOTS('',3,(#84037,#84038,#84039,#84040,#84041,
#84042,#84043,#84044,#84045,#84046,#84047,#84048,#84049,#84050,#84051,#84052,
#84053,#84054,#84055,#84056,#84057,#84058,#84059,#84060,#84061,#84062,#84063,
#84064,#84065,#84066,#84067,#84068,#84069,#84070,#84071,#84072,#84073,#84074,
#84075,#84076,#84077,#84078,#84079,#84080,#84081,#84082,#84083,#84084,#84085,
#84086,#84087,#84088,#84089,#84090,#84091,#84092,#84093,#84094,#84095,#84096,
#84097,#84098,#84099,#84100,#84101,#84102,#84103,#84104,#84105,#84106,#84107,
#84108,#84109,#84110,#84111,#84112,#84113,#84114,#84115,#84116,#84117,#84118,
#84119,#84120,#84121,#84122,#84123,#84124,#84125,#84126,#84127,#84128,#84129,
#84130,#84131,#84132,#84133,#84134,#84135,#84136,#84137,#84138,#84139,#84140,
#84141,#84142,#84143,#84144,#84145,#84146,#84147,#84148,#84149,#84150,#84151,
#84152,#84153,#84154,#84155,#84156,#84157,#84158,#84159,#84160,#84161,#84162,
#84163,#84164,#84165,#84166,#84167,#84168,#84169,#84170,#84171,#84172,#84173,
#84174,#84175,#84176,#84177,#84178,#84179,#84180,#84181,#84182,#84183,#84184,
#84185,#84186,#84187,#84188,#84189,#84190,#84191,#84192,#84193,#84194,#84195,
#84196,#84197,#84198,#84199,#84200,#84201,#84202,#84203,#84204,#84205,#84206,
#84207,#84208,#84209,#84210,#84211,#84212,#84213,#84214,#84215,#84216,#84217),
 .UNSPECIFIED.,.F.,.F.,(4,3,3,3,3,3,3,3,3,3,3,3,3,3,3,3,3,3,3,3,3,3,3,3,
3,3,3,3,3,3,3,3,3,3,3,3,3,3,3,3,3,3,3,3,3,3,3,3,3,3,3,3,3,3,3,3,3,3,3,3,
4),(14.2303478778739,14.329105063061,14.4278397994346,14.5265818258258,
14.6254258105938,14.7243233111684,14.8233894932032,14.8935212760397,14.9926074889702,
15.091553836683,15.1909124439029,15.2896833329404,15.3884220331809,15.487158290449,
15.5869743914473,15.6858519159895,15.7861373052159,15.8864226944424,15.9855088639308,
16.0844551671027,16.1838137853205,16.2825846274612,16.3813232800216,16.4800594888892,
16.5798756448781,16.6787531197307,16.7790386162878,16.879324112845,16.9784103341468,
17.0773566899656,17.1767152951259,17.2754861915545,17.3742248988989,17.4729611629723,
17.5727772550412,17.6716547855774,17.7719401584125,17.8722255312477,17.9713117348412,
18.0702580727662,18.1696166823767,18.2683875605948,18.3671262496506,18.4658624953827,
18.5656786089496,18.6645561212032,18.7648415354267,18.8651269496503,18.9642131523896,
19.0631594893563,19.1625180991934,19.2612889762052,19.3600276639639,19.4587639083096,
19.5585800232454,19.6574575339053,19.7577429509792,19.858028368053,19.9779659444179,
20.0964128676089,20.1591190625158),.UNSPECIFIED.);
#703=B_SPLINE_CURVE_WITH_KNOTS('',3,(#84218,#84219,#84220,#84221),
 .UNSPECIFIED.,.F.,.F.,(4,4),(20.1591190625158,20.5123630354388),
 .UNSPECIFIED.);
#704=B_SPLINE_CURVE_WITH_KNOTS('',3,(#84223,#84224,#84225,#84226,#84227,
#84228,#84229,#84230,#84231,#84232),.UNSPECIFIED.,.F.,.F.,(4,2,2,2,4),(-0.0900798583104094,
-0.0731194009899147,-0.0178332553777174,-0.0079637246705691,-0.000765186884287919),
 .UNSPECIFIED.);
#705=B_SPLINE_CURVE_WITH_KNOTS('',3,(#84233,#84234,#84235,#84236,#84237,
#84238,#84239,#84240,#84241,#84242),.UNSPECIFIED.,.F.,.F.,(4,1,1,1,1,1,
1,4),(-16.4153450200003,-15.8864226944424,-14.8935212760397,-13.9006198576371,
-12.9077184392344,-11.9148170208318,-10.9219156024291,-10.4858135521078),
 .UNSPECIFIED.);
#706=B_SPLINE_CURVE_WITH_KNOTS('',3,(#84248,#84249,#84250,#84251,#84252,
#84253,#84254,#84255,#84256,#84257,#84258,#84259,#84260),.UNSPECIFIED.,
 .F.,.F.,(4,3,3,3,4),(-4.20357440982612,-4.10477081863081,-4.00580716021436,
-3.9716056736106,-3.84897440564112),.UNSPECIFIED.);
#707=B_SPLINE_CURVE_WITH_KNOTS('',3,(#84262,#84263,#84264,#84265,#84266,
#84267,#84268,#84269,#84270,#84271,#84272,#84273,#84274,#84275,#84276,#84277,
#84278,#84279,#84280,#84281,#84282,#84283,#84284,#84285,#84286,#84287,#84288,
#84289,#84290,#84291,#84292,#84293,#84294,#84295,#84296,#84297,#84298,#84299,
#84300,#84301,#84302,#84303,#84304,#84305,#84306,#84307,#84308,#84309,#84310,
#84311,#84312,#84313,#84314,#84315,#84316,#84317,#84318,#84319,#84320,#84321,
#84322,#84323,#84324,#84325,#84326,#84327,#84328,#84329,#84330,#84331,#84332,
#84333,#84334,#84335,#84336,#84337,#84338,#84339,#84340,#84341,#84342,#84343,
#84344,#84345,#84346,#84347,#84348,#84349,#84350,#84351,#84352,#84353,#84354,
#84355,#84356,#84357,#84358,#84359,#84360,#84361,#84362,#84363,#84364,#84365,
#84366,#84367,#84368,#84369,#84370,#84371,#84372,#84373,#84374,#84375,#84376,
#84377,#84378,#84379),.UNSPECIFIED.,.F.,.F.,(4,3,3,3,3,3,3,3,3,3,3,3,3,
3,3,3,3,3,3,3,3,3,3,3,3,3,3,3,3,3,3,3,3,3,3,3,3,3,3,4),(-3.84897440539012,
-3.75118261568908,-3.65352307956186,-3.55593660581752,-3.45839196281045,
-3.36085797170509,-3.26323988314662,-3.16558158777684,-3.06775694336586,
-2.97870425520795,-2.87951096573215,-2.78045540351959,-2.6811238326803,
-2.58223942123546,-2.48338585298897,-2.38453355427412,-2.28485087490691,
-2.18585568108901,-2.08582925894716,-1.9858028368053,-1.88771322941384,
-1.78976397356157,-1.6901561541667,-1.59237691450442,-1.49462591498151,
-1.39687225137187,-1.29587954312957,-1.19796246900829,-1.09543194370547,
-0.992901418402649,-0.89112328419197,-0.789504516915043,-0.688044984898128,
-0.586679197074179,-0.485382845519511,-0.384131701056394,-0.282872156371267,
-0.181614269833575,-0.0802834070124286,0.),.UNSPECIFIED.);
#708=B_SPLINE_CURVE_WITH_KNOTS('',3,(#84383,#84384,#84385,#84386,#84387,
#84388,#84389,#84390,#84391,#84392,#84393,#84394,#84395,#84396,#84397,#84398,
#84399,#84400,#84401,#84402,#84403,#84404,#84405,#84406,#84407,#84408,#84409,
#84410,#84411,#84412,#84413,#84414,#84415,#84416,#84417,#84418,#84419,#84420,
#84421,#84422,#84423,#84424,#84425,#84426,#84427,#84428,#84429,#84430,#84431,
#84432,#84433,#84434,#84435,#84436,#84437,#84438,#84439,#84440,#84441,#84442,
#84443,#84444,#84445,#84446,#84447,#84448,#84449,#84450,#84451,#84452,#84453,
#84454,#84455,#84456,#84457,#84458,#84459,#84460,#84461,#84462,#84463,#84464,
#84465,#84466,#84467,#84468,#84469,#84470,#84471,#84472,#84473,#84474,#84475,
#84476,#84477,#84478,#84479,#84480,#84481,#84482,#84483,#84484,#84485,#84486,
#84487,#84488,#84489,#84490,#84491,#84492,#84493,#84494,#84495,#84496,#84497,
#84498,#84499,#84500,#84501,#84502,#84503,#84504,#84505,#84506,#84507,#84508,
#84509,#84510,#84511,#84512,#84513,#84514,#84515,#84516,#84517,#84518,#84519,
#84520,#84521,#84522,#84523,#84524,#84525,#84526,#84527,#84528,#84529,#84530,
#84531,#84532,#84533,#84534,#84535,#84536,#84537,#84538,#84539,#84540,#84541,
#84542,#84543,#84544,#84545,#84546,#84547,#84548,#84549,#84550,#84551,#84552,
#84553,#84554),.UNSPECIFIED.,.F.,.F.,(4,3,3,3,3,3,3,3,3,3,3,3,3,3,3,3,3,
3,3,3,3,3,3,3,3,3,3,3,3,3,3,3,3,3,3,3,3,3,3,3,3,3,3,3,3,3,3,3,3,3,3,3,3,
3,3,3,3,4),(2.01695736539979,2.11562565186726,2.21415522447183,2.3125739720312,
2.41093268850728,2.50926169686093,2.60759128292761,2.70601567817816,2.80448866800834,
2.90312821026225,2.97870425520795,3.07795262354351,3.1770644355191,3.27638209028053,
3.3753252578773,3.47423841070976,3.57315105478647,3.6727647094925,3.77182156828368,
3.87171362094714,3.9716056736106,4.07057405953448,4.16940092002274,4.26878919152156,
4.36743741751875,4.46605253078176,4.56466444154242,4.66462510416012,4.76337766491379,
4.86394237846352,4.96450709201325,5.06361683813577,5.1625868114871,5.2619395238532,
5.36073408273825,5.45949641510771,5.55825623360058,5.65804430280441,5.75694496937577,
5.85717673989584,5.9574085104159,6.05651255527721,6.15547712567804,6.25483122607061,
6.35362115696554,6.45237916506658,6.55113497045899,6.65092871004888,6.74982617701673,
6.85006805291764,6.95030992881855,7.04969433302994,7.14893807815273,7.24807060895532,
7.34712014750351,7.44612108226041,7.5451208045432,7.59274844815667),
 .UNSPECIFIED.);
#709=B_SPLINE_CURVE_WITH_KNOTS('',3,(#84555,#84556,#84557,#84558,#84559,
#84560,#84561,#84562,#84563,#84564,#84565,#84566,#84567),.UNSPECIFIED.,
 .F.,.F.,(4,3,3,3,4),(7.59274844852443,7.70563146856783,7.82442140789452,
7.9432113472212,7.94673289122112),.UNSPECIFIED.);
#710=B_SPLINE_CURVE_WITH_KNOTS('',3,(#84573,#84574,#84575,#84576,#84577,
#84578,#84579,#84580,#84581,#84582),.UNSPECIFIED.,.F.,.F.,(4,2,2,2,4),(-0.0892373222902252,
-0.0215572701752487,-0.00841522927678683,-0.00391774174210212,0.),
 .UNSPECIFIED.);
#711=B_SPLINE_CURVE_WITH_KNOTS('',3,(#84585,#84586,#84587,#84588,#84589,
#84590,#84591,#84592,#84593,#84594,#84595,#84596,#84597,#84598,#84599,#84600,
#84601,#84602,#84603,#84604,#84605,#84606,#84607,#84608,#84609,#84610,#84611,
#84612,#84613,#84614,#84615,#84616,#84617,#84618,#84619,#84620,#84621,#84622,
#84623,#84624,#84625,#84626,#84627,#84628,#84629,#84630,#84631,#84632,#84633,
#84634,#84635,#84636,#84637,#84638,#84639,#84640),.UNSPECIFIED.,.F.,.F.,
(4,2,2,2,2,2,2,2,2,2,2,2,2,2,2,2,2,2,2,2,2,2,2,2,2,2,2,4),(-2.19717915922714,
-2.19645659009491,-2.18931965603961,-2.15050379135875,-2.11839010273414,
-2.09607100903603,-2.08392470023533,-2.07289364098603,-2.05763555569738,
-2.01581763729026,-1.98568438600816,-1.96817169548238,-1.96050423950668,
-1.95417132940057,-1.94455971106179,-1.89929675230279,-1.86927758549977,
-1.84792623098591,-1.83601276060896,-1.82505977551714,-1.80973768729716,
-1.76181010825729,-1.73403052891512,-1.71725415524436,-1.70977854721702,
-1.70358054739824,-1.69426186068016,-1.67609529766553),.UNSPECIFIED.);
#712=B_SPLINE_CURVE_WITH_KNOTS('',3,(#84646,#84647,#84648,#84649,#84650,
#84651,#84652,#84653,#84654,#84655,#84656,#84657,#84658,#84659,#84660,#84661,
#84662,#84663,#84664,#84665,#84666,#84667,#84668,#84669,#84670,#84671,#84672,
#84673,#84674,#84675,#84676,#84677,#84678,#84679,#84680,#84681,#84682,#84683,
#84684,#84685,#84686,#84687,#84688,#84689,#84690,#84691,#84692,#84693,#84694,
#84695,#84696,#84697,#84698,#84699,#84700,#84701,#84702,#84703,#84704,#84705,
#84706,#84707,#84708,#84709,#84710,#84711,#84712,#84713,#84714,#84715,#84716,
#84717,#84718,#84719,#84720,#84721,#84722,#84723,#84724,#84725,#84726,#84727,
#84728,#84729,#84730,#84731,#84732,#84733,#84734,#84735,#84736,#84737,#84738,
#84739,#84740,#84741,#84742,#84743,#84744,#84745,#84746,#84747,#84748,#84749,
#84750,#84751,#84752,#84753,#84754,#84755,#84756,#84757,#84758,#84759,#84760,
#84761,#84762,#84763,#84764,#84765,#84766,#84767,#84768,#84769,#84770,#84771,
#84772,#84773,#84774,#84775,#84776,#84777,#84778,#84779,#84780,#84781,#84782,
#84783,#84784,#84785,#84786,#84787,#84788,#84789,#84790,#84791,#84792,#84793,
#84794,#84795,#84796,#84797,#84798,#84799,#84800,#84801,#84802,#84803,#84804,
#84805,#84806,#84807,#84808,#84809,#84810,#84811,#84812,#84813,#84814,#84815,
#84816,#84817,#84818,#84819,#84820,#84821,#84822,#84823,#84824,#84825,#84826),
 .UNSPECIFIED.,.F.,.F.,(4,3,3,3,3,3,3,3,3,3,3,3,3,3,3,3,3,3,3,3,3,3,3,3,
3,3,3,3,3,3,3,3,3,3,3,3,3,3,3,3,3,3,3,3,3,3,3,3,3,3,3,3,3,3,3,3,3,3,3,3,
4),(33.0799350929859,33.1787180525024,33.27747369025,33.3762317226554,33.4750883991966,
33.5739941598867,33.6730728822677,33.7586482256901,33.857757189267,33.9567265860696,
34.0560794683225,34.1548739552646,34.2536364053097,34.3523965307192,34.4521848090626,
34.5510862436967,34.6513179438947,34.7515496440927,34.8505112553917,34.9493327069361,
35.048722501381,35.1473686785809,35.2459830077185,35.3445953985981,35.4445593145724,
35.5433154579641,35.6438832602297,35.7444510624954,35.8437172783021,35.942843131204,
36.0421567999157,36.141104668409,36.2400190007244,36.3389293052607,36.43853509917,
36.537581025639,36.6374667532685,36.737352480898,36.8365465941635,36.9356029841046,
37.0349343485041,37.1338195908865,37.2326739893535,37.3315271163957,37.431208812122,
37.5302048209883,37.6302293601445,37.7302538993007,37.8283418314163,37.9262894071898,
38.025897646004,38.1236752026466,38.2214245205825,38.3191765055242,38.420171208569,
38.5180866257596,38.6206209717314,38.7231553177033,38.8550671088507,38.9837349211043,
39.0086643637188),.UNSPECIFIED.);
#713=B_SPLINE_CURVE_WITH_KNOTS('',3,(#84827,#84828,#84829,#84830,#84831,
#84832,#84833,#84834,#84835,#84836,#84837,#84838,#84839,#84840),
 .UNSPECIFIED.,.F.,.F.,(4,2,2,2,2,2,4),(-0.178881538265878,-0.14875089528117,
-0.131111218924469,-0.117656600924242,-0.105764816929103,-0.0895156630152576,
-0.0892373222902252),.UNSPECIFIED.);
#714=B_SPLINE_CURVE_WITH_KNOTS('',3,(#84841,#84842,#84843,#84844,#84845,
#84846,#84847,#84848,#84849,#84850,#84851,#84852,#84853,#84854,#84855,#84856,
#84857,#84858,#84859,#84860,#84861,#84862,#84863,#84864,#84865,#84866,#84867,
#84868,#84869,#84870,#84871,#84872,#84873,#84874,#84875,#84876,#84877,#84878,
#84879,#84880,#84881,#84882,#84883,#84884,#84885,#84886,#84887,#84888,#84889,
#84890,#84891,#84892,#84893,#84894,#84895,#84896,#84897,#84898,#84899,#84900,
#84901,#84902,#84903,#84904,#84905,#84906,#84907,#84908,#84909,#84910,#84911,
#84912,#84913,#84914,#84915,#84916,#84917,#84918,#84919,#84920,#84921,#84922,
#84923,#84924,#84925,#84926,#84927,#84928,#84929,#84930,#84931,#84932,#84933,
#84934,#84935,#84936,#84937,#84938,#84939,#84940,#84941,#84942,#84943,#84944,
#84945,#84946,#84947,#84948,#84949,#84950,#84951,#84952,#84953,#84954,#84955,
#84956,#84957,#84958,#84959,#84960,#84961,#84962,#84963,#84964,#84965,#84966,
#84967,#84968,#84969,#84970,#84971,#84972,#84973,#84974,#84975,#84976,#84977,
#84978,#84979,#84980,#84981,#84982,#84983,#84984,#84985,#84986,#84987,#84988,
#84989,#84990,#84991,#84992),.UNSPECIFIED.,.F.,.F.,(4,2,2,2,2,2,2,2,2,2,
2,2,2,2,2,2,2,2,2,2,2,2,2,2,2,2,2,2,2,2,2,2,2,2,2,2,2,2,2,2,2,2,2,2,2,2,
2,2,2,2,2,2,2,2,2,2,2,2,2,2,2,2,2,2,2,2,2,2,2,2,2,2,2,2,2,4),(-1.67609529766553,
-1.64671553914685,-1.61757900798281,-1.59663124306229,-1.58486995679092,
-1.57404350494896,-1.55890499236992,-1.50110180973233,-1.4795265849896,
-1.46515816266859,-1.45810063060918,-1.45184906365944,-1.44175954178262,
-1.41020899241748,-1.3719498655606,-1.35462917073466,-1.33973807254146,
-1.32886447655595,-1.31682811125898,-1.29455574748249,-1.24300901245012,
-1.22590455158308,-1.21355791334137,-1.20681516593851,-1.20020972960133,
-1.18854564067458,-1.13693985211147,-1.10104765354146,-1.08748853903,-1.07675187350426,
-1.0639741421333,-1.03626889690998,-0.985736232314045,-0.966465563951661,
-0.958541460300993,-0.952393138793696,-0.943736788111427,-0.914837267675602,
-0.852507151479367,-0.839533244827146,-0.828616662260341,-0.816853068039929,
-0.796161751914324,-0.767668513762618,-0.718696450045662,-0.709512462908799,
-0.703318801253057,-0.69574917775228,-0.678250055048964,-0.648246585598915,
-0.604153726816397,-0.588788941402707,-0.577872060287989,-0.566061952678386,
-0.545135101238413,-0.516106350454803,-0.468429108519963,-0.459108136308134,
-0.452894153556565,-0.445390943741233,-0.428358716657414,-0.39976905988297,
-0.353548207875082,-0.338224108628993,-0.327316247095225,-0.315499053855471,
-0.294510774400837,-0.265342670852866,-0.217920285619976,-0.20857071567736,
-0.202356004370044,-0.194875823355679,-0.177993703842297,-0.149843235549889,
-0.10290260483124,-0.0902465477143886),.UNSPECIFIED.);
#715=B_SPLINE_CURVE_WITH_KNOTS('',3,(#84998,#84999,#85000,#85001,#85002,
#85003,#85004,#85005,#85006,#85007,#85008,#85009,#85010,#85011,#85012,#85013,
#85014,#85015,#85016,#85017,#85018,#85019,#85020,#85021,#85022,#85023,#85024,
#85025,#85026,#85027,#85028,#85029,#85030,#85031,#85032,#85033,#85034,#85035,
#85036,#85037,#85038,#85039,#85040,#85041,#85042,#85043,#85044,#85045,#85046,
#85047,#85048,#85049,#85050,#85051,#85052,#85053,#85054,#85055,#85056,#85057,
#85058,#85059,#85060,#85061,#85062,#85063,#85064,#85065,#85066,#85067,#85068,
#85069,#85070,#85071,#85072,#85073,#85074,#85075,#85076,#85077,#85078,#85079,
#85080,#85081,#85082,#85083,#85084,#85085,#85086,#85087,#85088,#85089,#85090,
#85091,#85092,#85093,#85094,#85095,#85096,#85097,#85098,#85099,#85100,#85101,
#85102,#85103,#85104,#85105,#85106,#85107,#85108,#85109,#85110,#85111,#85112,
#85113,#85114,#85115,#85116,#85117,#85118,#85119,#85120,#85121,#85122,#85123,
#85124,#85125,#85126,#85127,#85128,#85129,#85130,#85131,#85132,#85133,#85134,
#85135,#85136,#85137,#85138,#85139,#85140,#85141,#85142,#85143,#85144,#85145,
#85146,#85147,#85148,#85149,#85150,#85151,#85152,#85153,#85154,#85155,#85156,
#85157,#85158,#85159,#85160,#85161,#85162,#85163,#85164,#85165,#85166,#85167,
#85168,#85169,#85170,#85171,#85172,#85173,#85174,#85175,#85176,#85177,#85178,
#85179,#85180,#85181),.UNSPECIFIED.,.F.,.F.,(4,3,3,3,3,3,3,3,3,3,3,3,3,
3,3,3,3,3,3,3,3,3,3,3,3,3,3,3,3,3,3,3,3,3,3,3,3,3,3,3,3,3,3,3,3,3,3,3,3,
3,3,3,3,3,3,3,3,3,3,3,3,4),(26.7961973726131,26.8083382968715,26.907424690282,
27.0063712157574,27.105729778197,27.2045008371582,27.3032397040171,27.4019761243891,
27.5017920221104,27.6006696995348,27.7009547074045,27.8012397152742,27.9003266702602,
27.9992737646337,28.0986321857641,28.1974038270813,28.296143280017,28.3948802893619,
28.4946955004406,28.5935737678283,28.6938574507526,28.7941411336768,28.8932250203573,
28.9921690389877,29.0915282281242,29.190296798151,29.2890331882864,29.3877671474404,
29.4875859986002,29.5864612776629,29.6867519148712,29.7870425520795,29.8861308403733,
29.9850792486213,30.0844373388539,30.1832102378347,30.2819509246824,30.3806891426645,
30.4805028496189,30.5793822519147,30.6796631111984,30.7799439704821,30.8790345488744,
30.9779853010793,31.077342812055,31.1761181673173,31.2748613468469,31.3736020902608,
31.4734129149168,31.5722948962214,31.6725701425531,31.7728453888848,31.8712867592265,
31.9695887507089,32.0677794829529,32.1659101501907,32.2640113496284,32.3621136410874,
32.4603104275931,32.5585567870616,32.6569669327387,32.7254896765487),
 .UNSPECIFIED.);
#716=B_SPLINE_CURVE_WITH_KNOTS('',3,(#85182,#85183,#85184,#85185,#85186,
#85187,#85188,#85189,#85190,#85191,#85192,#85193,#85194,#85195,#85196,#85197),
 .UNSPECIFIED.,.F.,.F.,(4,3,3,3,3,4),(32.725489676875,32.7657468072874,
32.8648376936571,32.9638056775635,33.062661762309,33.0799350929859),
 .UNSPECIFIED.);
#717=B_SPLINE_CURVE_WITH_KNOTS('',3,(#85199,#85200,#85201,#85202,#85203,
#85204,#85205,#85206,#85207,#85208,#85209,#85210),.UNSPECIFIED.,.F.,.F.,
(4,2,2,2,2,4),(-0.0902465477143886,-0.0876095400998589,-0.0767075193960174,
-0.0648825206908752,-0.0438360192347396,-0.000729083341957605),
 .UNSPECIFIED.);
#718=B_SPLINE_CURVE_WITH_KNOTS('',3,(#85211,#85212,#85213,#85214,#85215,
#85216,#85217,#85218,#85219,#85220,#85221,#85222,#85223,#85224,#85225,#85226,
#85227,#85228,#85229,#85230,#85231,#85232,#85233,#85234,#85235,#85236,#85237,
#85238,#85239,#85240,#85241,#85242,#85243,#85244,#85245,#85246,#85247,#85248,
#85249,#85250,#85251,#85252,#85253,#85254,#85255,#85256,#85257,#85258,#85259,
#85260,#85261,#85262,#85263,#85264,#85265,#85266,#85267,#85268,#85269,#85270,
#85271,#85272,#85273,#85274,#85275,#85276,#85277,#85278,#85279,#85280,#85281,
#85282,#85283,#85284,#85285,#85286,#85287,#85288,#85289,#85290,#85291,#85292,
#85293,#85294,#85295,#85296,#85297,#85298,#85299,#85300,#85301,#85302,#85303,
#85304,#85305,#85306,#85307,#85308,#85309,#85310,#85311,#85312,#85313,#85314,
#85315,#85316,#85317,#85318,#85319,#85320,#85321,#85322,#85323,#85324,#85325,
#85326,#85327,#85328,#85329,#85330,#85331,#85332,#85333,#85334,#85335,#85336,
#85337,#85338,#85339,#85340,#85341,#85342,#85343,#85344,#85345,#85346,#85347,
#85348,#85349,#85350,#85351,#85352,#85353,#85354,#85355,#85356,#85357,#85358,
#85359,#85360),.UNSPECIFIED.,.F.,.F.,(4,2,2,2,2,2,2,2,2,2,2,2,2,2,2,2,2,
2,2,2,2,2,2,2,2,2,2,2,2,2,2,2,2,2,2,2,2,2,2,2,2,2,2,2,2,2,2,2,2,2,2,2,2,
2,2,2,2,2,2,2,2,2,2,2,2,2,2,2,2,2,2,2,2,2,4),(-3.17269239421731,-3.1418080264104,
-3.13385954589945,-3.12672655156742,-3.12047280516759,-3.1104172371218,
-3.07299620890547,-3.03857721203288,-3.01548585115055,-3.00333909904038,
-2.99252480308098,-2.9779715427723,-2.92308193523701,-2.89900662609222,
-2.88361165360702,-2.87635565952824,-2.87014566122291,-2.86038664063358,
-2.81686173958364,-2.7858454430596,-2.76407706049396,-2.75213363579342,
-2.74126556810184,-2.72625965209991,-2.69116856650147,-2.65413166490487,
-2.63460179508923,-2.62676618807796,-2.6206059931027,-2.61181910365338,
-2.58193611504223,-2.54072680564311,-2.51538698177176,-2.50291729143309,
-2.49215734816347,-2.47841522688553,-2.41842410715263,-2.39645719873271,
-2.3819126630231,-2.37479506001559,-2.36853287548749,-2.35842916883865,
-2.32452674348858,-2.2878831010503,-2.26399844770101,-2.25173309026112,
-2.24094080149394,-2.22686244955933,-2.16941165174081,-2.14641839599599,
-2.13145176960661,-2.12426403664912,-2.11802875825167,-2.10810294433784,
-2.06796256488764,-2.03507111840387,-2.01894162719182,-2.00478194164045,
-1.99400494516425,-1.98164158191672,-1.95707581947592,-1.94344851811339,
-1.90317769083255,-1.88285290838813,-1.87492156667475,-1.86876834808487,
-1.86010465337482,-1.83300344367185,-1.7958742160871,-1.76535200430175,
-1.75225805290813,-1.74153228251082,-1.72833698796303,-1.69978753189247,
-1.67614738790005),.UNSPECIFIED.);
#719=B_SPLINE_CURVE_WITH_KNOTS('',3,(#85366,#85367,#85368,#85369,#85370,
#85371,#85372,#85373,#85374,#85375),.UNSPECIFIED.,.F.,.F.,(4,1,1,1,1,1,
1,4),(20.5123632666524,20.8509297864556,21.8438312048583,22.8367326232609,
23.8296340416636,24.8225354600662,25.8154368784689,26.4423043696954),
 .UNSPECIFIED.);
#720=B_SPLINE_CURVE_WITH_KNOTS('',3,(#85376,#85377,#85378,#85379,#85380,
#85381,#85382,#85383,#85384,#85385,#85386,#85387,#85388),.UNSPECIFIED.,
 .F.,.F.,(4,3,3,3,4),(26.4423043696954,26.5538023203891,26.6658196926276,
26.778442326011,26.7961973726131),.UNSPECIFIED.);
#721=B_SPLINE_CURVE_WITH_KNOTS('',3,(#85389,#85390,#85391,#85392,#85393,
#85394,#85395,#85396,#85397,#85398,#85399,#85400,#85401,#85402,#85403,#85404,
#85405,#85406,#85407,#85408,#85409,#85410,#85411,#85412,#85413,#85414,#85415,
#85416,#85417,#85418,#85419,#85420,#85421,#85422,#85423,#85424,#85425,#85426,
#85427,#85428,#85429,#85430,#85431,#85432,#85433,#85434,#85435,#85436,#85437,
#85438,#85439,#85440,#85441,#85442,#85443,#85444,#85445,#85446,#85447,#85448,
#85449,#85450,#85451,#85452,#85453,#85454,#85455,#85456,#85457,#85458,#85459,
#85460,#85461,#85462,#85463,#85464,#85465,#85466,#85467,#85468,#85469,#85470,
#85471,#85472,#85473,#85474,#85475,#85476,#85477,#85478,#85479,#85480,#85481,
#85482,#85483,#85484,#85485,#85486,#85487,#85488,#85489,#85490,#85491,#85492,
#85493,#85494,#85495,#85496,#85497,#85498,#85499,#85500,#85501,#85502,#85503,
#85504,#85505,#85506,#85507,#85508,#85509,#85510,#85511,#85512,#85513,#85514,
#85515,#85516,#85517,#85518,#85519,#85520,#85521,#85522,#85523,#85524,#85525,
#85526,#85527,#85528,#85529,#85530,#85531,#85532,#85533,#85534,#85535,#85536,
#85537,#85538,#85539,#85540,#85541,#85542,#85543,#85544,#85545,#85546,#85547,
#85548),.UNSPECIFIED.,.F.,.F.,(4,2,2,2,2,2,2,2,2,2,2,2,2,2,2,2,2,2,2,2,
2,2,2,2,2,2,2,2,2,2,2,2,2,2,2,2,2,2,2,2,2,2,2,2,2,2,2,2,2,2,2,2,2,2,2,2,
2,2,2,2,2,2,2,2,2,2,2,2,2,2,2,2,2,2,2,2,2,2,2,4),(-1.67614738790005,-1.65401539803214,
-1.63251200410341,-1.6244494917157,-1.61830380027013,-1.60979962397045,
-1.58696266804934,-1.52960415803192,-1.50957204956521,-1.49790669752566,
-1.48692708081092,-1.47112065152718,-1.45223194399327,-1.40489440322899,
-1.38255080966505,-1.37499656378177,-1.36881636593124,-1.36113055468062,
-1.34278630121307,-1.31005254648512,-1.26959232320727,-1.25432845224904,
-1.24342540625013,-1.23157974231834,-1.21043333302154,-1.1809041913237,
-1.13425114923896,-1.12481474505895,-1.11858677379479,-1.11114565468571,
-1.0945465402581,-1.06722144679975,-1.0188238102491,-1.00360783327805,-0.992711770276206,
-0.980849417064562,-0.959595084991448,-0.929811860271617,-0.883723717419915,
-0.874227982324294,-0.867992659951299,-0.860582344874721,-0.844187932972367,
-0.817438862528606,-0.767998151644771,-0.752861690727202,-0.741976737251043,
-0.730085262520449,-0.70864419881481,-0.678417516809986,-0.633298972396409,
-0.623701712095381,-0.617453115407401,-0.610093002657982,-0.594028063783899,
-0.568185038995766,-0.517001317180073,-0.502024174319338,-0.491160355365596,
-0.479206491575932,-0.457365804191386,-0.426170830491055,-0.383071357672949,
-0.373282689208771,-0.367068994072127,-0.359827730726221,-0.344520787293964,
-0.320668537576263,-0.265214737806784,-0.250726549549183,-0.239920698609147,
-0.227744574156621,-0.204445619843977,-0.169451754272856,-0.133092188794971,
-0.122991416082315,-0.116731032841127,-0.109615614144809,-0.0950760407469734,
-0.0900799055529525),.UNSPECIFIED.);
#722=B_SPLINE_CURVE_WITH_KNOTS('',3,(#85554,#85555,#85556,#85557,#85558,
#85559,#85560,#85561,#85562,#85563,#85564,#85565,#85566,#85567,#85568,#85569,
#85570,#85571,#85572,#85573,#85574,#85575,#85576,#85577,#85578,#85579,#85580,
#85581,#85582,#85583,#85584,#85585,#85586,#85587,#85588,#85589,#85590,#85591,
#85592,#85593,#85594,#85595,#85596,#85597,#85598,#85599,#85600,#85601,#85602,
#85603,#85604,#85605,#85606,#85607,#85608,#85609,#85610,#85611,#85612,#85613,
#85614,#85615,#85616,#85617,#85618,#85619,#85620,#85621,#85622,#85623,#85624,
#85625,#85626,#85627,#85628,#85629,#85630,#85631,#85632,#85633,#85634,#85635,
#85636,#85637,#85638,#85639,#85640,#85641,#85642,#85643,#85644,#85645,#85646,
#85647,#85648,#85649,#85650,#85651,#85652,#85653,#85654,#85655,#85656,#85657,
#85658,#85659,#85660,#85661,#85662,#85663,#85664,#85665,#85666,#85667,#85668,
#85669,#85670,#85671,#85672,#85673,#85674,#85675,#85676,#85677,#85678,#85679,
#85680,#85681,#85682,#85683,#85684,#85685,#85686,#85687,#85688,#85689,#85690,
#85691,#85692,#85693,#85694,#85695,#85696,#85697,#85698,#85699,#85700,#85701,
#85702,#85703,#85704,#85705,#85706,#85707,#85708,#85709,#85710,#85711,#85712,
#85713,#85714,#85715,#85716,#85717,#85718,#85719,#85720,#85721,#85722,#85723,
#85724,#85725,#85726,#85727,#85728,#85729,#85730,#85731,#85732,#85733,#85734),
 .UNSPECIFIED.,.F.,.F.,(4,3,3,3,3,3,3,3,3,3,3,3,3,3,3,3,3,3,3,3,3,3,3,3,
3,3,3,3,3,3,3,3,3,3,3,3,3,3,3,3,3,3,3,3,3,3,3,3,3,3,3,3,3,3,3,3,3,3,3,3,
4),(14.2303481072454,14.3291052935583,14.4278400311323,14.5265820587969,
14.6254260448789,14.7243235468301,14.8233897301623,14.8935212760397,14.992607488937,
15.0915538366193,15.1909124438472,15.2896833328613,15.3884220330811,15.4871582903312,
15.586974391359,15.6858519158902,15.7861373051663,15.8864226944424,15.9855088636077,
16.0844551664509,16.1838137847501,16.2825846265504,16.3813232787667,16.4800594872869,
16.5798756436764,16.6787531181774,16.7790386155112,16.879324112845,16.9784103343415,
17.0773566903575,17.1767152954688,17.2754861920995,17.3742248996474,17.4729611639253,
17.5727772557559,17.6716547864972,17.7719401588725,17.8722255312477,17.9713117348143,
18.0702580727126,18.1696166823298,18.2683875605216,18.3671262495515,18.465862495258,
18.565678608856,18.6645561210849,18.7648415353676,18.8651269496503,18.964213152378,
19.0631594893323,19.1625180991724,19.2612889761701,19.360027663914,19.4587639082443,
19.5585800231964,19.6574575338396,19.7577429509463,19.858028368053,19.9779659443332,
20.0964128674536,20.1591190625159),.UNSPECIFIED.);
#723=B_SPLINE_CURVE_WITH_KNOTS('',3,(#85735,#85736,#85737,#85738),
 .UNSPECIFIED.,.F.,.F.,(4,4),(20.1591190625159,20.5123632666524),
 .UNSPECIFIED.);
#724=B_SPLINE_CURVE_WITH_KNOTS('',3,(#85740,#85741,#85742,#85743,#85744,
#85745,#85746,#85747,#85748,#85749),.UNSPECIFIED.,.F.,.F.,(4,2,2,2,4),(-0.0900799055529525,
-0.0731163611940172,-0.0178336702430842,-0.00796388538298541,-0.00076518352726976),
 .UNSPECIFIED.);
#725=B_SPLINE_CURVE_WITH_KNOTS('',3,(#85750,#85751,#85752,#85753,#85754,
#85755,#85756,#85757,#85758,#85759),.UNSPECIFIED.,.F.,.F.,(4,1,1,1,1,1,
1,4),(-16.4153450200003,-15.8864226944424,-14.8935212760397,-13.9006198576371,
-12.9077184392344,-11.9148170208318,-10.9219156024291,-10.4858137779553),
 .UNSPECIFIED.);
#726=B_SPLINE_CURVE_WITH_KNOTS('',3,(#85765,#85766,#85767,#85768,#85769,
#85770,#85771,#85772,#85773,#85774,#85775,#85776,#85777),.UNSPECIFIED.,
 .F.,.F.,(4,3,3,3,4),(-4.20357446602247,-4.10477053931125,-4.00580655102466,
-3.9716056736106,-3.84897440564113),.UNSPECIFIED.);
#727=B_SPLINE_CURVE_WITH_KNOTS('',3,(#85779,#85780,#85781,#85782,#85783,
#85784,#85785,#85786,#85787,#85788,#85789,#85790,#85791,#85792,#85793,#85794,
#85795,#85796,#85797,#85798,#85799,#85800,#85801,#85802,#85803,#85804,#85805,
#85806,#85807,#85808,#85809,#85810,#85811,#85812,#85813,#85814,#85815,#85816,
#85817,#85818,#85819,#85820,#85821,#85822,#85823,#85824,#85825,#85826,#85827,
#85828,#85829,#85830,#85831,#85832,#85833,#85834,#85835,#85836,#85837,#85838,
#85839,#85840,#85841,#85842,#85843,#85844,#85845,#85846,#85847,#85848,#85849,
#85850,#85851,#85852,#85853,#85854,#85855,#85856,#85857,#85858,#85859,#85860,
#85861,#85862,#85863,#85864,#85865,#85866,#85867,#85868,#85869,#85870,#85871,
#85872,#85873,#85874,#85875,#85876,#85877,#85878,#85879,#85880,#85881,#85882,
#85883,#85884,#85885,#85886,#85887,#85888,#85889,#85890,#85891,#85892,#85893,
#85894,#85895,#85896),.UNSPECIFIED.,.F.,.F.,(4,3,3,3,3,3,3,3,3,3,3,3,3,
3,3,3,3,3,3,3,3,3,3,3,3,3,3,3,3,3,3,3,3,3,3,3,3,3,3,4),(-3.8489744053901,
-3.75118264277131,-3.65352312873579,-3.55593667405005,-3.45839204708363,
-3.36085806901283,-3.26323998878766,-3.16558169918367,-3.06775705625276,
-2.97870425520795,-2.87951180797405,-2.78045709200363,-2.68112531010384,
-2.58224174811673,-2.48338902857077,-2.38453757659689,-2.284853891649,-2.18585953093757,
-2.08583118387143,-1.9858028368053,-1.88771151482969,-1.78976053950896,
-1.69015314937067,-1.59237218731071,-1.49461946688772,-1.39686408539742,
-1.29587341864873,-1.19795464897449,-1.09542803368857,-0.992901418402651,
-0.891124553118223,-0.789507061012913,-0.68804880427994,-0.58668428904758,
-0.485389203973641,-0.384139316452674,-0.282881003294853,-0.181624333840912,
-0.0802946514713979,0.),.UNSPECIFIED.);
#728=B_SPLINE_CURVE_WITH_KNOTS('',3,(#85900,#85901,#85902,#85903,#85904,
#85905,#85906,#85907,#85908,#85909,#85910,#85911,#85912,#85913,#85914,#85915,
#85916,#85917,#85918,#85919,#85920,#85921,#85922,#85923,#85924,#85925,#85926,
#85927,#85928,#85929,#85930,#85931,#85932,#85933,#85934,#85935,#85936,#85937,
#85938,#85939,#85940,#85941,#85942,#85943,#85944,#85945,#85946,#85947,#85948,
#85949,#85950,#85951,#85952,#85953,#85954,#85955,#85956,#85957,#85958,#85959,
#85960,#85961,#85962,#85963,#85964,#85965,#85966,#85967,#85968,#85969,#85970,
#85971,#85972,#85973,#85974,#85975,#85976,#85977,#85978,#85979,#85980,#85981,
#85982,#85983,#85984,#85985,#85986,#85987,#85988,#85989,#85990,#85991,#85992,
#85993,#85994,#85995,#85996,#85997,#85998,#85999,#86000,#86001,#86002,#86003,
#86004,#86005,#86006,#86007,#86008,#86009,#86010,#86011,#86012,#86013,#86014,
#86015,#86016,#86017,#86018,#86019,#86020,#86021,#86022,#86023,#86024,#86025,
#86026,#86027,#86028,#86029,#86030,#86031,#86032,#86033,#86034,#86035,#86036,
#86037,#86038,#86039,#86040,#86041,#86042,#86043,#86044,#86045,#86046,#86047,
#86048,#86049,#86050,#86051,#86052,#86053,#86054,#86055,#86056,#86057,#86058,
#86059,#86060,#86061,#86062,#86063,#86064,#86065,#86066,#86067,#86068,#86069,
#86070,#86071),.UNSPECIFIED.,.F.,.F.,(4,3,3,3,3,3,3,3,3,3,3,3,3,3,3,3,3,
3,3,3,3,3,3,3,3,3,3,3,3,3,3,3,3,3,3,3,3,3,3,3,3,3,3,3,3,3,3,3,3,3,3,3,3,
3,3,3,3,4),(2.01695735912304,2.11562654140827,2.21415701847924,2.31257667970888,
2.41093631520768,2.50926624683899,2.60759675934576,2.70602208019458,2.80449599663101,
2.90313645744952,2.97870425520795,3.07795276095063,3.17706471441973,3.27638233431859,
3.37532565237687,3.47423895872607,3.57315175917927,3.6727652377871,3.77182225845132,
3.87171396603096,3.9716056736106,4.07057367524206,4.16940014596475,4.26878851422081,
4.36743633982893,4.46605104956199,4.56466255416582,4.66462368862768,4.76337584074457,
4.86394146637891,4.96450709201324,5.06361700642839,5.16258714977056,5.26193981985123,
5.36073455159112,5.45949705750217,5.55825704998521,5.65804491509288,5.75694575497821,
5.85717713269705,5.95740851041589,6.05651259099809,6.15547719813649,6.25483128947175,
6.35362125932815,6.45237930714439,6.55113515295565,6.65092884692138,6.749826355645,
6.85006814223177,6.95030992881854,7.04969426096498,7.14893793290924,7.24807038953629,
7.34711985275463,7.44612071151953,7.5451203572188,7.59274844815668),
 .UNSPECIFIED.);
#729=B_SPLINE_CURVE_WITH_KNOTS('',3,(#86072,#86073,#86074,#86075,#86076,
#86077,#86078,#86079,#86080,#86081,#86082,#86083,#86084),.UNSPECIFIED.,
 .F.,.F.,(4,3,3,3,4),(7.59274844852451,7.70563133194379,7.82442133958249,
7.94321134722119,7.94673310592174),.UNSPECIFIED.);
#730=B_SPLINE_CURVE_WITH_KNOTS('',3,(#86087,#86088,#86089,#86090,#86091,
#86092,#86093,#86094,#86095,#86096,#86097,#86098,#86099,#86100,#86101,#86102,
#86103,#86104,#86105,#86106,#86107,#86108,#86109,#86110,#86111,#86112,#86113,
#86114,#86115,#86116,#86117,#86118,#86119,#86120,#86121,#86122,#86123,#86124,
#86125,#86126,#86127,#86128,#86129,#86130,#86131,#86132,#86133,#86134,#86135,
#86136,#86137,#86138,#86139,#86140,#86141,#86142,#86143,#86144,#86145,#86146,
#86147,#86148,#86149,#86150,#86151,#86152,#86153,#86154,#86155,#86156,#86157,
#86158,#86159,#86160,#86161,#86162,#86163,#86164,#86165,#86166,#86167,#86168,
#86169,#86170,#86171,#86172,#86173,#86174,#86175,#86176,#86177,#86178,#86179,
#86180,#86181,#86182,#86183,#86184,#86185,#86186,#86187,#86188,#86189,#86190,
#86191,#86192,#86193,#86194,#86195,#86196,#86197,#86198,#86199,#86200,#86201,
#86202,#86203,#86204,#86205,#86206,#86207,#86208,#86209,#86210,#86211,#86212,
#86213,#86214,#86215,#86216,#86217,#86218,#86219,#86220,#86221,#86222,#86223,
#86224,#86225,#86226,#86227,#86228,#86229,#86230,#86231,#86232,#86233,#86234,
#86235,#86236,#86237,#86238,#86239,#86240,#86241,#86242,#86243,#86244,#86245,
#86246,#86247,#86248,#86249,#86250,#86251,#86252,#86253,#86254,#86255,#86256,
#86257,#86258,#86259,#86260,#86261,#86262,#86263,#86264,#86265,#86266,#86267),
 .UNSPECIFIED.,.F.,.F.,(4,3,3,3,3,3,3,3,3,3,3,3,3,3,3,3,3,3,3,3,3,3,3,3,
3,3,3,3,3,3,3,3,3,3,3,3,3,3,3,3,3,3,3,3,3,3,3,3,3,3,3,3,3,3,3,3,3,3,3,3,
4),(7.94673310592174,8.04581817646567,8.14476459328382,8.24368311482633,
8.34245702765183,8.44119968485212,8.53994082527461,8.63898381036192,8.73786714282491,
8.83698995422438,8.93611276562384,9.03520077646614,9.1341489668641,9.2335071190094,
9.33227994653866,9.43102061705201,9.52975887377632,9.62957270133887,9.728452277143,
9.82873323058475,9.92901418402649,10.0280982190887,10.127042354227,10.2264015102523,
10.3251701184937,10.4239065173681,10.5226404558074,10.6224592424628,10.7213344287368,
10.8216250155829,10.9219156024291,11.0210025472156,11.1199496335807,11.2193080569871,
11.3180796956776,11.4168191480129,11.515556158782,11.6153713742944,11.7142496480606,
11.8145333344462,11.9148170208318,12.0139033809216,12.112849880234,12.2122084501091,
12.310979500489,12.4097183653858,12.5084547904101,12.6082707026162,12.7071484008778,
12.8074334200561,12.9077184392344,13.006397200346,13.1049363913014,13.2033637313469,
13.3017302940464,13.4000663981463,13.498402324608,13.5968336628894,13.6953128615516,
13.7939621905588,13.8759337551205),.UNSPECIFIED.);
#731=B_SPLINE_CURVE_WITH_KNOTS('',3,(#86268,#86269,#86270,#86271,#86272,
#86273,#86274,#86275,#86276,#86277,#86278,#86279,#86280,#86281,#86282,#86283),
 .UNSPECIFIED.,.F.,.F.,(4,3,3,3,3,4),(13.8759337553363,13.9006198576371,
13.9996876770314,14.0986328228261,14.1974668341838,14.2303481072454),
 .UNSPECIFIED.);
#732=B_SPLINE_CURVE_WITH_KNOTS('',3,(#86285,#86286,#86287,#86288),
 .UNSPECIFIED.,.F.,.F.,(4,4),(-10.4858137779553,-10.132162382237),
 .UNSPECIFIED.);
#733=B_SPLINE_CURVE_WITH_KNOTS('',3,(#86289,#86290,#86291,#86292,#86293,
#86294,#86295,#86296,#86297,#86298,#86299,#86300,#86301,#86302,#86303,#86304,
#86305,#86306,#86307,#86308,#86309,#86310,#86311,#86312,#86313,#86314,#86315,
#86316,#86317,#86318,#86319,#86320,#86321,#86322,#86323,#86324,#86325,#86326,
#86327,#86328,#86329,#86330,#86331,#86332,#86333,#86334,#86335,#86336,#86337,
#86338,#86339,#86340,#86341,#86342,#86343,#86344,#86345,#86346,#86347,#86348,
#86349,#86350,#86351,#86352,#86353,#86354,#86355,#86356,#86357,#86358,#86359,
#86360,#86361,#86362,#86363,#86364,#86365,#86366,#86367,#86368,#86369,#86370,
#86371,#86372,#86373,#86374,#86375,#86376,#86377,#86378,#86379,#86380,#86381,
#86382,#86383,#86384,#86385,#86386,#86387,#86388,#86389,#86390,#86391,#86392,
#86393,#86394,#86395,#86396,#86397,#86398,#86399,#86400,#86401,#86402,#86403,
#86404,#86405,#86406,#86407,#86408,#86409,#86410,#86411,#86412,#86413,#86414,
#86415,#86416,#86417,#86418,#86419,#86420,#86421,#86422,#86423,#86424,#86425,
#86426,#86427,#86428,#86429,#86430,#86431,#86432,#86433,#86434,#86435,#86436,
#86437,#86438,#86439,#86440,#86441,#86442,#86443,#86444,#86445,#86446,#86447,
#86448,#86449,#86450,#86451,#86452,#86453,#86454,#86455,#86456,#86457,#86458,
#86459,#86460,#86461,#86462,#86463,#86464,#86465,#86466,#86467,#86468,#86469),
 .UNSPECIFIED.,.F.,.F.,(4,3,3,3,3,3,3,3,3,3,3,3,3,3,3,3,3,3,3,3,3,3,3,3,
3,3,3,3,3,3,3,3,3,3,3,3,3,3,3,3,3,3,3,3,3,3,3,3,3,3,3,3,3,3,3,3,3,3,3,3,
4),(-10.1321597128207,-9.99259860333552,-9.9290141840265,-9.82992590631703,
-9.73097750849788,-9.63161941563862,-9.53284652663874,-9.43410584958342,
-9.3353676411932,-9.23555392230086,-9.13667452901384,-9.03639364731884,
-8.93611276562384,-8.83702224548506,-8.73807155189518,-8.63871402631093,
-8.53993873010981,-8.4411956096771,-8.34245492531528,-8.24264403079176,
-8.14376210782866,-8.04348672752493,-7.9432113472212,-7.84414223683077,
-7.74521302140415,-7.64585013483095,-7.54709632547949,-7.44837464743071,
-7.34965533209489,-7.2498189812758,-7.15095803039816,-7.05063397960835,
-6.95030992881855,-6.85120368873458,-6.75223740083337,-6.65288378953119,
-6.55409331422877,-6.45533520337683,-6.35657973652944,-6.25678693000106,
-6.15789088086669,-6.05764969564129,-5.95740851041589,-5.85829983722156,
-5.75933073268631,-5.65997777760218,-5.56118358533646,-5.46242143021034,
-5.36366159955868,-5.26387297267232,-5.16497182938891,-5.06473946070108,
-4.96450709201325,-4.86557200000987,-4.76676516593899,-4.66805645652568,
-4.56941584216026,-4.47078819908846,-4.37217137319955,-4.2734867160408,
-4.20357446602247),.UNSPECIFIED.);
#734=B_SPLINE_CURVE_WITH_KNOTS('',3,(#86472,#86473,#86474,#86475,#86476,
#86477,#86478,#86479,#86480,#86481,#86482,#86483,#86484,#86485,#86486,#86487,
#86488,#86489,#86490,#86491,#86492,#86493,#86494,#86495,#86496,#86497,#86498,
#86499,#86500,#86501,#86502,#86503,#86504,#86505,#86506,#86507,#86508,#86509,
#86510,#86511,#86512,#86513,#86514,#86515,#86516,#86517,#86518,#86519,#86520,
#86521,#86522,#86523,#86524,#86525,#86526,#86527,#86528,#86529,#86530,#86531,
#86532,#86533,#86534,#86535,#86536,#86537,#86538,#86539,#86540,#86541,#86542,
#86543,#86544,#86545,#86546,#86547,#86548,#86549,#86550,#86551,#86552,#86553,
#86554,#86555,#86556,#86557,#86558,#86559,#86560,#86561,#86562,#86563,#86564,
#86565,#86566,#86567,#86568,#86569,#86570,#86571,#86572,#86573,#86574,#86575,
#86576,#86577,#86578,#86579,#86580,#86581,#86582,#86583,#86584,#86585,#86586,
#86587,#86588,#86589,#86590,#86591,#86592,#86593,#86594,#86595,#86596,#86597,
#86598,#86599,#86600,#86601,#86602,#86603,#86604,#86605,#86606,#86607,#86608,
#86609,#86610,#86611,#86612,#86613,#86614,#86615,#86616,#86617,#86618,#86619,
#86620,#86621,#86622,#86623,#86624,#86625,#86626,#86627,#86628,#86629,#86630,
#86631,#86632,#86633,#86634,#86635,#86636,#86637,#86638,#86639,#86640,#86641,
#86642,#86643,#86644,#86645,#86646,#86647,#86648,#86649,#86650,#86651,#86652),
 .UNSPECIFIED.,.F.,.F.,(4,3,3,3,3,3,3,3,3,3,3,3,3,3,3,3,3,3,3,3,3,3,3,3,
3,3,3,3,3,3,3,3,3,3,3,3,3,3,3,3,3,3,3,3,3,3,3,3,3,3,3,3,3,3,3,3,3,3,3,3,
4),(7.94673289122112,8.04581792837314,8.14476431138301,8.24368286816311,
8.34245674641829,8.44119936884877,8.53994047434931,8.63898354716794,8.73786684476973,
8.83698980519679,8.93611276562385,9.03520077148316,9.13414895672167,9.23350711013477,
9.33227993210958,9.43102059693156,9.52975884783475,9.62957268188268,9.72845225160275,
9.82873321781462,9.92901418402649,10.0280982326817,10.1270423816281,10.2264015342282,
10.325170156701,10.4239065699343,10.5226405228411,10.6224592927381,10.7213344936009,
10.821625048015,10.9219156024291,11.0210025407565,11.1199496205909,11.219308045621,
11.3180796776554,11.4168191233022,11.5155561273596,11.6153713507277,11.7142496177934,
11.8145333193126,11.9148170208318,12.0139033805419,12.1128498794499,12.212208449423,
12.3109794993409,12.4097183637549,12.5084547882763,12.6082707010158,12.7071483987294,
12.8074334189819,12.9077184392344,13.0063972024842,13.1049363956126,13.2033637378739,
13.301730302815,13.4000664091795,13.4984023379264,13.5968336785102,13.6953128794884,
13.7939622108089,13.8759337551205),.UNSPECIFIED.);
#735=B_SPLINE_CURVE_WITH_KNOTS('',3,(#86653,#86654,#86655,#86656,#86657,
#86658,#86659,#86660,#86661,#86662,#86663,#86664,#86665,#86666,#86667,#86668),
 .UNSPECIFIED.,.F.,.F.,(4,3,3,3,3,4),(13.8759337553363,13.9006198576371,
13.9996876759034,14.0986328205549,14.1974668307429,14.2303478778739),
 .UNSPECIFIED.);
#736=B_SPLINE_CURVE_WITH_KNOTS('',3,(#86670,#86671,#86672,#86673),
 .UNSPECIFIED.,.F.,.F.,(4,4),(-10.4858135521078,-10.1321623805438),
 .UNSPECIFIED.);
#737=B_SPLINE_CURVE_WITH_KNOTS('',3,(#86674,#86675,#86676,#86677,#86678,
#86679,#86680,#86681,#86682,#86683,#86684,#86685,#86686,#86687,#86688,#86689,
#86690,#86691,#86692,#86693,#86694,#86695,#86696,#86697,#86698,#86699,#86700,
#86701,#86702,#86703,#86704,#86705,#86706,#86707,#86708,#86709,#86710,#86711,
#86712,#86713,#86714,#86715,#86716,#86717,#86718,#86719,#86720,#86721,#86722,
#86723,#86724,#86725,#86726,#86727,#86728,#86729,#86730,#86731,#86732,#86733,
#86734,#86735,#86736,#86737,#86738,#86739,#86740,#86741,#86742,#86743,#86744,
#86745,#86746,#86747,#86748,#86749,#86750,#86751,#86752,#86753,#86754,#86755,
#86756,#86757,#86758,#86759,#86760,#86761,#86762,#86763,#86764,#86765,#86766,
#86767,#86768,#86769,#86770,#86771,#86772,#86773,#86774,#86775,#86776,#86777,
#86778,#86779,#86780,#86781,#86782,#86783,#86784,#86785,#86786,#86787,#86788,
#86789,#86790,#86791,#86792,#86793,#86794,#86795,#86796,#86797,#86798,#86799,
#86800,#86801,#86802,#86803,#86804,#86805,#86806,#86807,#86808,#86809,#86810,
#86811,#86812,#86813,#86814,#86815,#86816,#86817,#86818,#86819,#86820,#86821,
#86822,#86823,#86824,#86825,#86826,#86827,#86828,#86829,#86830,#86831,#86832,
#86833,#86834,#86835,#86836,#86837,#86838,#86839,#86840,#86841,#86842,#86843,
#86844,#86845,#86846,#86847,#86848,#86849,#86850,#86851,#86852,#86853,#86854),
 .UNSPECIFIED.,.F.,.F.,(4,3,3,3,3,3,3,3,3,3,3,3,3,3,3,3,3,3,3,3,3,3,3,3,
3,3,3,3,3,3,3,3,3,3,3,3,3,3,3,3,3,3,3,3,3,3,3,3,3,3,3,3,3,3,3,3,3,3,3,3,
4),(-10.1321597128207,-9.99259863041052,-9.9290141840265,-9.82992590097336,
-9.73097749788903,-9.63161940635588,-9.53284651231657,-9.43410583031699,
-9.33536761708367,-9.23555390421872,-9.13667450638263,-9.03639363600324,
-8.93611276562384,-8.83702221611555,-8.73807149297398,-8.63871397475489,
-8.53993864877712,-8.44119549854981,-8.34245478441589,-8.24264392511722,
-8.14376197274035,-8.04348665998078,-7.9432113472212,-7.84414230710637,
-7.74521316205596,-7.64585025790128,-7.54709651866685,-7.44837491048508,
-7.3496556646746,-7.24981923071059,-7.15095834782461,-7.05063413832158,
-6.95030992881855,-6.8512036523718,-6.75223732846605,-6.65288372620978,
-6.55409321601646,-6.45533507076485,-6.35657957005115,-6.25678680514234,
-6.15789072377564,-6.05764961709577,-5.9574085104159,-5.8582996906847,-5.75933043866179,
-5.65997752033072,-5.5611831793623,-5.46242087541135,-5.36366089601644,
-5.26387244501564,-5.16497115470896,-5.0647391233611,-4.96450709201325,
-4.86557234860677,-4.76676586361448,-4.66805750331981,-4.56941723767383,
-4.47078994099785,-4.37217346045678,-4.27348914445664,-4.20357440982612),
 .UNSPECIFIED.);
#738=B_SPLINE_CURVE_WITH_KNOTS('',3,(#86857,#86858,#86859,#86860,#86861,
#86862,#86863,#86864),.UNSPECIFIED.,.F.,.F.,(4,1,1,1,1,4),(17.934417062947,
18.8092987911264,19.802200209529,20.7951016279317,21.7880030463343,21.9911485751285),
 .UNSPECIFIED.);
#739=B_SPLINE_CURVE_WITH_KNOTS('',3,(#86865,#86866,#86867,#86868,#86869,
#86870,#86871,#86872,#86873,#86874,#86875,#86876,#86877,#86878,#86879,#86880,
#86881,#86882,#86883,#86884,#86885,#86886,#86887,#86888,#86889,#86890,#86891,
#86892,#86893,#86894,#86895,#86896,#86897,#86898,#86899,#86900,#86901,#86902,
#86903,#86904,#86905,#86906,#86907,#86908,#86909,#86910,#86911,#86912,#86913,
#86914,#86915,#86916,#86917,#86918,#86919,#86920,#86921,#86922,#86923,#86924,
#86925,#86926,#86927,#86928,#86929,#86930,#86931,#86932,#86933,#86934,#86935,
#86936,#86937,#86938,#86939,#86940),.UNSPECIFIED.,.F.,.F.,(4,3,3,3,3,3,
3,3,3,3,3,3,3,3,3,3,3,3,3,3,3,3,3,3,3,4),(21.9911485751285,22.0839073590714,
22.1765824116993,22.2692136891438,22.3618281746274,22.4544528291803,22.5471704847007,
22.6399399937748,22.7328552617387,22.780904464737,22.8751694663624,22.9693071643559,
23.0633460667357,23.1573182064377,23.2512564850146,23.3451865167536,23.4391339018238,
23.5331822013363,23.6272862468957,23.7215409230576,23.7738058831396,23.8680772171186,
23.9621978437796,24.0562310887038,24.1502000668644,24.2171289178558),
 .UNSPECIFIED.);
#740=B_SPLINE_CURVE_WITH_KNOTS('',3,(#86942,#86943,#86944,#86945,#86946,
#86947),.UNSPECIFIED.,.F.,.F.,(4,1,1,4),(21.9911557963905,22.3416114741931,
23.3345128925957,24.2163566964775),.UNSPECIFIED.);
#741=B_SPLINE_CURVE_WITH_KNOTS('',3,(#86948,#86949,#86950,#86951,#86952,
#86953,#86954,#86955,#86956,#86957,#86958,#86959,#86960,#86961,#86962,#86963,
#86964,#86965,#86966,#86967,#86968,#86969,#86970,#86971,#86972,#86973,#86974,
#86975,#86976,#86977,#86978,#86979,#86980,#86981,#86982,#86983,#86984,#86985,
#86986,#86987,#86988,#86989,#86990,#86991,#86992,#86993,#86994,#86995,#86996,
#86997,#86998,#86999,#87000,#87001,#87002,#87003,#87004,#87005,#87006,#87007,
#87008,#87009,#87010,#87011,#87012,#87013,#87014,#87015,#87016,#87017,#87018,
#87019,#87020,#87021,#87022,#87023,#87024,#87025,#87026,#87027,#87028,#87029,
#87030,#87031,#87032,#87033,#87034,#87035,#87036,#87037,#87038,#87039,#87040,
#87041,#87042,#87043,#87044,#87045,#87046,#87047,#87048,#87049,#87050,#87051,
#87052,#87053,#87054,#87055,#87056,#87057,#87058,#87059,#87060,#87061,#87062,
#87063,#87064,#87065,#87066,#87067,#87068,#87069,#87070,#87071,#87072,#87073,
#87074,#87075,#87076,#87077,#87078,#87079,#87080,#87081,#87082,#87083),
 .UNSPECIFIED.,.F.,.F.,(4,3,3,3,3,3,3,3,3,3,3,3,3,3,3,3,3,3,3,3,3,3,3,3,
3,3,3,3,3,3,3,3,3,3,3,3,3,3,3,3,3,3,3,3,3,4),(17.933562797591,18.027675652425,
18.1218896239166,18.2161582961348,18.3105802127554,18.3700058005825,18.4641580180287,
18.5581814190289,18.6521046770886,18.7459596395798,18.8397798343671,18.9335910183375,
19.0274189336518,19.121347534599,19.2153315750444,19.309466936441,19.3629072189851,
19.4571939175188,19.5513533907898,19.6454141155,19.7394080541651,19.8333681083284,
19.9273198645896,20.0212888953817,20.1153585868841,20.2094839117571,20.3037594805915,
20.3558086373878,20.4500899121047,20.5442442313676,20.6383000780776,20.73228957412,
20.8262454576189,20.9201933215444,21.0141587449332,21.1082252887648,21.2023477218278,
21.2966208318784,21.3487100557904,21.4432580465324,21.5376780899157,21.6319955406164,
21.7262338036894,21.8204240372999,21.914613503733,21.9911485751285),
 .UNSPECIFIED.);
#742=B_SPLINE_CURVE_WITH_KNOTS('',3,(#87086,#87087,#87088,#87089,#87090,
#87091,#87092,#87093),.UNSPECIFIED.,.F.,.F.,(4,1,1,1,1,4),(17.9344169320433,
18.8092987911264,19.802200209529,20.7951016279317,21.7880030463343,21.9911485751285),
 .UNSPECIFIED.);
#743=B_SPLINE_CURVE_WITH_KNOTS('',3,(#87094,#87095,#87096,#87097,#87098,
#87099,#87100,#87101,#87102,#87103,#87104,#87105,#87106,#87107,#87108,#87109,
#87110,#87111,#87112,#87113,#87114,#87115,#87116,#87117,#87118,#87119,#87120,
#87121,#87122,#87123,#87124,#87125,#87126,#87127,#87128,#87129,#87130,#87131,
#87132,#87133,#87134,#87135,#87136,#87137,#87138,#87139,#87140,#87141,#87142,
#87143,#87144,#87145,#87146,#87147,#87148,#87149,#87150,#87151,#87152,#87153,
#87154,#87155,#87156,#87157,#87158,#87159,#87160,#87161,#87162,#87163,#87164,
#87165,#87166,#87167,#87168,#87169),.UNSPECIFIED.,.F.,.F.,(4,3,3,3,3,3,
3,3,3,3,3,3,3,3,3,3,3,3,3,3,3,3,3,3,3,4),(21.9911485751285,22.0839073709794,
22.1765824356426,22.2692137252015,22.3618282228698,22.4544528896688,22.5471705574739,
22.6399400788727,22.7328553591282,22.780904464737,22.8751694611138,22.9693071538032,
23.0633460508314,23.157318185133,23.2512564582814,23.3451864845702,23.4391338641752,
23.5331821582336,23.6272861983369,23.7215408690931,23.7738058831396,23.8680772168287,
23.9621978431654,24.056231087749,24.1502000655167,24.2171287697742),
 .UNSPECIFIED.);
#744=B_SPLINE_CURVE_WITH_KNOTS('',3,(#87171,#87172,#87173,#87174,#87175,
#87176),.UNSPECIFIED.,.F.,.F.,(4,1,1,4),(21.9911557978734,22.3416114741931,
23.3345128925957,24.2163565526082),.UNSPECIFIED.);
#745=B_SPLINE_CURVE_WITH_KNOTS('',3,(#87177,#87178,#87179,#87180,#87181,
#87182,#87183,#87184,#87185,#87186,#87187,#87188,#87189,#87190,#87191,#87192,
#87193,#87194,#87195,#87196,#87197,#87198,#87199,#87200,#87201,#87202,#87203,
#87204,#87205,#87206,#87207,#87208,#87209,#87210,#87211,#87212,#87213,#87214,
#87215,#87216,#87217,#87218,#87219,#87220,#87221,#87222,#87223,#87224,#87225,
#87226,#87227,#87228,#87229,#87230,#87231,#87232,#87233,#87234,#87235,#87236,
#87237,#87238,#87239,#87240,#87241,#87242,#87243,#87244,#87245,#87246,#87247,
#87248,#87249,#87250,#87251,#87252,#87253,#87254,#87255,#87256,#87257,#87258,
#87259,#87260,#87261,#87262,#87263,#87264,#87265,#87266,#87267,#87268,#87269,
#87270,#87271,#87272,#87273,#87274,#87275,#87276,#87277,#87278,#87279,#87280,
#87281,#87282,#87283,#87284,#87285,#87286,#87287,#87288,#87289,#87290,#87291,
#87292,#87293,#87294,#87295,#87296,#87297,#87298,#87299,#87300,#87301,#87302,
#87303,#87304,#87305,#87306,#87307,#87308,#87309,#87310,#87311,#87312),
 .UNSPECIFIED.,.F.,.F.,(4,3,3,3,3,3,3,3,3,3,3,3,3,3,3,3,3,3,3,3,3,3,3,3,
3,3,3,3,3,3,3,3,3,3,3,3,3,3,3,3,3,3,3,3,3,4),(17.9335626655157,18.0276756704584,
18.1218897949067,18.2161586217505,18.310580694799,18.3700058005825,18.4641576524374,
18.5581806828801,18.6521035659322,18.7459581482699,18.8397779598427,18.9335887579803,
19.0274162852848,19.1213444971949,19.2153281474366,19.3094631205816,19.3629072189851,
19.4571940776216,19.551353712538,19.6454146002015,19.7394087030847,19.8333689221839,
19.9273208438937,20.0212900404422,20.1153598971617,20.2094853871854,20.3037611194529,
20.3558086373878,20.4500899460874,20.5442443002541,20.6383001827375,20.7322897157095,
20.8262456368411,20.9201935390591,21.0141590013572,21.1082255848112,21.2023480579584,
21.2966212084346,21.3487100557904,21.4432579779742,21.537677951789,21.6319953320113,
21.7262335235201,21.8204236849522,21.9146130786406,21.9911485751285),
 .UNSPECIFIED.);
#746=B_SPLINE_CURVE_WITH_KNOTS('',3,(#87486,#87487,#87488,#87489,#87490,
#87491,#87492,#87493,#87494,#87495,#87496,#87497,#87498,#87499,#87500,#87501,
#87502,#87503,#87504,#87505,#87506,#87507,#87508,#87509,#87510,#87511,#87512,
#87513,#87514,#87515,#87516,#87517,#87518,#87519,#87520,#87521,#87522,#87523,
#87524,#87525,#87526,#87527,#87528,#87529,#87530,#87531,#87532,#87533,#87534,
#87535,#87536,#87537,#87538,#87539,#87540,#87541,#87542,#87543,#87544,#87545,
#87546,#87547,#87548,#87549,#87550,#87551,#87552,#87553,#87554,#87555,#87556,
#87557,#87558,#87559,#87560,#87561,#87562,#87563,#87564,#87565,#87566,#87567,
#87568,#87569,#87570,#87571,#87572,#87573,#87574,#87575,#87576),
 .UNSPECIFIED.,.F.,.F.,(4,3,3,3,3,3,3,3,3,3,3,3,3,3,3,3,3,3,3,3,3,3,3,3,
3,3,3,3,3,3,4),(0.,0.0300159935056151,0.0604743500360521,0.0909579961729321,
0.11495774109072,0.120628826798375,0.150390662795823,0.179990444032073,
0.208918759997128,0.22052111292651,0.229057706928878,0.233702755111811,
0.26200301285018,0.290174366185419,0.294101824832485,0.323060492781776,
0.339554831971467,0.343320212454064,0.371322118638722,0.399422729592019,
0.427289788372197,0.437570748201759,0.44383438261869,0.448938125741618,
0.476009686934302,0.498103681939219,0.50628921912477,0.511794812399658,
0.537727274345166,0.561316539907562,0.569248610399424),.UNSPECIFIED.);
#747=B_SPLINE_CURVE_WITH_KNOTS('',3,(#87577,#87578,#87579,#87580,#87581,
#87582,#87583,#87584,#87585,#87586,#87587,#87588,#87589,#87590,#87591,#87592,
#87593,#87594,#87595,#87596,#87597,#87598,#87599,#87600,#87601,#87602,#87603,
#87604,#87605,#87606,#87607,#87608,#87609,#87610,#87611,#87612,#87613,#87614,
#87615,#87616,#87617,#87618,#87619,#87620,#87621,#87622,#87623,#87624,#87625,
#87626,#87627,#87628,#87629,#87630,#87631,#87632,#87633,#87634,#87635,#87636,
#87637,#87638,#87639,#87640,#87641,#87642,#87643,#87644,#87645,#87646,#87647,
#87648,#87649,#87650,#87651,#87652,#87653,#87654,#87655,#87656,#87657,#87658,
#87659,#87660,#87661,#87662,#87663,#87664),.UNSPECIFIED.,.F.,.F.,(4,3,3,
3,3,3,3,3,3,3,3,3,3,3,3,3,3,3,3,3,3,3,3,3,3,3,3,3,3,4),(0.,0.0255422152389494,
0.0516177884235197,0.0783410487135325,0.0899179575897014,0.096618619084006,
0.102681367695304,0.130058793828978,0.157808810247486,0.185592138961451,
0.195924569149338,0.202922297119531,0.206879012885186,0.236200442199667,
0.265521871514148,0.293412035650182,0.309408739020944,0.314635271121598,
0.343053617094055,0.372027540249262,0.401483685393919,0.421616489784836,
0.426693998849235,0.456850944397209,0.481878239127351,0.490063670760061,
0.498374798665562,0.528883352060159,0.557282026181539,0.566784192699823),
 .UNSPECIFIED.);
#748=B_SPLINE_CURVE_WITH_KNOTS('',3,(#87665,#87666,#87667,#87668),
 .UNSPECIFIED.,.F.,.F.,(4,4),(-0.0155024185535969,0.),.UNSPECIFIED.);
#749=B_SPLINE_CURVE_WITH_KNOTS('',3,(#87841,#87842,#87843,#87844,#87845,
#87846,#87847,#87848,#87849,#87850,#87851,#87852,#87853,#87854,#87855,#87856,
#87857,#87858,#87859,#87860,#87861,#87862,#87863,#87864,#87865,#87866,#87867,
#87868,#87869,#87870,#87871,#87872,#87873,#87874,#87875,#87876,#87877,#87878,
#87879,#87880,#87881,#87882,#87883,#87884,#87885,#87886,#87887,#87888,#87889,
#87890,#87891,#87892,#87893,#87894,#87895,#87896,#87897,#87898,#87899,#87900,
#87901,#87902,#87903,#87904,#87905,#87906,#87907,#87908,#87909,#87910,#87911,
#87912,#87913,#87914,#87915,#87916,#87917,#87918,#87919,#87920,#87921,#87922,
#87923,#87924,#87925,#87926,#87927,#87928),.UNSPECIFIED.,.F.,.F.,(4,3,3,
3,3,3,3,3,3,3,3,3,3,3,3,3,3,3,3,3,3,3,3,3,3,3,3,3,3,4),(1.04239282054807E-14,
0.0254572747588063,0.0518172438748224,0.0781772129908385,0.0966186262417464,
0.103162062894422,0.130547954004623,0.158302436395126,0.186083150718936,
0.195924591412827,0.202922307188184,0.206879036916929,0.236200454215543,
0.265521871514156,0.293411964117121,0.302822187650876,0.3094079319206,0.314634984029602,
0.343053229098208,0.372027084515964,0.401483217598252,0.421615452936291,
0.426694040216341,0.456850977316032,0.481878254523113,0.49006368288519,
0.499045747647966,0.529549458312069,0.557282026181566,0.566816216565832),
 .UNSPECIFIED.);
#750=B_SPLINE_CURVE_WITH_KNOTS('',3,(#87929,#87930,#87931,#87932,#87933,
#87934,#87935,#87936,#87937,#87938,#87939,#87940,#87941,#87942,#87943,#87944,
#87945,#87946,#87947,#87948,#87949,#87950,#87951,#87952,#87953,#87954,#87955,
#87956,#87957,#87958,#87959,#87960,#87961,#87962,#87963,#87964,#87965,#87966,
#87967,#87968,#87969,#87970,#87971,#87972,#87973,#87974,#87975,#87976,#87977,
#87978,#87979,#87980,#87981,#87982,#87983,#87984,#87985,#87986,#87987,#87988,
#87989,#87990,#87991,#87992,#87993,#87994,#87995,#87996,#87997,#87998,#87999,
#88000,#88001,#88002,#88003,#88004,#88005,#88006,#88007,#88008,#88009,#88010,
#88011,#88012,#88013,#88014,#88015,#88016,#88017,#88018,#88019),
 .UNSPECIFIED.,.F.,.F.,(4,3,3,3,3,3,3,3,3,3,3,3,3,3,3,3,3,3,3,3,3,3,3,3,
3,3,3,3,3,3,4),(0.,0.0300160900779859,0.0604744914019228,0.0909581108839495,
0.114957874464915,0.120628837064466,0.150390666664299,0.179990414269659,
0.20891869318285,0.220521069668172,0.229057577762524,0.233702774585337,
0.262002994102814,0.290174314790119,0.294101824832485,0.323060497067606,
0.339554809732512,0.343320179866502,0.371322084504482,0.399422690124115,
0.427289724843109,0.437570609423,0.443833557401397,0.448938172443596,0.476009696567213,
0.498103708209085,0.506289235973561,0.511794807845771,0.537727197803124,
0.561316539907572,0.569248610399431),.UNSPECIFIED.);
#751=B_SPLINE_CURVE_WITH_KNOTS('',3,(#88029,#88030,#88031,#88032,#88033,
#88034,#88035,#88036,#88037,#88038,#88039,#88040,#88041,#88042,#88043,#88044,
#88045,#88046,#88047,#88048,#88049,#88050,#88051,#88052,#88053,#88054,#88055,
#88056,#88057,#88058,#88059,#88060,#88061,#88062,#88063,#88064,#88065,#88066,
#88067,#88068,#88069,#88070,#88071,#88072,#88073,#88074,#88075,#88076,#88077,
#88078,#88079,#88080,#88081,#88082,#88083,#88084,#88085,#88086,#88087,#88088,
#88089,#88090,#88091,#88092,#88093,#88094,#88095,#88096,#88097,#88098,#88099,
#88100,#88101,#88102,#88103,#88104,#88105,#88106,#88107,#88108,#88109,#88110,
#88111,#88112,#88113,#88114,#88115,#88116,#88117,#88118,#88119),
 .UNSPECIFIED.,.F.,.F.,(4,3,3,3,3,3,3,3,3,3,3,3,3,3,3,3,3,3,3,3,3,3,3,3,
3,3,3,3,3,3,4),(0.,0.025457205048592,0.0518171512135332,0.0781770973784744,
0.0899179847267486,0.0966186227065892,0.102681367591522,0.129991616367842,
0.157832389105944,0.184687665901973,0.195924580418245,0.202922302220591,
0.206879025059384,0.236200448286765,0.265521871514145,0.29342151830769,
0.302822262870922,0.309408330719355,0.314635125840642,0.343053420777207,
0.372027309636075,0.40148344864646,0.421615965153544,0.426694019602539,
0.456850960866328,0.481878246781235,0.491733467196207,0.498374793580113,
0.528883346995961,0.557282026181531,0.566784188998617),.UNSPECIFIED.);
#752=B_SPLINE_CURVE_WITH_KNOTS('',3,(#88120,#88121,#88122,#88123,#88124,
#88125,#88126,#88127,#88128,#88129,#88130,#88131,#88132,#88133,#88134,#88135,
#88136,#88137,#88138,#88139,#88140,#88141,#88142,#88143,#88144,#88145,#88146,
#88147,#88148,#88149,#88150,#88151,#88152,#88153,#88154,#88155,#88156,#88157,
#88158,#88159,#88160,#88161,#88162,#88163,#88164,#88165,#88166,#88167,#88168,
#88169,#88170,#88171,#88172,#88173,#88174,#88175,#88176,#88177,#88178,#88179,
#88180,#88181,#88182,#88183,#88184,#88185,#88186,#88187,#88188,#88189,#88190,
#88191,#88192,#88193,#88194,#88195,#88196,#88197,#88198,#88199,#88200,#88201,
#88202,#88203,#88204,#88205,#88206,#88207,#88208,#88209,#88210),
 .UNSPECIFIED.,.F.,.F.,(4,3,3,3,3,3,3,3,3,3,3,3,3,3,3,3,3,3,3,3,3,3,3,3,
3,3,3,3,3,3,4),(0.,0.0300160333477477,0.0604744083323999,0.0909580434563729,
0.114957796091441,0.120628831026791,0.150388839258673,0.179796669056497,
0.208512063304176,0.220521095101031,0.229057653709693,0.23370276314254,
0.262003005144642,0.290174345004673,0.294101824832486,0.323048758434001,
0.339554822814053,0.343320199032514,0.371322104568047,0.399422713338306,
0.42728976222237,0.437570691067827,0.443834042831826,0.448938144811474,
0.476009690744306,0.498103692666017,0.506289225879212,0.511794810465465,
0.537727242743261,0.561316539907572,0.569248610399431),.UNSPECIFIED.);
#753=B_SPLINE_CURVE_WITH_KNOTS('',3,(#88386,#88387,#88388,#88389,#88390,
#88391,#88392,#88393,#88394,#88395,#88396,#88397,#88398,#88399,#88400,#88401,
#88402,#88403,#88404,#88405,#88406,#88407,#88408,#88409,#88410,#88411,#88412,
#88413,#88414,#88415,#88416,#88417,#88418,#88419,#88420,#88421,#88422,#88423,
#88424,#88425,#88426,#88427,#88428,#88429,#88430,#88431,#88432,#88433,#88434,
#88435,#88436,#88437,#88438,#88439,#88440,#88441,#88442,#88443,#88444,#88445,
#88446,#88447,#88448,#88449,#88450,#88451,#88452,#88453,#88454,#88455,#88456,
#88457,#88458,#88459,#88460,#88461,#88462,#88463,#88464,#88465,#88466,#88467,
#88468,#88469,#88470,#88471,#88472,#88473,#88474,#88475,#88476),
 .UNSPECIFIED.,.F.,.F.,(4,3,3,3,3,3,3,3,3,3,3,3,3,3,3,3,3,3,3,3,3,3,3,3,
3,3,3,3,3,3,4),(0.,0.030016042371606,0.0604744215895692,0.0909580542444513,
0.114957808579322,0.120628831988276,0.150388840111643,0.17979666618708,
0.2085120615786,0.220521091051168,0.229057641618228,0.233702764936734,0.262003003352699,
0.290174340161946,0.294101824832484,0.32306049493075,0.339554820728239,
0.343320195973592,0.371362527908372,0.399540213697088,0.427306356009437,
0.437570678055961,0.443833965453209,0.448938149214107,0.47703274688747,
0.498103695142492,0.506289227485511,0.512902840722385,0.538820003579557,
0.561316539907558,0.56924861039942),.UNSPECIFIED.);
#754=B_SPLINE_CURVE_WITH_KNOTS('',3,(#88477,#88478,#88479,#88480),
 .UNSPECIFIED.,.F.,.F.,(4,4),(-0.0155031780625747,0.),.UNSPECIFIED.);
#755=B_SPLINE_CURVE_WITH_KNOTS('',3,(#88653,#88654,#88655,#88656,#88657,
#88658,#88659,#88660,#88661,#88662,#88663,#88664,#88665,#88666,#88667,#88668,
#88669,#88670,#88671,#88672,#88673,#88674,#88675,#88676,#88677,#88678,#88679,
#88680,#88681,#88682,#88683,#88684,#88685,#88686,#88687,#88688,#88689,#88690,
#88691,#88692,#88693,#88694,#88695,#88696,#88697,#88698,#88699,#88700,#88701,
#88702,#88703,#88704,#88705,#88706,#88707,#88708,#88709,#88710,#88711,#88712,
#88713,#88714,#88715,#88716,#88717,#88718,#88719,#88720,#88721,#88722,#88723,
#88724,#88725,#88726,#88727,#88728,#88729,#88730,#88731,#88732,#88733,#88734,
#88735,#88736,#88737,#88738,#88739,#88740,#88741,#88742,#88743),
 .UNSPECIFIED.,.F.,.F.,(4,3,3,3,3,3,3,3,3,3,3,3,3,3,3,3,3,3,3,3,3,3,3,3,
3,3,3,3,3,3,4),(0.,0.0254571918318206,0.0518171336468171,0.0781770754618136,
0.089917979704679,0.0966186220362691,0.102681367599265,0.129991607231578,
0.157832378191868,0.184687655883825,0.195924578330426,0.202922301283516,
0.206879022820041,0.236200447167097,0.265521871514153,0.293412006162953,
0.302822277125942,0.309408406301434,0.31463515273045,0.343053457095624,
0.372027352294228,0.401483492527513,0.421616062260858,0.426694015683236,
0.456850957722602,0.481878245307923,0.490063675457469,0.498374794492553,
0.528883347928461,0.557282026181522,0.566816364269905),.UNSPECIFIED.);
#897=SHAPE_REPRESENTATION_RELATIONSHIP('SRR','None',#105865,#909);
#909=ADVANCED_BREP_SHAPE_REPRESENTATION('',(#933),#105800);
#921=STYLED_ITEM('',(#105930),#933);
#933=MANIFOLD_SOLID_BREP('Body1',#7208);
#983=FACE_BOUND('',#1582,.T.);
#984=FACE_BOUND('',#1583,.T.);
#985=FACE_BOUND('',#1584,.T.);
#986=FACE_BOUND('',#1593,.T.);
#987=FACE_BOUND('',#1594,.T.);
#988=FACE_BOUND('',#1595,.T.);
#1036=PLANE('',#7620);
#1037=PLANE('',#7624);
#1038=PLANE('',#7625);
#1039=PLANE('',#7626);
#1040=PLANE('',#7627);
#1041=PLANE('',#7628);
#1235=FACE_OUTER_BOUND('',#1551,.T.);
#1236=FACE_OUTER_BOUND('',#1552,.T.);
#1237=FACE_OUTER_BOUND('',#1553,.T.);
#1238=FACE_OUTER_BOUND('',#1554,.T.);
#1239=FACE_OUTER_BOUND('',#1555,.T.);
#1240=FACE_OUTER_BOUND('',#1556,.T.);
#1241=FACE_OUTER_BOUND('',#1557,.T.);
#1242=FACE_OUTER_BOUND('',#1558,.T.);
#1243=FACE_OUTER_BOUND('',#1559,.T.);
#1244=FACE_OUTER_BOUND('',#1560,.T.);
#1245=FACE_OUTER_BOUND('',#1561,.T.);
#1246=FACE_OUTER_BOUND('',#1562,.T.);
#1247=FACE_OUTER_BOUND('',#1563,.T.);
#1248=FACE_OUTER_BOUND('',#1564,.T.);
#1249=FACE_OUTER_BOUND('',#1565,.T.);
#1250=FACE_OUTER_BOUND('',#1566,.T.);
#1251=FACE_OUTER_BOUND('',#1567,.T.);
#1252=FACE_OUTER_BOUND('',#1568,.T.);
#1253=FACE_OUTER_BOUND('',#1569,.T.);
#1254=FACE_OUTER_BOUND('',#1570,.T.);
#1255=FACE_OUTER_BOUND('',#1571,.T.);
#1256=FACE_OUTER_BOUND('',#1572,.T.);
#1257=FACE_OUTER_BOUND('',#1573,.T.);
#1258=FACE_OUTER_BOUND('',#1574,.T.);
#1259=FACE_OUTER_BOUND('',#1575,.T.);
#1260=FACE_OUTER_BOUND('',#1576,.T.);
#1261=FACE_OUTER_BOUND('',#1577,.T.);
#1262=FACE_OUTER_BOUND('',#1578,.T.);
#1263=FACE_OUTER_BOUND('',#1579,.T.);
#1264=FACE_OUTER_BOUND('',#1580,.T.);
#1265=FACE_OUTER_BOUND('',#1581,.T.);
#1266=FACE_OUTER_BOUND('',#1585,.T.);
#1267=FACE_OUTER_BOUND('',#1586,.T.);
#1268=FACE_OUTER_BOUND('',#1587,.T.);
#1269=FACE_OUTER_BOUND('',#1588,.T.);
#1270=FACE_OUTER_BOUND('',#1589,.T.);
#1271=FACE_OUTER_BOUND('',#1590,.T.);
#1272=FACE_OUTER_BOUND('',#1591,.T.);
#1273=FACE_OUTER_BOUND('',#1592,.T.);
#1551=EDGE_LOOP('',(#5979,#5980,#5981,#5982));
#1552=EDGE_LOOP('',(#5983,#5984,#5985,#5986,#5987,#5988));
#1553=EDGE_LOOP('',(#5989,#5990,#5991,#5992,#5993,#5994));
#1554=EDGE_LOOP('',(#5995,#5996,#5997,#5998,#5999,#6000));
#1555=EDGE_LOOP('',(#6001,#6002,#6003,#6004,#6005,#6006));
#1556=EDGE_LOOP('',(#6007,#6008,#6009,#6010,#6011,#6012));
#1557=EDGE_LOOP('',(#6013,#6014,#6015,#6016));
#1558=EDGE_LOOP('',(#6017,#6018,#6019,#6020,#6021,#6022));
#1559=EDGE_LOOP('',(#6023,#6024,#6025,#6026,#6027,#6028));
#1560=EDGE_LOOP('',(#6029,#6030,#6031,#6032,#6033,#6034));
#1561=EDGE_LOOP('',(#6035,#6036,#6037,#6038,#6039,#6040));
#1562=EDGE_LOOP('',(#6041,#6042,#6043,#6044,#6045,#6046));
#1563=EDGE_LOOP('',(#6047,#6048,#6049,#6050));
#1564=EDGE_LOOP('',(#6051,#6052,#6053,#6054,#6055));
#1565=EDGE_LOOP('',(#6056,#6057,#6058,#6059,#6060,#6061));
#1566=EDGE_LOOP('',(#6062,#6063,#6064,#6065,#6066));
#1567=EDGE_LOOP('',(#6067,#6068,#6069,#6070,#6071,#6072));
#1568=EDGE_LOOP('',(#6073,#6074,#6075,#6076,#6077,#6078));
#1569=EDGE_LOOP('',(#6079,#6080,#6081,#6082));
#1570=EDGE_LOOP('',(#6083,#6084,#6085,#6086,#6087));
#1571=EDGE_LOOP('',(#6088,#6089,#6090,#6091,#6092,#6093));
#1572=EDGE_LOOP('',(#6094,#6095,#6096,#6097,#6098));
#1573=EDGE_LOOP('',(#6099,#6100,#6101,#6102,#6103,#6104));
#1574=EDGE_LOOP('',(#6105,#6106,#6107,#6108,#6109,#6110));
#1575=EDGE_LOOP('',(#6111,#6112,#6113,#6114,#6115,#6116));
#1576=EDGE_LOOP('',(#6117,#6118,#6119,#6120,#6121,#6122));
#1577=EDGE_LOOP('',(#6123,#6124,#6125,#6126,#6127,#6128));
#1578=EDGE_LOOP('',(#6129,#6130,#6131,#6132,#6133,#6134));
#1579=EDGE_LOOP('',(#6135,#6136,#6137,#6138,#6139,#6140,#6141,#6142,#6143,
#6144,#6145,#6146,#6147,#6148,#6149,#6150,#6151,#6152,#6153,#6154,#6155,
#6156,#6157,#6158,#6159,#6160,#6161));
#1580=EDGE_LOOP('',(#6162,#6163,#6164,#6165,#6166,#6167,#6168,#6169,#6170,
#6171,#6172,#6173,#6174,#6175,#6176,#6177,#6178,#6179,#6180,#6181,#6182,
#6183,#6184,#6185,#6186,#6187,#6188,#6189));
#1581=EDGE_LOOP('',(#6190,#6191,#6192,#6193));
#1582=EDGE_LOOP('',(#6194,#6195,#6196,#6197));
#1583=EDGE_LOOP('',(#6198,#6199,#6200,#6201));
#1584=EDGE_LOOP('',(#6202));
#1585=EDGE_LOOP('',(#6203,#6204,#6205,#6206,#6207,#6208,#6209,#6210,#6211,
#6212,#6213,#6214,#6215,#6216,#6217,#6218,#6219,#6220,#6221,#6222,#6223,
#6224,#6225,#6226,#6227,#6228,#6229));
#1586=EDGE_LOOP('',(#6230,#6231,#6232,#6233,#6234,#6235,#6236,#6237,#6238,
#6239,#6240,#6241,#6242,#6243,#6244,#6245,#6246,#6247,#6248,#6249,#6250,
#6251,#6252,#6253,#6254,#6255,#6256,#6257));
#1587=EDGE_LOOP('',(#6258,#6259,#6260,#6261));
#1588=EDGE_LOOP('',(#6262,#6263,#6264,#6265));
#1589=EDGE_LOOP('',(#6266,#6267,#6268,#6269));
#1590=EDGE_LOOP('',(#6270,#6271,#6272,#6273));
#1591=EDGE_LOOP('',(#6274,#6275,#6276,#6277));
#1592=EDGE_LOOP('',(#6278,#6279,#6280,#6281));
#1593=EDGE_LOOP('',(#6282,#6283,#6284,#6285,#6286));
#1594=EDGE_LOOP('',(#6287,#6288,#6289,#6290,#6291));
#1595=EDGE_LOOP('',(#6292));
#1851=LINE('',#79846,#2131);
#1852=LINE('',#79953,#2132);
#1853=LINE('',#80319,#2133);
#1854=LINE('',#80621,#2134);
#1855=LINE('',#80985,#2135);
#1856=LINE('',#81290,#2136);
#1857=LINE('',#81451,#2137);
#1858=LINE('',#81558,#2138);
#1859=LINE('',#81924,#2139);
#1860=LINE('',#82226,#2140);
#1861=LINE('',#82590,#2141);
#1862=LINE('',#82895,#2142);
#1863=LINE('',#83056,#2143);
#1864=LINE('',#83129,#2144);
#1865=LINE('',#83481,#2145);
#1866=LINE('',#83847,#2146);
#1867=LINE('',#84035,#2147);
#1868=LINE('',#84246,#2148);
#1869=LINE('',#84571,#2149);
#1870=LINE('',#84644,#2150);
#1871=LINE('',#84996,#2151);
#1872=LINE('',#85364,#2152);
#1873=LINE('',#85552,#2153);
#1874=LINE('',#85763,#2154);
#1875=LINE('',#88023,#2155);
#1876=LINE('',#88025,#2156);
#1877=LINE('',#88027,#2157);
#1878=LINE('',#88028,#2158);
#1879=LINE('',#88746,#2159);
#1880=LINE('',#88751,#2160);
#1881=LINE('',#88752,#2161);
#1882=LINE('',#88753,#2162);
#1883=LINE('',#88756,#2163);
#1884=LINE('',#88757,#2164);
#1885=LINE('',#88760,#2165);
#1886=LINE('',#88761,#2166);
#1887=LINE('',#88763,#2167);
#2131=VECTOR('',#8402,3.0735);
#2132=VECTOR('',#8407,3.0735);
#2133=VECTOR('',#8410,3.0735);
#2134=VECTOR('',#8413,3.0735);
#2135=VECTOR('',#8416,3.0735);
#2136=VECTOR('',#8419,3.0735);
#2137=VECTOR('',#8424,3.0735);
#2138=VECTOR('',#8429,3.0735);
#2139=VECTOR('',#8432,3.0735);
#2140=VECTOR('',#8435,3.0735);
#2141=VECTOR('',#8438,3.0735);
#2142=VECTOR('',#8441,3.0735);
#2143=VECTOR('',#8446,2.5175);
#2144=VECTOR('',#8451,2.5175);
#2145=VECTOR('',#8454,2.5175);
#2146=VECTOR('',#8457,2.5175);
#2147=VECTOR('',#8460,2.5175);
#2148=VECTOR('',#8463,2.5175);
#2149=VECTOR('',#8468,2.5175);
#2150=VECTOR('',#8473,2.5175);
#2151=VECTOR('',#8476,2.5175);
#2152=VECTOR('',#8479,2.5175);
#2153=VECTOR('',#8482,2.5175);
#2154=VECTOR('',#8485,2.5175);
#2155=VECTOR('',#8498,10.);
#2156=VECTOR('',#8499,10.);
#2157=VECTOR('',#8500,10.);
#2158=VECTOR('',#8501,10.);
#2159=VECTOR('',#8506,11.);
#2160=VECTOR('',#8511,10.);
#2161=VECTOR('',#8512,10.);
#2162=VECTOR('',#8513,10.);
#2163=VECTOR('',#8516,10.);
#2164=VECTOR('',#8517,10.);
#2165=VECTOR('',#8520,10.);
#2166=VECTOR('',#8521,10.);
#2167=VECTOR('',#8524,10.);
#2289=CIRCLE('',#7585,3.0735);
#2290=CIRCLE('',#7591,3.0735);
#2291=CIRCLE('',#7593,3.0735);
#2292=CIRCLE('',#7599,3.0735);
#2293=CIRCLE('',#7601,2.5175);
#2294=CIRCLE('',#7607,2.5175);
#2295=CIRCLE('',#7609,2.5175);
#2296=CIRCLE('',#7615,2.5175);
#2297=CIRCLE('',#7621,11.);
#2298=CIRCLE('',#7623,11.);
#2957=VERTEX_POINT('',#79844);
#2958=VERTEX_POINT('',#79845);
#2959=VERTEX_POINT('',#79847);
#2960=VERTEX_POINT('',#79854);
#2961=VERTEX_POINT('',#79951);
#2962=VERTEX_POINT('',#79952);
#2963=VERTEX_POINT('',#79954);
#2964=VERTEX_POINT('',#80097);
#2965=VERTEX_POINT('',#80317);
#2966=VERTEX_POINT('',#80318);
#2967=VERTEX_POINT('',#80320);
#2968=VERTEX_POINT('',#80405);
#2969=VERTEX_POINT('',#80619);
#2970=VERTEX_POINT('',#80620);
#2971=VERTEX_POINT('',#80622);
#2972=VERTEX_POINT('',#80769);
#2973=VERTEX_POINT('',#80983);
#2974=VERTEX_POINT('',#80984);
#2975=VERTEX_POINT('',#80986);
#2976=VERTEX_POINT('',#81199);
#2977=VERTEX_POINT('',#81288);
#2978=VERTEX_POINT('',#81289);
#2979=VERTEX_POINT('',#81291);
#2980=VERTEX_POINT('',#81368);
#2981=VERTEX_POINT('',#81374);
#2982=VERTEX_POINT('',#81376);
#2983=VERTEX_POINT('',#81449);
#2984=VERTEX_POINT('',#81450);
#2985=VERTEX_POINT('',#81452);
#2986=VERTEX_POINT('',#81459);
#2987=VERTEX_POINT('',#81556);
#2988=VERTEX_POINT('',#81557);
#2989=VERTEX_POINT('',#81559);
#2990=VERTEX_POINT('',#81702);
#2991=VERTEX_POINT('',#81922);
#2992=VERTEX_POINT('',#81923);
#2993=VERTEX_POINT('',#81925);
#2994=VERTEX_POINT('',#82010);
#2995=VERTEX_POINT('',#82224);
#2996=VERTEX_POINT('',#82225);
#2997=VERTEX_POINT('',#82227);
#2998=VERTEX_POINT('',#82374);
#2999=VERTEX_POINT('',#82588);
#3000=VERTEX_POINT('',#82589);
#3001=VERTEX_POINT('',#82591);
#3002=VERTEX_POINT('',#82804);
#3003=VERTEX_POINT('',#82893);
#3004=VERTEX_POINT('',#82894);
#3005=VERTEX_POINT('',#82896);
#3006=VERTEX_POINT('',#82973);
#3007=VERTEX_POINT('',#82979);
#3008=VERTEX_POINT('',#82981);
#3009=VERTEX_POINT('',#83054);
#3010=VERTEX_POINT('',#83055);
#3011=VERTEX_POINT('',#83057);
#3012=VERTEX_POINT('',#83068);
#3013=VERTEX_POINT('',#83127);
#3014=VERTEX_POINT('',#83128);
#3015=VERTEX_POINT('',#83130);
#3016=VERTEX_POINT('',#83479);
#3017=VERTEX_POINT('',#83480);
#3018=VERTEX_POINT('',#83482);
#3019=VERTEX_POINT('',#83683);
#3020=VERTEX_POINT('',#83845);
#3021=VERTEX_POINT('',#83846);
#3022=VERTEX_POINT('',#83848);
#3023=VERTEX_POINT('',#84033);
#3024=VERTEX_POINT('',#84034);
#3025=VERTEX_POINT('',#84036);
#3026=VERTEX_POINT('',#84222);
#3027=VERTEX_POINT('',#84244);
#3028=VERTEX_POINT('',#84245);
#3029=VERTEX_POINT('',#84247);
#3030=VERTEX_POINT('',#84261);
#3031=VERTEX_POINT('',#84380);
#3032=VERTEX_POINT('',#84382);
#3033=VERTEX_POINT('',#84569);
#3034=VERTEX_POINT('',#84570);
#3035=VERTEX_POINT('',#84572);
#3036=VERTEX_POINT('',#84583);
#3037=VERTEX_POINT('',#84642);
#3038=VERTEX_POINT('',#84643);
#3039=VERTEX_POINT('',#84645);
#3040=VERTEX_POINT('',#84994);
#3041=VERTEX_POINT('',#84995);
#3042=VERTEX_POINT('',#84997);
#3043=VERTEX_POINT('',#85198);
#3044=VERTEX_POINT('',#85362);
#3045=VERTEX_POINT('',#85363);
#3046=VERTEX_POINT('',#85365);
#3047=VERTEX_POINT('',#85550);
#3048=VERTEX_POINT('',#85551);
#3049=VERTEX_POINT('',#85553);
#3050=VERTEX_POINT('',#85739);
#3051=VERTEX_POINT('',#85761);
#3052=VERTEX_POINT('',#85762);
#3053=VERTEX_POINT('',#85764);
#3054=VERTEX_POINT('',#85778);
#3055=VERTEX_POINT('',#85897);
#3056=VERTEX_POINT('',#85899);
#3057=VERTEX_POINT('',#86086);
#3058=VERTEX_POINT('',#86284);
#3059=VERTEX_POINT('',#86471);
#3060=VERTEX_POINT('',#86669);
#3061=VERTEX_POINT('',#86856);
#3062=VERTEX_POINT('',#86941);
#3063=VERTEX_POINT('',#87085);
#3064=VERTEX_POINT('',#87170);
#3065=VERTEX_POINT('',#87485);
#3066=VERTEX_POINT('',#88021);
#3067=VERTEX_POINT('',#88022);
#3068=VERTEX_POINT('',#88024);
#3069=VERTEX_POINT('',#88026);
#3070=VERTEX_POINT('',#88211);
#3071=VERTEX_POINT('',#88385);
#3072=VERTEX_POINT('',#88745);
#3073=VERTEX_POINT('',#88749);
#3074=VERTEX_POINT('',#88750);
#3075=VERTEX_POINT('',#88755);
#3076=VERTEX_POINT('',#88759);
#4034=EDGE_CURVE('',#2957,#2958,#1851,.T.);
#4035=EDGE_CURVE('',#2958,#2959,#646,.T.);
#4036=EDGE_CURVE('',#2960,#2959,#2289,.T.);
#4037=EDGE_CURVE('',#2957,#2960,#647,.T.);
#4038=EDGE_CURVE('',#2961,#2962,#1852,.T.);
#4039=EDGE_CURVE('',#2962,#2963,#648,.T.);
#4040=EDGE_CURVE('',#2963,#2958,#649,.T.);
#4041=EDGE_CURVE('',#2964,#2957,#650,.T.);
#4042=EDGE_CURVE('',#2961,#2964,#651,.T.);
#4043=EDGE_CURVE('',#2965,#2966,#1853,.T.);
#4044=EDGE_CURVE('',#2966,#2967,#652,.T.);
#4045=EDGE_CURVE('',#2967,#2962,#653,.T.);
#4046=EDGE_CURVE('',#2968,#2961,#654,.T.);
#4047=EDGE_CURVE('',#2965,#2968,#655,.T.);
#4048=EDGE_CURVE('',#2969,#2970,#1854,.T.);
#4049=EDGE_CURVE('',#2970,#2971,#656,.T.);
#4050=EDGE_CURVE('',#2971,#2966,#657,.T.);
#4051=EDGE_CURVE('',#2972,#2965,#658,.T.);
#4052=EDGE_CURVE('',#2969,#2972,#659,.T.);
#4053=EDGE_CURVE('',#2973,#2974,#1855,.T.);
#4054=EDGE_CURVE('',#2974,#2975,#660,.T.);
#4055=EDGE_CURVE('',#2975,#2970,#661,.T.);
#4056=EDGE_CURVE('',#2976,#2969,#662,.T.);
#4057=EDGE_CURVE('',#2973,#2976,#663,.T.);
#4058=EDGE_CURVE('',#2977,#2978,#1856,.T.);
#4059=EDGE_CURVE('',#2979,#2977,#664,.T.);
#4060=EDGE_CURVE('',#2980,#2979,#665,.T.);
#4061=EDGE_CURVE('',#2981,#2980,#2290,.T.);
#4062=EDGE_CURVE('',#2981,#2982,#666,.T.);
#4063=EDGE_CURVE('',#2982,#2978,#667,.T.);
#4064=EDGE_CURVE('',#2983,#2984,#1857,.T.);
#4065=EDGE_CURVE('',#2984,#2985,#668,.T.);
#4066=EDGE_CURVE('',#2986,#2985,#2291,.T.);
#4067=EDGE_CURVE('',#2983,#2986,#669,.T.);
#4068=EDGE_CURVE('',#2987,#2988,#1858,.T.);
#4069=EDGE_CURVE('',#2988,#2989,#670,.T.);
#4070=EDGE_CURVE('',#2989,#2984,#671,.T.);
#4071=EDGE_CURVE('',#2990,#2983,#672,.T.);
#4072=EDGE_CURVE('',#2987,#2990,#673,.T.);
#4073=EDGE_CURVE('',#2991,#2992,#1859,.T.);
#4074=EDGE_CURVE('',#2992,#2993,#674,.T.);
#4075=EDGE_CURVE('',#2993,#2988,#675,.T.);
#4076=EDGE_CURVE('',#2994,#2987,#676,.T.);
#4077=EDGE_CURVE('',#2991,#2994,#677,.T.);
#4078=EDGE_CURVE('',#2995,#2996,#1860,.T.);
#4079=EDGE_CURVE('',#2996,#2997,#678,.T.);
#4080=EDGE_CURVE('',#2997,#2992,#679,.T.);
#4081=EDGE_CURVE('',#2998,#2991,#680,.T.);
#4082=EDGE_CURVE('',#2995,#2998,#681,.T.);
#4083=EDGE_CURVE('',#2999,#3000,#1861,.T.);
#4084=EDGE_CURVE('',#3000,#3001,#682,.T.);
#4085=EDGE_CURVE('',#3001,#2996,#683,.T.);
#4086=EDGE_CURVE('',#3002,#2995,#684,.T.);
#4087=EDGE_CURVE('',#2999,#3002,#685,.T.);
#4088=EDGE_CURVE('',#3003,#3004,#1862,.T.);
#4089=EDGE_CURVE('',#3005,#3003,#686,.T.);
#4090=EDGE_CURVE('',#3006,#3005,#687,.T.);
#4091=EDGE_CURVE('',#3007,#3006,#2292,.T.);
#4092=EDGE_CURVE('',#3007,#3008,#688,.T.);
#4093=EDGE_CURVE('',#3008,#3004,#689,.T.);
#4094=EDGE_CURVE('',#3009,#3010,#1863,.T.);
#4095=EDGE_CURVE('',#3010,#3011,#690,.T.);
#4096=EDGE_CURVE('',#3012,#3011,#2293,.F.);
#4097=EDGE_CURVE('',#3012,#3009,#691,.T.);
#4098=EDGE_CURVE('',#3013,#3014,#1864,.T.);
#4099=EDGE_CURVE('',#3014,#3015,#692,.T.);
#4100=EDGE_CURVE('',#3015,#3010,#693,.T.);
#4101=EDGE_CURVE('',#3009,#3013,#694,.T.);
#4102=EDGE_CURVE('',#3016,#3017,#1865,.T.);
#4103=EDGE_CURVE('',#3017,#3018,#695,.T.);
#4104=EDGE_CURVE('',#3018,#3014,#696,.T.);
#4105=EDGE_CURVE('',#3013,#3019,#697,.T.);
#4106=EDGE_CURVE('',#3019,#3016,#698,.T.);
#4107=EDGE_CURVE('',#3020,#3021,#1866,.T.);
#4108=EDGE_CURVE('',#3021,#3022,#699,.T.);
#4109=EDGE_CURVE('',#3022,#3017,#700,.T.);
#4110=EDGE_CURVE('',#3016,#3020,#701,.T.);
#4111=EDGE_CURVE('',#3023,#3024,#1867,.T.);
#4112=EDGE_CURVE('',#3024,#3025,#702,.T.);
#4113=EDGE_CURVE('',#3025,#3021,#703,.T.);
#4114=EDGE_CURVE('',#3020,#3026,#704,.T.);
#4115=EDGE_CURVE('',#3026,#3023,#705,.T.);
#4116=EDGE_CURVE('',#3027,#3028,#1868,.T.);
#4117=EDGE_CURVE('',#3027,#3029,#706,.T.);
#4118=EDGE_CURVE('',#3029,#3030,#707,.T.);
#4119=EDGE_CURVE('',#3031,#3030,#2294,.T.);
#4120=EDGE_CURVE('',#3031,#3032,#708,.T.);
#4121=EDGE_CURVE('',#3032,#3028,#709,.T.);
#4122=EDGE_CURVE('',#3033,#3034,#1869,.T.);
#4123=EDGE_CURVE('',#3034,#3035,#710,.T.);
#4124=EDGE_CURVE('',#3036,#3035,#2295,.F.);
#4125=EDGE_CURVE('',#3036,#3033,#711,.T.);
#4126=EDGE_CURVE('',#3037,#3038,#1870,.T.);
#4127=EDGE_CURVE('',#3038,#3039,#712,.T.);
#4128=EDGE_CURVE('',#3039,#3034,#713,.T.);
#4129=EDGE_CURVE('',#3033,#3037,#714,.T.);
#4130=EDGE_CURVE('',#3040,#3041,#1871,.T.);
#4131=EDGE_CURVE('',#3041,#3042,#715,.T.);
#4132=EDGE_CURVE('',#3042,#3038,#716,.T.);
#4133=EDGE_CURVE('',#3037,#3043,#717,.T.);
#4134=EDGE_CURVE('',#3043,#3040,#718,.T.);
#4135=EDGE_CURVE('',#3044,#3045,#1872,.T.);
#4136=EDGE_CURVE('',#3045,#3046,#719,.T.);
#4137=EDGE_CURVE('',#3046,#3041,#720,.T.);
#4138=EDGE_CURVE('',#3040,#3044,#721,.T.);
#4139=EDGE_CURVE('',#3047,#3048,#1873,.T.);
#4140=EDGE_CURVE('',#3048,#3049,#722,.T.);
#4141=EDGE_CURVE('',#3049,#3045,#723,.T.);
#4142=EDGE_CURVE('',#3044,#3050,#724,.T.);
#4143=EDGE_CURVE('',#3050,#3047,#725,.T.);
#4144=EDGE_CURVE('',#3051,#3052,#1874,.T.);
#4145=EDGE_CURVE('',#3051,#3053,#726,.T.);
#4146=EDGE_CURVE('',#3053,#3054,#727,.T.);
#4147=EDGE_CURVE('',#3055,#3054,#2296,.T.);
#4148=EDGE_CURVE('',#3055,#3056,#728,.T.);
#4149=EDGE_CURVE('',#3056,#3052,#729,.T.);
#4150=EDGE_CURVE('',#3052,#3057,#730,.T.);
#4151=EDGE_CURVE('',#3057,#3048,#731,.T.);
#4152=EDGE_CURVE('',#3047,#3058,#732,.T.);
#4153=EDGE_CURVE('',#3058,#3051,#733,.T.);
#4154=EDGE_CURVE('',#3028,#3059,#734,.T.);
#4155=EDGE_CURVE('',#3059,#3024,#735,.T.);
#4156=EDGE_CURVE('',#3023,#3060,#736,.T.);
#4157=EDGE_CURVE('',#3060,#3027,#737,.T.);
#4158=EDGE_CURVE('',#3004,#3061,#738,.T.);
#4159=EDGE_CURVE('',#3061,#3000,#739,.T.);
#4160=EDGE_CURVE('',#3062,#2999,#740,.T.);
#4161=EDGE_CURVE('',#3003,#3062,#741,.T.);
#4162=EDGE_CURVE('',#2978,#3063,#742,.T.);
#4163=EDGE_CURVE('',#3063,#2974,#743,.T.);
#4164=EDGE_CURVE('',#3064,#2973,#744,.T.);
#4165=EDGE_CURVE('',#2977,#3064,#745,.T.);
#4166=EDGE_CURVE('',#2959,#3065,#746,.T.);
#4167=EDGE_CURVE('',#3054,#2981,#747,.T.);
#4168=EDGE_CURVE('',#3065,#3036,#748,.T.);
#4169=EDGE_CURVE('',#3035,#2960,#749,.T.);
#4170=EDGE_CURVE('',#2980,#3055,#750,.T.);
#4171=EDGE_CURVE('',#3066,#3067,#1875,.T.);
#4172=EDGE_CURVE('',#3067,#3068,#1876,.T.);
#4173=EDGE_CURVE('',#3068,#3069,#1877,.T.);
#4174=EDGE_CURVE('',#3069,#3066,#1878,.T.);
#4175=EDGE_CURVE('',#3030,#3007,#751,.T.);
#4176=EDGE_CURVE('',#3006,#3031,#752,.T.);
#4177=EDGE_CURVE('',#3070,#3070,#2297,.T.);
#4178=EDGE_CURVE('',#2985,#3071,#753,.T.);
#4179=EDGE_CURVE('',#3071,#3012,#754,.T.);
#4180=EDGE_CURVE('',#3011,#2986,#755,.T.);
#4181=EDGE_CURVE('',#3070,#3072,#1879,.T.);
#4182=EDGE_CURVE('',#3072,#3072,#2298,.T.);
#4183=EDGE_CURVE('',#3073,#3074,#1880,.T.);
#4184=EDGE_CURVE('',#3074,#3066,#1881,.T.);
#4185=EDGE_CURVE('',#3073,#3069,#1882,.T.);
#4186=EDGE_CURVE('',#3075,#3073,#1883,.T.);
#4187=EDGE_CURVE('',#3075,#3068,#1884,.T.);
#4188=EDGE_CURVE('',#3076,#3075,#1885,.T.);
#4189=EDGE_CURVE('',#3076,#3067,#1886,.T.);
#4190=EDGE_CURVE('',#3074,#3076,#1887,.T.);
#5979=ORIENTED_EDGE('',*,*,#4034,.T.);
#5980=ORIENTED_EDGE('',*,*,#4035,.T.);
#5981=ORIENTED_EDGE('',*,*,#4036,.F.);
#5982=ORIENTED_EDGE('',*,*,#4037,.F.);
#5983=ORIENTED_EDGE('',*,*,#4038,.T.);
#5984=ORIENTED_EDGE('',*,*,#4039,.T.);
#5985=ORIENTED_EDGE('',*,*,#4040,.T.);
#5986=ORIENTED_EDGE('',*,*,#4034,.F.);
#5987=ORIENTED_EDGE('',*,*,#4041,.F.);
#5988=ORIENTED_EDGE('',*,*,#4042,.F.);
#5989=ORIENTED_EDGE('',*,*,#4043,.T.);
#5990=ORIENTED_EDGE('',*,*,#4044,.T.);
#5991=ORIENTED_EDGE('',*,*,#4045,.T.);
#5992=ORIENTED_EDGE('',*,*,#4038,.F.);
#5993=ORIENTED_EDGE('',*,*,#4046,.F.);
#5994=ORIENTED_EDGE('',*,*,#4047,.F.);
#5995=ORIENTED_EDGE('',*,*,#4048,.T.);
#5996=ORIENTED_EDGE('',*,*,#4049,.T.);
#5997=ORIENTED_EDGE('',*,*,#4050,.T.);
#5998=ORIENTED_EDGE('',*,*,#4043,.F.);
#5999=ORIENTED_EDGE('',*,*,#4051,.F.);
#6000=ORIENTED_EDGE('',*,*,#4052,.F.);
#6001=ORIENTED_EDGE('',*,*,#4053,.T.);
#6002=ORIENTED_EDGE('',*,*,#4054,.T.);
#6003=ORIENTED_EDGE('',*,*,#4055,.T.);
#6004=ORIENTED_EDGE('',*,*,#4048,.F.);
#6005=ORIENTED_EDGE('',*,*,#4056,.F.);
#6006=ORIENTED_EDGE('',*,*,#4057,.F.);
#6007=ORIENTED_EDGE('',*,*,#4058,.F.);
#6008=ORIENTED_EDGE('',*,*,#4059,.F.);
#6009=ORIENTED_EDGE('',*,*,#4060,.F.);
#6010=ORIENTED_EDGE('',*,*,#4061,.F.);
#6011=ORIENTED_EDGE('',*,*,#4062,.T.);
#6012=ORIENTED_EDGE('',*,*,#4063,.T.);
#6013=ORIENTED_EDGE('',*,*,#4064,.T.);
#6014=ORIENTED_EDGE('',*,*,#4065,.T.);
#6015=ORIENTED_EDGE('',*,*,#4066,.F.);
#6016=ORIENTED_EDGE('',*,*,#4067,.F.);
#6017=ORIENTED_EDGE('',*,*,#4068,.T.);
#6018=ORIENTED_EDGE('',*,*,#4069,.T.);
#6019=ORIENTED_EDGE('',*,*,#4070,.T.);
#6020=ORIENTED_EDGE('',*,*,#4064,.F.);
#6021=ORIENTED_EDGE('',*,*,#4071,.F.);
#6022=ORIENTED_EDGE('',*,*,#4072,.F.);
#6023=ORIENTED_EDGE('',*,*,#4073,.T.);
#6024=ORIENTED_EDGE('',*,*,#4074,.T.);
#6025=ORIENTED_EDGE('',*,*,#4075,.T.);
#6026=ORIENTED_EDGE('',*,*,#4068,.F.);
#6027=ORIENTED_EDGE('',*,*,#4076,.F.);
#6028=ORIENTED_EDGE('',*,*,#4077,.F.);
#6029=ORIENTED_EDGE('',*,*,#4078,.T.);
#6030=ORIENTED_EDGE('',*,*,#4079,.T.);
#6031=ORIENTED_EDGE('',*,*,#4080,.T.);
#6032=ORIENTED_EDGE('',*,*,#4073,.F.);
#6033=ORIENTED_EDGE('',*,*,#4081,.F.);
#6034=ORIENTED_EDGE('',*,*,#4082,.F.);
#6035=ORIENTED_EDGE('',*,*,#4083,.T.);
#6036=ORIENTED_EDGE('',*,*,#4084,.T.);
#6037=ORIENTED_EDGE('',*,*,#4085,.T.);
#6038=ORIENTED_EDGE('',*,*,#4078,.F.);
#6039=ORIENTED_EDGE('',*,*,#4086,.F.);
#6040=ORIENTED_EDGE('',*,*,#4087,.F.);
#6041=ORIENTED_EDGE('',*,*,#4088,.F.);
#6042=ORIENTED_EDGE('',*,*,#4089,.F.);
#6043=ORIENTED_EDGE('',*,*,#4090,.F.);
#6044=ORIENTED_EDGE('',*,*,#4091,.F.);
#6045=ORIENTED_EDGE('',*,*,#4092,.T.);
#6046=ORIENTED_EDGE('',*,*,#4093,.T.);
#6047=ORIENTED_EDGE('',*,*,#4094,.T.);
#6048=ORIENTED_EDGE('',*,*,#4095,.T.);
#6049=ORIENTED_EDGE('',*,*,#4096,.F.);
#6050=ORIENTED_EDGE('',*,*,#4097,.T.);
#6051=ORIENTED_EDGE('',*,*,#4098,.T.);
#6052=ORIENTED_EDGE('',*,*,#4099,.T.);
#6053=ORIENTED_EDGE('',*,*,#4100,.T.);
#6054=ORIENTED_EDGE('',*,*,#4094,.F.);
#6055=ORIENTED_EDGE('',*,*,#4101,.T.);
#6056=ORIENTED_EDGE('',*,*,#4102,.T.);
#6057=ORIENTED_EDGE('',*,*,#4103,.T.);
#6058=ORIENTED_EDGE('',*,*,#4104,.T.);
#6059=ORIENTED_EDGE('',*,*,#4098,.F.);
#6060=ORIENTED_EDGE('',*,*,#4105,.T.);
#6061=ORIENTED_EDGE('',*,*,#4106,.T.);
#6062=ORIENTED_EDGE('',*,*,#4107,.T.);
#6063=ORIENTED_EDGE('',*,*,#4108,.T.);
#6064=ORIENTED_EDGE('',*,*,#4109,.T.);
#6065=ORIENTED_EDGE('',*,*,#4102,.F.);
#6066=ORIENTED_EDGE('',*,*,#4110,.T.);
#6067=ORIENTED_EDGE('',*,*,#4111,.T.);
#6068=ORIENTED_EDGE('',*,*,#4112,.T.);
#6069=ORIENTED_EDGE('',*,*,#4113,.T.);
#6070=ORIENTED_EDGE('',*,*,#4107,.F.);
#6071=ORIENTED_EDGE('',*,*,#4114,.T.);
#6072=ORIENTED_EDGE('',*,*,#4115,.T.);
#6073=ORIENTED_EDGE('',*,*,#4116,.F.);
#6074=ORIENTED_EDGE('',*,*,#4117,.T.);
#6075=ORIENTED_EDGE('',*,*,#4118,.T.);
#6076=ORIENTED_EDGE('',*,*,#4119,.F.);
#6077=ORIENTED_EDGE('',*,*,#4120,.T.);
#6078=ORIENTED_EDGE('',*,*,#4121,.T.);
#6079=ORIENTED_EDGE('',*,*,#4122,.T.);
#6080=ORIENTED_EDGE('',*,*,#4123,.T.);
#6081=ORIENTED_EDGE('',*,*,#4124,.F.);
#6082=ORIENTED_EDGE('',*,*,#4125,.T.);
#6083=ORIENTED_EDGE('',*,*,#4126,.T.);
#6084=ORIENTED_EDGE('',*,*,#4127,.T.);
#6085=ORIENTED_EDGE('',*,*,#4128,.T.);
#6086=ORIENTED_EDGE('',*,*,#4122,.F.);
#6087=ORIENTED_EDGE('',*,*,#4129,.T.);
#6088=ORIENTED_EDGE('',*,*,#4130,.T.);
#6089=ORIENTED_EDGE('',*,*,#4131,.T.);
#6090=ORIENTED_EDGE('',*,*,#4132,.T.);
#6091=ORIENTED_EDGE('',*,*,#4126,.F.);
#6092=ORIENTED_EDGE('',*,*,#4133,.T.);
#6093=ORIENTED_EDGE('',*,*,#4134,.T.);
#6094=ORIENTED_EDGE('',*,*,#4135,.T.);
#6095=ORIENTED_EDGE('',*,*,#4136,.T.);
#6096=ORIENTED_EDGE('',*,*,#4137,.T.);
#6097=ORIENTED_EDGE('',*,*,#4130,.F.);
#6098=ORIENTED_EDGE('',*,*,#4138,.T.);
#6099=ORIENTED_EDGE('',*,*,#4139,.T.);
#6100=ORIENTED_EDGE('',*,*,#4140,.T.);
#6101=ORIENTED_EDGE('',*,*,#4141,.T.);
#6102=ORIENTED_EDGE('',*,*,#4135,.F.);
#6103=ORIENTED_EDGE('',*,*,#4142,.T.);
#6104=ORIENTED_EDGE('',*,*,#4143,.T.);
#6105=ORIENTED_EDGE('',*,*,#4144,.F.);
#6106=ORIENTED_EDGE('',*,*,#4145,.T.);
#6107=ORIENTED_EDGE('',*,*,#4146,.T.);
#6108=ORIENTED_EDGE('',*,*,#4147,.F.);
#6109=ORIENTED_EDGE('',*,*,#4148,.T.);
#6110=ORIENTED_EDGE('',*,*,#4149,.T.);
#6111=ORIENTED_EDGE('',*,*,#4144,.T.);
#6112=ORIENTED_EDGE('',*,*,#4150,.T.);
#6113=ORIENTED_EDGE('',*,*,#4151,.T.);
#6114=ORIENTED_EDGE('',*,*,#4139,.F.);
#6115=ORIENTED_EDGE('',*,*,#4152,.T.);
#6116=ORIENTED_EDGE('',*,*,#4153,.T.);
#6117=ORIENTED_EDGE('',*,*,#4116,.T.);
#6118=ORIENTED_EDGE('',*,*,#4154,.T.);
#6119=ORIENTED_EDGE('',*,*,#4155,.T.);
#6120=ORIENTED_EDGE('',*,*,#4111,.F.);
#6121=ORIENTED_EDGE('',*,*,#4156,.T.);
#6122=ORIENTED_EDGE('',*,*,#4157,.T.);
#6123=ORIENTED_EDGE('',*,*,#4088,.T.);
#6124=ORIENTED_EDGE('',*,*,#4158,.T.);
#6125=ORIENTED_EDGE('',*,*,#4159,.T.);
#6126=ORIENTED_EDGE('',*,*,#4083,.F.);
#6127=ORIENTED_EDGE('',*,*,#4160,.F.);
#6128=ORIENTED_EDGE('',*,*,#4161,.F.);
#6129=ORIENTED_EDGE('',*,*,#4058,.T.);
#6130=ORIENTED_EDGE('',*,*,#4162,.T.);
#6131=ORIENTED_EDGE('',*,*,#4163,.T.);
#6132=ORIENTED_EDGE('',*,*,#4053,.F.);
#6133=ORIENTED_EDGE('',*,*,#4164,.F.);
#6134=ORIENTED_EDGE('',*,*,#4165,.F.);
#6135=ORIENTED_EDGE('',*,*,#4166,.F.);
#6136=ORIENTED_EDGE('',*,*,#4035,.F.);
#6137=ORIENTED_EDGE('',*,*,#4040,.F.);
#6138=ORIENTED_EDGE('',*,*,#4039,.F.);
#6139=ORIENTED_EDGE('',*,*,#4045,.F.);
#6140=ORIENTED_EDGE('',*,*,#4044,.F.);
#6141=ORIENTED_EDGE('',*,*,#4050,.F.);
#6142=ORIENTED_EDGE('',*,*,#4049,.F.);
#6143=ORIENTED_EDGE('',*,*,#4055,.F.);
#6144=ORIENTED_EDGE('',*,*,#4054,.F.);
#6145=ORIENTED_EDGE('',*,*,#4163,.F.);
#6146=ORIENTED_EDGE('',*,*,#4162,.F.);
#6147=ORIENTED_EDGE('',*,*,#4063,.F.);
#6148=ORIENTED_EDGE('',*,*,#4062,.F.);
#6149=ORIENTED_EDGE('',*,*,#4167,.F.);
#6150=ORIENTED_EDGE('',*,*,#4146,.F.);
#6151=ORIENTED_EDGE('',*,*,#4145,.F.);
#6152=ORIENTED_EDGE('',*,*,#4153,.F.);
#6153=ORIENTED_EDGE('',*,*,#4152,.F.);
#6154=ORIENTED_EDGE('',*,*,#4143,.F.);
#6155=ORIENTED_EDGE('',*,*,#4142,.F.);
#6156=ORIENTED_EDGE('',*,*,#4138,.F.);
#6157=ORIENTED_EDGE('',*,*,#4134,.F.);
#6158=ORIENTED_EDGE('',*,*,#4133,.F.);
#6159=ORIENTED_EDGE('',*,*,#4129,.F.);
#6160=ORIENTED_EDGE('',*,*,#4125,.F.);
#6161=ORIENTED_EDGE('',*,*,#4168,.F.);
#6162=ORIENTED_EDGE('',*,*,#4169,.F.);
#6163=ORIENTED_EDGE('',*,*,#4123,.F.);
#6164=ORIENTED_EDGE('',*,*,#4128,.F.);
#6165=ORIENTED_EDGE('',*,*,#4127,.F.);
#6166=ORIENTED_EDGE('',*,*,#4132,.F.);
#6167=ORIENTED_EDGE('',*,*,#4131,.F.);
#6168=ORIENTED_EDGE('',*,*,#4137,.F.);
#6169=ORIENTED_EDGE('',*,*,#4136,.F.);
#6170=ORIENTED_EDGE('',*,*,#4141,.F.);
#6171=ORIENTED_EDGE('',*,*,#4140,.F.);
#6172=ORIENTED_EDGE('',*,*,#4151,.F.);
#6173=ORIENTED_EDGE('',*,*,#4150,.F.);
#6174=ORIENTED_EDGE('',*,*,#4149,.F.);
#6175=ORIENTED_EDGE('',*,*,#4148,.F.);
#6176=ORIENTED_EDGE('',*,*,#4170,.F.);
#6177=ORIENTED_EDGE('',*,*,#4060,.T.);
#6178=ORIENTED_EDGE('',*,*,#4059,.T.);
#6179=ORIENTED_EDGE('',*,*,#4165,.T.);
#6180=ORIENTED_EDGE('',*,*,#4164,.T.);
#6181=ORIENTED_EDGE('',*,*,#4057,.T.);
#6182=ORIENTED_EDGE('',*,*,#4056,.T.);
#6183=ORIENTED_EDGE('',*,*,#4052,.T.);
#6184=ORIENTED_EDGE('',*,*,#4051,.T.);
#6185=ORIENTED_EDGE('',*,*,#4047,.T.);
#6186=ORIENTED_EDGE('',*,*,#4046,.T.);
#6187=ORIENTED_EDGE('',*,*,#4042,.T.);
#6188=ORIENTED_EDGE('',*,*,#4041,.T.);
#6189=ORIENTED_EDGE('',*,*,#4037,.T.);
#6190=ORIENTED_EDGE('',*,*,#4171,.T.);
#6191=ORIENTED_EDGE('',*,*,#4172,.T.);
#6192=ORIENTED_EDGE('',*,*,#4173,.T.);
#6193=ORIENTED_EDGE('',*,*,#4174,.T.);
#6194=ORIENTED_EDGE('',*,*,#4175,.T.);
#6195=ORIENTED_EDGE('',*,*,#4091,.T.);
#6196=ORIENTED_EDGE('',*,*,#4176,.T.);
#6197=ORIENTED_EDGE('',*,*,#4119,.T.);
#6198=ORIENTED_EDGE('',*,*,#4167,.T.);
#6199=ORIENTED_EDGE('',*,*,#4061,.T.);
#6200=ORIENTED_EDGE('',*,*,#4170,.T.);
#6201=ORIENTED_EDGE('',*,*,#4147,.T.);
#6202=ORIENTED_EDGE('',*,*,#4177,.T.);
#6203=ORIENTED_EDGE('',*,*,#4178,.F.);
#6204=ORIENTED_EDGE('',*,*,#4065,.F.);
#6205=ORIENTED_EDGE('',*,*,#4070,.F.);
#6206=ORIENTED_EDGE('',*,*,#4069,.F.);
#6207=ORIENTED_EDGE('',*,*,#4075,.F.);
#6208=ORIENTED_EDGE('',*,*,#4074,.F.);
#6209=ORIENTED_EDGE('',*,*,#4080,.F.);
#6210=ORIENTED_EDGE('',*,*,#4079,.F.);
#6211=ORIENTED_EDGE('',*,*,#4085,.F.);
#6212=ORIENTED_EDGE('',*,*,#4084,.F.);
#6213=ORIENTED_EDGE('',*,*,#4159,.F.);
#6214=ORIENTED_EDGE('',*,*,#4158,.F.);
#6215=ORIENTED_EDGE('',*,*,#4093,.F.);
#6216=ORIENTED_EDGE('',*,*,#4092,.F.);
#6217=ORIENTED_EDGE('',*,*,#4175,.F.);
#6218=ORIENTED_EDGE('',*,*,#4118,.F.);
#6219=ORIENTED_EDGE('',*,*,#4117,.F.);
#6220=ORIENTED_EDGE('',*,*,#4157,.F.);
#6221=ORIENTED_EDGE('',*,*,#4156,.F.);
#6222=ORIENTED_EDGE('',*,*,#4115,.F.);
#6223=ORIENTED_EDGE('',*,*,#4114,.F.);
#6224=ORIENTED_EDGE('',*,*,#4110,.F.);
#6225=ORIENTED_EDGE('',*,*,#4106,.F.);
#6226=ORIENTED_EDGE('',*,*,#4105,.F.);
#6227=ORIENTED_EDGE('',*,*,#4101,.F.);
#6228=ORIENTED_EDGE('',*,*,#4097,.F.);
#6229=ORIENTED_EDGE('',*,*,#4179,.F.);
#6230=ORIENTED_EDGE('',*,*,#4180,.F.);
#6231=ORIENTED_EDGE('',*,*,#4095,.F.);
#6232=ORIENTED_EDGE('',*,*,#4100,.F.);
#6233=ORIENTED_EDGE('',*,*,#4099,.F.);
#6234=ORIENTED_EDGE('',*,*,#4104,.F.);
#6235=ORIENTED_EDGE('',*,*,#4103,.F.);
#6236=ORIENTED_EDGE('',*,*,#4109,.F.);
#6237=ORIENTED_EDGE('',*,*,#4108,.F.);
#6238=ORIENTED_EDGE('',*,*,#4113,.F.);
#6239=ORIENTED_EDGE('',*,*,#4112,.F.);
#6240=ORIENTED_EDGE('',*,*,#4155,.F.);
#6241=ORIENTED_EDGE('',*,*,#4154,.F.);
#6242=ORIENTED_EDGE('',*,*,#4121,.F.);
#6243=ORIENTED_EDGE('',*,*,#4120,.F.);
#6244=ORIENTED_EDGE('',*,*,#4176,.F.);
#6245=ORIENTED_EDGE('',*,*,#4090,.T.);
#6246=ORIENTED_EDGE('',*,*,#4089,.T.);
#6247=ORIENTED_EDGE('',*,*,#4161,.T.);
#6248=ORIENTED_EDGE('',*,*,#4160,.T.);
#6249=ORIENTED_EDGE('',*,*,#4087,.T.);
#6250=ORIENTED_EDGE('',*,*,#4086,.T.);
#6251=ORIENTED_EDGE('',*,*,#4082,.T.);
#6252=ORIENTED_EDGE('',*,*,#4081,.T.);
#6253=ORIENTED_EDGE('',*,*,#4077,.T.);
#6254=ORIENTED_EDGE('',*,*,#4076,.T.);
#6255=ORIENTED_EDGE('',*,*,#4072,.T.);
#6256=ORIENTED_EDGE('',*,*,#4071,.T.);
#6257=ORIENTED_EDGE('',*,*,#4067,.T.);
#6258=ORIENTED_EDGE('',*,*,#4177,.F.);
#6259=ORIENTED_EDGE('',*,*,#4181,.T.);
#6260=ORIENTED_EDGE('',*,*,#4182,.F.);
#6261=ORIENTED_EDGE('',*,*,#4181,.F.);
#6262=ORIENTED_EDGE('',*,*,#4183,.T.);
#6263=ORIENTED_EDGE('',*,*,#4184,.T.);
#6264=ORIENTED_EDGE('',*,*,#4174,.F.);
#6265=ORIENTED_EDGE('',*,*,#4185,.F.);
#6266=ORIENTED_EDGE('',*,*,#4186,.T.);
#6267=ORIENTED_EDGE('',*,*,#4185,.T.);
#6268=ORIENTED_EDGE('',*,*,#4173,.F.);
#6269=ORIENTED_EDGE('',*,*,#4187,.F.);
#6270=ORIENTED_EDGE('',*,*,#4188,.T.);
#6271=ORIENTED_EDGE('',*,*,#4187,.T.);
#6272=ORIENTED_EDGE('',*,*,#4172,.F.);
#6273=ORIENTED_EDGE('',*,*,#4189,.F.);
#6274=ORIENTED_EDGE('',*,*,#4190,.T.);
#6275=ORIENTED_EDGE('',*,*,#4189,.T.);
#6276=ORIENTED_EDGE('',*,*,#4171,.F.);
#6277=ORIENTED_EDGE('',*,*,#4184,.F.);
#6278=ORIENTED_EDGE('',*,*,#4190,.F.);
#6279=ORIENTED_EDGE('',*,*,#4183,.F.);
#6280=ORIENTED_EDGE('',*,*,#4186,.F.);
#6281=ORIENTED_EDGE('',*,*,#4188,.F.);
#6282=ORIENTED_EDGE('',*,*,#4166,.T.);
#6283=ORIENTED_EDGE('',*,*,#4168,.T.);
#6284=ORIENTED_EDGE('',*,*,#4124,.T.);
#6285=ORIENTED_EDGE('',*,*,#4169,.T.);
#6286=ORIENTED_EDGE('',*,*,#4036,.T.);
#6287=ORIENTED_EDGE('',*,*,#4178,.T.);
#6288=ORIENTED_EDGE('',*,*,#4179,.T.);
#6289=ORIENTED_EDGE('',*,*,#4096,.T.);
#6290=ORIENTED_EDGE('',*,*,#4180,.T.);
#6291=ORIENTED_EDGE('',*,*,#4066,.T.);
#6292=ORIENTED_EDGE('',*,*,#4182,.T.);
#6864=CYLINDRICAL_SURFACE('',#7584,3.0735);
#6865=CYLINDRICAL_SURFACE('',#7586,3.0735);
#6866=CYLINDRICAL_SURFACE('',#7587,3.0735);
#6867=CYLINDRICAL_SURFACE('',#7588,3.0735);
#6868=CYLINDRICAL_SURFACE('',#7589,3.0735);
#6869=CYLINDRICAL_SURFACE('',#7590,3.0735);
#6870=CYLINDRICAL_SURFACE('',#7592,3.0735);
#6871=CYLINDRICAL_SURFACE('',#7594,3.0735);
#6872=CYLINDRICAL_SURFACE('',#7595,3.0735);
#6873=CYLINDRICAL_SURFACE('',#7596,3.0735);
#6874=CYLINDRICAL_SURFACE('',#7597,3.0735);
#6875=CYLINDRICAL_SURFACE('',#7598,3.0735);
#6876=CYLINDRICAL_SURFACE('',#7600,2.5175);
#6877=CYLINDRICAL_SURFACE('',#7602,2.5175);
#6878=CYLINDRICAL_SURFACE('',#7603,2.5175);
#6879=CYLINDRICAL_SURFACE('',#7604,2.5175);
#6880=CYLINDRICAL_SURFACE('',#7605,2.5175);
#6881=CYLINDRICAL_SURFACE('',#7606,2.5175);
#6882=CYLINDRICAL_SURFACE('',#7608,2.5175);
#6883=CYLINDRICAL_SURFACE('',#7610,2.5175);
#6884=CYLINDRICAL_SURFACE('',#7611,2.5175);
#6885=CYLINDRICAL_SURFACE('',#7612,2.5175);
#6886=CYLINDRICAL_SURFACE('',#7613,2.5175);
#6887=CYLINDRICAL_SURFACE('',#7614,2.5175);
#6888=CYLINDRICAL_SURFACE('',#7616,2.5175);
#6889=CYLINDRICAL_SURFACE('',#7617,2.5175);
#6890=CYLINDRICAL_SURFACE('',#7618,3.0735);
#6891=CYLINDRICAL_SURFACE('',#7619,3.0735);
#6892=CYLINDRICAL_SURFACE('',#7622,11.);
#7100=ADVANCED_FACE('',(#1235),#6864,.F.);
#7101=ADVANCED_FACE('',(#1236),#6865,.F.);
#7102=ADVANCED_FACE('',(#1237),#6866,.F.);
#7103=ADVANCED_FACE('',(#1238),#6867,.F.);
#7104=ADVANCED_FACE('',(#1239),#6868,.F.);
#7105=ADVANCED_FACE('',(#1240),#6869,.F.);
#7106=ADVANCED_FACE('',(#1241),#6870,.F.);
#7107=ADVANCED_FACE('',(#1242),#6871,.F.);
#7108=ADVANCED_FACE('',(#1243),#6872,.F.);
#7109=ADVANCED_FACE('',(#1244),#6873,.F.);
#7110=ADVANCED_FACE('',(#1245),#6874,.F.);
#7111=ADVANCED_FACE('',(#1246),#6875,.F.);
#7112=ADVANCED_FACE('',(#1247),#6876,.F.);
#7113=ADVANCED_FACE('',(#1248),#6877,.F.);
#7114=ADVANCED_FACE('',(#1249),#6878,.F.);
#7115=ADVANCED_FACE('',(#1250),#6879,.F.);
#7116=ADVANCED_FACE('',(#1251),#6880,.F.);
#7117=ADVANCED_FACE('',(#1252),#6881,.F.);
#7118=ADVANCED_FACE('',(#1253),#6882,.F.);
#7119=ADVANCED_FACE('',(#1254),#6883,.F.);
#7120=ADVANCED_FACE('',(#1255),#6884,.F.);
#7121=ADVANCED_FACE('',(#1256),#6885,.F.);
#7122=ADVANCED_FACE('',(#1257),#6886,.F.);
#7123=ADVANCED_FACE('',(#1258),#6887,.F.);
#7124=ADVANCED_FACE('',(#1259),#6888,.F.);
#7125=ADVANCED_FACE('',(#1260),#6889,.F.);
#7126=ADVANCED_FACE('',(#1261),#6890,.F.);
#7127=ADVANCED_FACE('',(#1262),#6891,.F.);
#7128=ADVANCED_FACE('',(#1263),#99,.F.);
#7129=ADVANCED_FACE('',(#1264),#100,.F.);
#7130=ADVANCED_FACE('',(#1265,#983,#984,#985),#1036,.T.);
#7131=ADVANCED_FACE('',(#1266),#101,.F.);
#7132=ADVANCED_FACE('',(#1267),#102,.F.);
#7133=ADVANCED_FACE('',(#1268),#6892,.F.);
#7134=ADVANCED_FACE('',(#1269),#1037,.T.);
#7135=ADVANCED_FACE('',(#1270),#1038,.T.);
#7136=ADVANCED_FACE('',(#1271),#1039,.T.);
#7137=ADVANCED_FACE('',(#1272),#1040,.T.);
#7138=ADVANCED_FACE('',(#1273,#986,#987,#988),#1041,.F.);
#7208=CLOSED_SHELL('',(#7100,#7101,#7102,#7103,#7104,#7105,#7106,#7107,
#7108,#7109,#7110,#7111,#7112,#7113,#7114,#7115,#7116,#7117,#7118,#7119,
#7120,#7121,#7122,#7123,#7124,#7125,#7126,#7127,#7128,#7129,#7130,#7131,
#7132,#7133,#7134,#7135,#7136,#7137,#7138));
#7583=AXIS2_PLACEMENT_3D('',#79842,#8398,#8399);
#7584=AXIS2_PLACEMENT_3D('',#79843,#8400,#8401);
#7585=AXIS2_PLACEMENT_3D('',#79855,#8403,#8404);
#7586=AXIS2_PLACEMENT_3D('',#79950,#8405,#8406);
#7587=AXIS2_PLACEMENT_3D('',#80316,#8408,#8409);
#7588=AXIS2_PLACEMENT_3D('',#80618,#8411,#8412);
#7589=AXIS2_PLACEMENT_3D('',#80982,#8414,#8415);
#7590=AXIS2_PLACEMENT_3D('',#81287,#8417,#8418);
#7591=AXIS2_PLACEMENT_3D('',#81375,#8420,#8421);
#7592=AXIS2_PLACEMENT_3D('',#81448,#8422,#8423);
#7593=AXIS2_PLACEMENT_3D('',#81460,#8425,#8426);
#7594=AXIS2_PLACEMENT_3D('',#81555,#8427,#8428);
#7595=AXIS2_PLACEMENT_3D('',#81921,#8430,#8431);
#7596=AXIS2_PLACEMENT_3D('',#82223,#8433,#8434);
#7597=AXIS2_PLACEMENT_3D('',#82587,#8436,#8437);
#7598=AXIS2_PLACEMENT_3D('',#82892,#8439,#8440);
#7599=AXIS2_PLACEMENT_3D('',#82980,#8442,#8443);
#7600=AXIS2_PLACEMENT_3D('',#83053,#8444,#8445);
#7601=AXIS2_PLACEMENT_3D('',#83069,#8447,#8448);
#7602=AXIS2_PLACEMENT_3D('',#83126,#8449,#8450);
#7603=AXIS2_PLACEMENT_3D('',#83478,#8452,#8453);
#7604=AXIS2_PLACEMENT_3D('',#83844,#8455,#8456);
#7605=AXIS2_PLACEMENT_3D('',#84032,#8458,#8459);
#7606=AXIS2_PLACEMENT_3D('',#84243,#8461,#8462);
#7607=AXIS2_PLACEMENT_3D('',#84381,#8464,#8465);
#7608=AXIS2_PLACEMENT_3D('',#84568,#8466,#8467);
#7609=AXIS2_PLACEMENT_3D('',#84584,#8469,#8470);
#7610=AXIS2_PLACEMENT_3D('',#84641,#8471,#8472);
#7611=AXIS2_PLACEMENT_3D('',#84993,#8474,#8475);
#7612=AXIS2_PLACEMENT_3D('',#85361,#8477,#8478);
#7613=AXIS2_PLACEMENT_3D('',#85549,#8480,#8481);
#7614=AXIS2_PLACEMENT_3D('',#85760,#8483,#8484);
#7615=AXIS2_PLACEMENT_3D('',#85898,#8486,#8487);
#7616=AXIS2_PLACEMENT_3D('',#86085,#8488,#8489);
#7617=AXIS2_PLACEMENT_3D('',#86470,#8490,#8491);
#7618=AXIS2_PLACEMENT_3D('',#86855,#8492,#8493);
#7619=AXIS2_PLACEMENT_3D('',#87084,#8494,#8495);
#7620=AXIS2_PLACEMENT_3D('',#88020,#8496,#8497);
#7621=AXIS2_PLACEMENT_3D('',#88212,#8502,#8503);
#7622=AXIS2_PLACEMENT_3D('',#88744,#8504,#8505);
#7623=AXIS2_PLACEMENT_3D('',#88747,#8507,#8508);
#7624=AXIS2_PLACEMENT_3D('',#88748,#8509,#8510);
#7625=AXIS2_PLACEMENT_3D('',#88754,#8514,#8515);
#7626=AXIS2_PLACEMENT_3D('',#88758,#8518,#8519);
#7627=AXIS2_PLACEMENT_3D('',#88762,#8522,#8523);
#7628=AXIS2_PLACEMENT_3D('',#88764,#8525,#8526);
#8398=DIRECTION('axis',(0.,0.,1.));
#8399=DIRECTION('refdir',(1.,0.,0.));
#8400=DIRECTION('center_axis',(0.,0.,-1.));
#8401=DIRECTION('ref_axis',(-0.609178726672388,-0.793032962095402,0.));
#8402=DIRECTION('',(0.,0.,-1.));
#8403=DIRECTION('center_axis',(0.,0.,1.));
#8404=DIRECTION('ref_axis',(1.,-7.46332589967923E-15,0.));
#8405=DIRECTION('center_axis',(0.,0.,-1.));
#8406=DIRECTION('ref_axis',(-0.609178726672388,-0.793032962095402,0.));
#8407=DIRECTION('',(0.,0.,-1.));
#8408=DIRECTION('center_axis',(0.,0.,-1.));
#8409=DIRECTION('ref_axis',(-0.609178726672388,-0.793032962095402,0.));
#8410=DIRECTION('',(0.,0.,-1.));
#8411=DIRECTION('center_axis',(0.,0.,-1.));
#8412=DIRECTION('ref_axis',(-0.609178726672388,-0.793032962095402,0.));
#8413=DIRECTION('',(0.,0.,-1.));
#8414=DIRECTION('center_axis',(0.,0.,-1.));
#8415=DIRECTION('ref_axis',(-0.609178726672388,-0.793032962095402,0.));
#8416=DIRECTION('',(0.,0.,-1.));
#8417=DIRECTION('center_axis',(0.,0.,-1.));
#8418=DIRECTION('ref_axis',(-0.609178726672388,-0.793032962095402,0.));
#8419=DIRECTION('',(0.,0.,-1.));
#8420=DIRECTION('center_axis',(0.,0.,-1.));
#8421=DIRECTION('ref_axis',(1.,-7.46332589967923E-15,0.));
#8422=DIRECTION('center_axis',(0.,0.,-1.));
#8423=DIRECTION('ref_axis',(-0.609178844542212,-0.793032871552129,0.));
#8424=DIRECTION('',(0.,0.,-1.));
#8425=DIRECTION('center_axis',(0.,0.,1.));
#8426=DIRECTION('ref_axis',(1.,-7.50489341657914E-15,0.));
#8427=DIRECTION('center_axis',(0.,0.,-1.));
#8428=DIRECTION('ref_axis',(-0.609178844542212,-0.793032871552129,0.));
#8429=DIRECTION('',(0.,0.,-1.));
#8430=DIRECTION('center_axis',(0.,0.,-1.));
#8431=DIRECTION('ref_axis',(-0.609178844542212,-0.793032871552129,0.));
#8432=DIRECTION('',(0.,0.,-1.));
#8433=DIRECTION('center_axis',(0.,0.,-1.));
#8434=DIRECTION('ref_axis',(-0.609178844542212,-0.793032871552129,0.));
#8435=DIRECTION('',(0.,0.,-1.));
#8436=DIRECTION('center_axis',(0.,0.,-1.));
#8437=DIRECTION('ref_axis',(-0.609178844542212,-0.793032871552129,0.));
#8438=DIRECTION('',(0.,0.,-1.));
#8439=DIRECTION('center_axis',(0.,0.,-1.));
#8440=DIRECTION('ref_axis',(-0.609178844542212,-0.793032871552129,0.));
#8441=DIRECTION('',(0.,0.,-1.));
#8442=DIRECTION('center_axis',(0.,0.,-1.));
#8443=DIRECTION('ref_axis',(1.,-7.50489341657914E-15,0.));
#8444=DIRECTION('center_axis',(0.,0.,-1.));
#8445=DIRECTION('ref_axis',(0.938005636158359,-0.34662000307996,0.));
#8446=DIRECTION('',(0.,0.,-1.));
#8447=DIRECTION('center_axis',(0.,0.,-1.));
#8448=DIRECTION('ref_axis',(1.,0.,0.));
#8449=DIRECTION('center_axis',(0.,0.,-1.));
#8450=DIRECTION('ref_axis',(0.938005636158359,-0.34662000307996,0.));
#8451=DIRECTION('',(0.,0.,-1.));
#8452=DIRECTION('center_axis',(0.,0.,-1.));
#8453=DIRECTION('ref_axis',(0.938005636158359,-0.34662000307996,0.));
#8454=DIRECTION('',(0.,0.,-1.));
#8455=DIRECTION('center_axis',(0.,0.,-1.));
#8456=DIRECTION('ref_axis',(0.938005636158359,-0.34662000307996,0.));
#8457=DIRECTION('',(0.,0.,-1.));
#8458=DIRECTION('center_axis',(0.,0.,-1.));
#8459=DIRECTION('ref_axis',(0.938005636158359,-0.34662000307996,0.));
#8460=DIRECTION('',(0.,0.,-1.));
#8461=DIRECTION('center_axis',(0.,0.,-1.));
#8462=DIRECTION('ref_axis',(0.938005636158359,-0.34662000307996,0.));
#8463=DIRECTION('',(0.,0.,-1.));
#8464=DIRECTION('center_axis',(0.,0.,-1.));
#8465=DIRECTION('ref_axis',(1.,0.,0.));
#8466=DIRECTION('center_axis',(0.,0.,-1.));
#8467=DIRECTION('ref_axis',(0.938005556308566,-0.346620219165381,0.));
#8468=DIRECTION('',(0.,0.,-1.));
#8469=DIRECTION('center_axis',(0.,0.,-1.));
#8470=DIRECTION('ref_axis',(1.,0.,0.));
#8471=DIRECTION('center_axis',(0.,0.,-1.));
#8472=DIRECTION('ref_axis',(0.938005556308566,-0.346620219165381,0.));
#8473=DIRECTION('',(0.,0.,-1.));
#8474=DIRECTION('center_axis',(0.,0.,-1.));
#8475=DIRECTION('ref_axis',(0.938005556308566,-0.346620219165381,0.));
#8476=DIRECTION('',(0.,0.,-1.));
#8477=DIRECTION('center_axis',(0.,0.,-1.));
#8478=DIRECTION('ref_axis',(0.938005556308566,-0.346620219165381,0.));
#8479=DIRECTION('',(0.,0.,-1.));
#8480=DIRECTION('center_axis',(0.,0.,-1.));
#8481=DIRECTION('ref_axis',(0.938005556308566,-0.346620219165381,0.));
#8482=DIRECTION('',(0.,0.,-1.));
#8483=DIRECTION('center_axis',(0.,0.,-1.));
#8484=DIRECTION('ref_axis',(0.938005556308566,-0.346620219165381,0.));
#8485=DIRECTION('',(0.,0.,-1.));
#8486=DIRECTION('center_axis',(0.,0.,-1.));
#8487=DIRECTION('ref_axis',(1.,0.,0.));
#8488=DIRECTION('center_axis',(0.,0.,-1.));
#8489=DIRECTION('ref_axis',(0.938005556308566,-0.346620219165381,0.));
#8490=DIRECTION('center_axis',(0.,0.,-1.));
#8491=DIRECTION('ref_axis',(0.938005636158359,-0.34662000307996,0.));
#8492=DIRECTION('center_axis',(0.,0.,-1.));
#8493=DIRECTION('ref_axis',(-0.609178844542212,-0.793032871552129,0.));
#8494=DIRECTION('center_axis',(0.,0.,-1.));
#8495=DIRECTION('ref_axis',(-0.609178726672388,-0.793032962095402,0.));
#8496=DIRECTION('center_axis',(0.,0.,1.));
#8497=DIRECTION('ref_axis',(1.,0.,0.));
#8498=DIRECTION('',(0.,-1.,0.));
#8499=DIRECTION('',(1.,0.,0.));
#8500=DIRECTION('',(0.,1.,0.));
#8501=DIRECTION('',(-1.,0.,0.));
#8502=DIRECTION('center_axis',(0.,0.,-1.));
#8503=DIRECTION('ref_axis',(1.,0.,0.));
#8504=DIRECTION('center_axis',(0.,0.,-1.));
#8505=DIRECTION('ref_axis',(1.,0.,0.));
#8506=DIRECTION('',(0.,0.,-1.));
#8507=DIRECTION('center_axis',(0.,0.,1.));
#8508=DIRECTION('ref_axis',(1.,0.,0.));
#8509=DIRECTION('center_axis',(0.,1.,0.));
#8510=DIRECTION('ref_axis',(-1.,0.,0.));
#8511=DIRECTION('',(-1.,0.,0.));
#8512=DIRECTION('',(0.,0.,1.));
#8513=DIRECTION('',(0.,0.,1.));
#8514=DIRECTION('center_axis',(1.,0.,0.));
#8515=DIRECTION('ref_axis',(0.,1.,0.));
#8516=DIRECTION('',(0.,1.,0.));
#8517=DIRECTION('',(0.,0.,1.));
#8518=DIRECTION('center_axis',(0.,-1.,0.));
#8519=DIRECTION('ref_axis',(1.,0.,0.));
#8520=DIRECTION('',(1.,0.,0.));
#8521=DIRECTION('',(0.,0.,1.));
#8522=DIRECTION('center_axis',(-1.,0.,0.));
#8523=DIRECTION('ref_axis',(0.,-1.,0.));
#8524=DIRECTION('',(0.,-1.,0.));
#8525=DIRECTION('center_axis',(0.,0.,1.));
#8526=DIRECTION('ref_axis',(1.,0.,0.));
#79842=CARTESIAN_POINT('',(0.,0.,0.));
#79843=CARTESIAN_POINT('Origin',(15.,0.,8.20842344717745));
#79844=CARTESIAN_POINT('',(16.8723108164276,2.43738680900022,0.437234123991138));
#79845=CARTESIAN_POINT('',(16.8725886476928,2.43775122616105,0.354313353567125));
#79846=CARTESIAN_POINT('',(16.8723108164276,2.43738680900022,8.20842344717745));
#79847=CARTESIAN_POINT('',(15.7937992825328,-2.9692229537457,0.));
#79848=CARTESIAN_POINT('Ctrl Pts',(16.8725886476925,2.43775122616123,0.354313353567141));
#79849=CARTESIAN_POINT('Ctrl Pts',(17.0693981870995,2.2896606486941,0.341559014872585));
#79850=CARTESIAN_POINT('Ctrl Pts',(17.9852366821766,1.41166315331641,0.276129619930782));
#79851=CARTESIAN_POINT('Ctrl Pts',(18.4440669366553,-1.13346924859543,0.158025168741733));
#79852=CARTESIAN_POINT('Ctrl Pts',(16.7765145099754,-2.70650147589442,0.052675056247244));
#79853=CARTESIAN_POINT('Ctrl Pts',(15.7937992825328,-2.9692229537457,-1.11022302462516E-15));
#79854=CARTESIAN_POINT('',(14.2061995950377,-2.96922265367245,2.23034764090801E-5));
#79855=CARTESIAN_POINT('Origin',(15.,0.,0.));
#79856=CARTESIAN_POINT('Ctrl Pts',(16.8723108164276,2.43738680900022,0.437234123991137));
#79857=CARTESIAN_POINT('Ctrl Pts',(16.9486000539327,2.37878422526983,0.432252120409439));
#79858=CARTESIAN_POINT('Ctrl Pts',(17.0222149233757,2.3165352990722,0.427270116827742));
#79859=CARTESIAN_POINT('Ctrl Pts',(17.0927910606528,2.25091710785889,0.422288113246044));
#79860=CARTESIAN_POINT('Ctrl Pts',(17.1633209527764,2.18534191309508,0.417309374132041));
#79861=CARTESIAN_POINT('Ctrl Pts',(17.2308157490115,2.11640214016536,0.412330635018037));
#79862=CARTESIAN_POINT('Ctrl Pts',(17.2949445180178,2.0444148085015,0.407351895904035));
#79863=CARTESIAN_POINT('Ctrl Pts',(17.3590525920387,1.97245070785851,0.402374763478175));
#79864=CARTESIAN_POINT('Ctrl Pts',(17.4197965046981,1.89744133072467,0.397397631052316));
#79865=CARTESIAN_POINT('Ctrl Pts',(17.4768832401704,1.81973944963634,0.392420498626455));
#79866=CARTESIAN_POINT('Ctrl Pts',(17.5339672179588,1.74204132208603,0.387443606630499));
#79867=CARTESIAN_POINT('Ctrl Pts',(17.5873941096951,1.66165130397085,0.382466714634545));
#79868=CARTESIAN_POINT('Ctrl Pts',(17.6369128106088,1.57895315929483,0.377489822638589));
#79869=CARTESIAN_POINT('Ctrl Pts',(17.6864427073912,1.49623631708526,0.372511805398464));
#79870=CARTESIAN_POINT('Ctrl Pts',(17.7320624324359,1.4112106892341,0.367533788158336));
#79871=CARTESIAN_POINT('Ctrl Pts',(17.7735661748459,1.32428581648768,0.362555770918211));
#79872=CARTESIAN_POINT('Ctrl Pts',(17.8151160151883,1.23726439685972,0.357572224627246));
#79873=CARTESIAN_POINT('Ctrl Pts',(17.8525405583626,1.14833991940812,0.35258867833628));
#79874=CARTESIAN_POINT('Ctrl Pts',(17.8856817322189,1.05794290504634,0.347605132045315));
#79875=CARTESIAN_POINT('Ctrl Pts',(17.9188438701762,0.967488708276125,0.342618433314177));
#79876=CARTESIAN_POINT('Ctrl Pts',(17.9477171132732,0.875560539500225,0.337631734583041));
#79877=CARTESIAN_POINT('Ctrl Pts',(17.9721935807742,0.782603072064333,0.332645035851904));
#79878=CARTESIAN_POINT('Ctrl Pts',(17.9967089243288,0.689497959978504,0.327650416730842));
#79879=CARTESIAN_POINT('Ctrl Pts',(18.0168134609883,0.595360715303609,0.32265579760978));
#79880=CARTESIAN_POINT('Ctrl Pts',(18.0324506333514,0.500644990274309,0.317661178488717));
#79881=CARTESIAN_POINT('Ctrl Pts',(18.0393042270298,0.459132172020722,0.31547209409165));
#79882=CARTESIAN_POINT('Ctrl Pts',(18.0453003284032,0.417508278592077,0.313283009694582));
#79883=CARTESIAN_POINT('Ctrl Pts',(18.0504373294725,0.375811587049335,0.311093925297515));
#79884=CARTESIAN_POINT('Ctrl Pts',(18.0621939245159,0.280384097254954,0.306083963565994));
#79885=CARTESIAN_POINT('Ctrl Pts',(18.0694885112601,0.184240555982924,0.301074001834474));
#79886=CARTESIAN_POINT('Ctrl Pts',(18.0722447249927,0.0878327943001572,
0.296064040102953));
#79887=CARTESIAN_POINT('Ctrl Pts',(18.0749972100634,-0.00844454500551578,
0.291060855949365));
#79888=CARTESIAN_POINT('Ctrl Pts',(18.0732235131107,-0.104984961100177,
0.286057671795777));
#79889=CARTESIAN_POINT('Ctrl Pts',(18.0668988426675,-0.201329925357491,
0.281054487642189));
#79890=CARTESIAN_POINT('Ctrl Pts',(18.0605808432663,-0.297573268304245,
0.276056580672879));
#79891=CARTESIAN_POINT('Ctrl Pts',(18.0497214423724,-0.393621135526973,
0.27105867370357));
#79892=CARTESIAN_POINT('Ctrl Pts',(18.034347895094,-0.489014418538606,0.26606076673426));
#79893=CARTESIAN_POINT('Ctrl Pts',(18.0189855206538,-0.584338373782033,
0.261066492030504));
#79894=CARTESIAN_POINT('Ctrl Pts',(17.9991155921472,-0.679008260532783,
0.256072217326748));
#79895=CARTESIAN_POINT('Ctrl Pts',(17.9748171546814,-0.772570479770897,
0.251077942622992));
#79896=CARTESIAN_POINT('Ctrl Pts',(17.9505277471661,-0.86609792878083,0.246085523925564));
#79897=CARTESIAN_POINT('Ctrl Pts',(17.9218132108177,-0.958518105804558,
0.241093105228137));
#79898=CARTESIAN_POINT('Ctrl Pts',(17.888803417088,-1.04938890189513,0.236100686530709));
#79899=CARTESIAN_POINT('Ctrl Pts',(17.8557969816939,-1.14025045301321,0.231108775749746));
#79900=CARTESIAN_POINT('Ctrl Pts',(17.8184963072286,-1.22956252603547,0.226116864968781));
#79901=CARTESIAN_POINT('Ctrl Pts',(17.7770803885989,-1.3169004386282,0.221124954187818));
#79902=CARTESIAN_POINT('Ctrl Pts',(17.7356575060978,-1.40425303663708,0.216132204042997));
#79903=CARTESIAN_POINT('Ctrl Pts',(17.6901181924538,-1.48963042019004,0.211139453898177));
#79904=CARTESIAN_POINT('Ctrl Pts',(17.6406881541377,-1.57263101921493,0.206146703753356));
#79905=CARTESIAN_POINT('Ctrl Pts',(17.5912068526544,-1.65571769694263,0.201148775700653));
#79906=CARTESIAN_POINT('Ctrl Pts',(17.5378269948197,-1.73642229307496,0.19615084764795));
#79907=CARTESIAN_POINT('Ctrl Pts',(17.4808184105717,-1.81437103806483,0.191152919595247));
#79908=CARTESIAN_POINT('Ctrl Pts',(17.4237770906029,-1.89236454312705,0.186152121610241));
#79909=CARTESIAN_POINT('Ctrl Pts',(17.3631031686193,-1.96759870545471,0.181151323625236));
#79910=CARTESIAN_POINT('Ctrl Pts',(17.299106357257,-2.03973336689388,0.17615052564023));
#79911=CARTESIAN_POINT('Ctrl Pts',(17.2350100731102,-2.11198015010117,0.171141954716378));
#79912=CARTESIAN_POINT('Ctrl Pts',(17.1675808912483,-2.18111749990926,0.166133383792525));
#79913=CARTESIAN_POINT('Ctrl Pts',(17.0971648279345,-2.24684265903837,0.161124812868673));
#79914=CARTESIAN_POINT('Ctrl Pts',(17.0594111599379,-2.28208129238432,0.158439460764373));
#79915=CARTESIAN_POINT('Ctrl Pts',(17.0207994536887,-2.3163397556618,0.155754108660072));
#79916=CARTESIAN_POINT('Ctrl Pts',(16.9813866277332,-2.34957640468239,0.153068756555772));
#79917=CARTESIAN_POINT('Ctrl Pts',(16.9083021280413,-2.41120821631254,0.14808921981155));
#79918=CARTESIAN_POINT('Ctrl Pts',(16.8322081567229,-2.46953728502221,0.14310968306733));
#79919=CARTESIAN_POINT('Ctrl Pts',(16.7534369591403,-2.52425455933447,0.138130146323109));
#79920=CARTESIAN_POINT('Ctrl Pts',(16.6747707605681,-2.57889889760119,0.133157247111975));
#79921=CARTESIAN_POINT('Ctrl Pts',(16.5934347875804,-2.62994075769122,0.128184347900842));
#79922=CARTESIAN_POINT('Ctrl Pts',(16.5097952239559,-2.67711050046874,0.123211448689709));
#79923=CARTESIAN_POINT('Ctrl Pts',(16.4234649138133,-2.72579772869974,0.118078567639155));
#79924=CARTESIAN_POINT('Ctrl Pts',(16.3346806322611,-2.77035914660608,0.112945686588602));
#79925=CARTESIAN_POINT('Ctrl Pts',(16.2438787989889,-2.81054581592722,0.107812805538048));
#79926=CARTESIAN_POINT('Ctrl Pts',(16.1560574750195,-2.84941338476941,0.102848407866847));
#79927=CARTESIAN_POINT('Ctrl Pts',(16.066349421105,-2.88418872496296,0.097884010195645));
#79928=CARTESIAN_POINT('Ctrl Pts',(15.9751742796223,-2.91469335854789,0.0929196125244438));
#79929=CARTESIAN_POINT('Ctrl Pts',(15.884027995866,-2.94518833715058,0.0879567861283488));
#79930=CARTESIAN_POINT('Ctrl Pts',(15.7914159666675,-2.97141515424664,0.0829939597322541));
#79931=CARTESIAN_POINT('Ctrl Pts',(15.6977757461357,-2.99324426970216,0.0780311333361592));
#79932=CARTESIAN_POINT('Ctrl Pts',(15.6041390697955,-3.0150725589468,0.0730684947782371));
#79933=CARTESIAN_POINT('Ctrl Pts',(15.5094747109312,-3.0325033776651,0.0681058562203135));
#79934=CARTESIAN_POINT('Ctrl Pts',(15.4142321453266,-3.0454579261218,0.0631432176623914));
#79935=CARTESIAN_POINT('Ctrl Pts',(15.3189666441661,-3.05841559418966,0.0581793840413839));
#79936=CARTESIAN_POINT('Ctrl Pts',(15.2231230984729,-3.0668947920386,0.0532155504203748));
#79937=CARTESIAN_POINT('Ctrl Pts',(15.1271567394664,-3.07086851128606,0.048251716799367));
#79938=CARTESIAN_POINT('Ctrl Pts',(15.0310858171913,-3.07484656022861,0.0432824746719422));
#79939=CARTESIAN_POINT('Ctrl Pts',(14.9348922574478,-3.0743093170539,0.0383132325445207));
#79940=CARTESIAN_POINT('Ctrl Pts',(14.8390315762507,-3.06928190568342,0.0333439904170962));
#79941=CARTESIAN_POINT('Ctrl Pts',(14.7431081497739,-3.0642512036381,0.028371495689299));
#79942=CARTESIAN_POINT('Ctrl Pts',(14.6475184752423,-3.05472452826285,0.023399000961501));
#79943=CARTESIAN_POINT('Ctrl Pts',(14.5527111342476,-3.04077867010638,0.0184265062337037));
#79944=CARTESIAN_POINT('Ctrl Pts',(14.4577618030923,-3.02681192564914,0.013446564347092));
#79945=CARTESIAN_POINT('Ctrl Pts',(14.3635975760094,-3.00841287909547,0.00846662246047965));
#79946=CARTESIAN_POINT('Ctrl Pts',(14.2706547108404,-2.98570891065769,0.00348668057386803));
#79947=CARTESIAN_POINT('Ctrl Pts',(14.2491023085036,-2.98044411640452,0.00233188820804814));
#79948=CARTESIAN_POINT('Ctrl Pts',(14.2276155056363,-2.97494804394752,0.00117709584222782));
#79949=CARTESIAN_POINT('Ctrl Pts',(14.2061995950377,-2.96922265367245,2.23034764079699E-5));
#79950=CARTESIAN_POINT('Origin',(15.,0.,8.20842344717745));
#79951=CARTESIAN_POINT('',(16.8723108164276,2.43738680900023,1.43740555432678));
#79952=CARTESIAN_POINT('',(16.8723108164276,2.43738680900022,1.35414036795513));
#79953=CARTESIAN_POINT('',(16.8723108164276,2.43738680900022,8.20842344717745));
#79954=CARTESIAN_POINT('',(11.9270323372931,0.000383793694356834,0.708423426365591));
#79955=CARTESIAN_POINT('Ctrl Pts',(16.8723108164276,2.43738680900022,1.35414036795513));
#79956=CARTESIAN_POINT('Ctrl Pts',(16.9488467645666,2.37859471124328,1.34915700951272));
#79957=CARTESIAN_POINT('Ctrl Pts',(17.0226289554853,2.31618034982088,1.34417365107031));
#79958=CARTESIAN_POINT('Ctrl Pts',(17.0933051804222,2.25043899531123,1.3391902926279));
#79959=CARTESIAN_POINT('Ctrl Pts',(17.163985736743,2.18469361185065,1.33420662878097));
#79960=CARTESIAN_POINT('Ctrl Pts',(17.2315596282501,2.11562112957336,1.32922296493404));
#79961=CARTESIAN_POINT('Ctrl Pts',(17.2957104120883,2.04355473472801,1.32423930108711));
#79962=CARTESIAN_POINT('Ctrl Pts',(17.3601121879841,1.97120637773592,1.31923613849101));
#79963=CARTESIAN_POINT('Ctrl Pts',(17.4210637143198,1.89584096046158,1.31423297589491));
#79964=CARTESIAN_POINT('Ctrl Pts',(17.4782856482745,1.81782906114865,1.3092298132988));
#79965=CARTESIAN_POINT('Ctrl Pts',(17.535369363359,1.74000559860883,1.30423873577976));
#79966=CARTESIAN_POINT('Ctrl Pts',(17.5887412740794,1.65954881494975,1.29924765826073));
#79967=CARTESIAN_POINT('Ctrl Pts',(17.6381683823442,1.57685441192242,1.29425658074169));
#79968=CARTESIAN_POINT('Ctrl Pts',(17.6877750100846,1.49385966245803,1.28924737560705));
#79969=CARTESIAN_POINT('Ctrl Pts',(17.7334079269677,1.40861140609851,1.28423817047242));
#79970=CARTESIAN_POINT('Ctrl Pts',(17.7748794341556,1.32153182931781,1.27922896533778));
#79971=CARTESIAN_POINT('Ctrl Pts',(17.8163509413436,1.2344522525371,1.27421976020315));
#79972=CARTESIAN_POINT('Ctrl Pts',(17.8536609240355,1.14554178452447,1.26921055506852));
#79973=CARTESIAN_POINT('Ctrl Pts',(17.8866717782577,1.05523850129278,1.26420134993389));
#79974=CARTESIAN_POINT('Ctrl Pts',(17.9196220614258,0.965100914017152,1.25920133610442));
#79975=CARTESIAN_POINT('Ctrl Pts',(17.9484040181812,0.873260955603744,1.25420132227496));
#79976=CARTESIAN_POINT('Ctrl Pts',(17.9728410642138,0.78013989573926,1.24920130844549));
#79977=CARTESIAN_POINT('Ctrl Pts',(17.9972450936874,0.687144650466591,1.2442080500664));
#79978=CARTESIAN_POINT('Ctrl Pts',(18.0173157690538,0.592872164657343,1.23921479168731));
#79979=CARTESIAN_POINT('Ctrl Pts',(18.0329252006786,0.49776196830291,1.23422153330823));
#79980=CARTESIAN_POINT('Ctrl Pts',(18.0485182458185,0.402751616826001,1.22923351675694));
#79981=CARTESIAN_POINT('Ctrl Pts',(18.0596592868045,0.306905733810672,1.22424550020565));
#79982=CARTESIAN_POINT('Ctrl Pts',(18.0662709882578,0.210676236363457,1.21925748365436));
#79983=CARTESIAN_POINT('Ctrl Pts',(18.0728779987174,0.114515013622831,1.2142730060945));
#79984=CARTESIAN_POINT('Ctrl Pts',(18.0749620280716,0.0179711540885037,
1.20928852853464));
#79985=CARTESIAN_POINT('Ctrl Pts',(18.0724974312295,-0.0784970387206864,
1.20430405097478));
#79986=CARTESIAN_POINT('Ctrl Pts',(18.0700337215717,-0.174930505744737,
1.19932136768401));
#79987=CARTESIAN_POINT('Ctrl Pts',(18.0630246502553,-0.271287921906674,
1.19433868439324));
#79988=CARTESIAN_POINT('Ctrl Pts',(18.0514966819704,-0.367110678029874,
1.18935600110248));
#79989=CARTESIAN_POINT('Ctrl Pts',(18.0399697184903,-0.462925082017096,
1.18437375211406));
#79990=CARTESIAN_POINT('Ctrl Pts',(18.0239246937907,-0.558204482949211,
1.17939150312564));
#79991=CARTESIAN_POINT('Ctrl Pts',(18.0034398632507,-0.652496159250288,
1.17440925413723));
#79992=CARTESIAN_POINT('Ctrl Pts',(17.9829512298507,-0.746805340116538,
1.16942608023046));
#79993=CARTESIAN_POINT('Ctrl Pts',(17.9580212468915,-0.840126003369507,
1.16444290632369));
#79994=CARTESIAN_POINT('Ctrl Pts',(17.9287788876878,-0.932017423138756,
1.15945973241692));
#79995=CARTESIAN_POINT('Ctrl Pts',(17.8995050420624,-1.02400778608743,1.15447119292682));
#79996=CARTESIAN_POINT('Ctrl Pts',(17.8659096838051,-1.11456541446941,1.14948265343671));
#79997=CARTESIAN_POINT('Ctrl Pts',(17.8281710387483,-1.20326673085614,1.14449411394661));
#79998=CARTESIAN_POINT('Ctrl Pts',(17.7904099793551,-1.29202073013984,1.13950261158378));
#79999=CARTESIAN_POINT('Ctrl Pts',(17.7485009237813,-1.37891582706822,1.13451110922094));
#80000=CARTESIAN_POINT('Ctrl Pts',(17.7026685033149,-1.46355225775839,1.12951960685811));
#80001=CARTESIAN_POINT('Ctrl Pts',(17.6567625502343,-1.54832447743685,1.1245200962292));
#80002=CARTESIAN_POINT('Ctrl Pts',(17.606920890662,-1.63083042003146,1.1195205856003));
#80003=CARTESIAN_POINT('Ctrl Pts',(17.5534119272192,-1.71069862335089,1.1145210749714));
#80004=CARTESIAN_POINT('Ctrl Pts',(17.5236405722932,-1.75513575080276,1.11173944371165));
#80005=CARTESIAN_POINT('Ctrl Pts',(17.4927347077816,-1.79875691118914,1.10895781245189));
#80006=CARTESIAN_POINT('Ctrl Pts',(17.4607457862635,-1.84150276279636,1.10617618119214));
#80007=CARTESIAN_POINT('Ctrl Pts',(17.4032237856212,-1.91836771437699,1.10117429342861));
#80008=CARTESIAN_POINT('Ctrl Pts',(17.3419966626954,-1.99266879379093,1.09617240566508));
#80009=CARTESIAN_POINT('Ctrl Pts',(17.2773210991351,-2.06402782477227,1.09117051790155));
#80010=CARTESIAN_POINT('Ctrl Pts',(17.2127329198155,-2.13529044136784,1.08617538827261));
#80011=CARTESIAN_POINT('Ctrl Pts',(17.1447058520614,-2.20361858776218,1.08118025864368));
#80012=CARTESIAN_POINT('Ctrl Pts',(17.0735384616154,-2.26866491536356,1.07618512901475));
#80013=CARTESIAN_POINT('Ctrl Pts',(17.0024458265917,-2.3336429172099,1.07119524635388));
#80014=CARTESIAN_POINT('Ctrl Pts',(16.9282197485466,-2.39534565917475,1.06620536369302));
#80015=CARTESIAN_POINT('Ctrl Pts',(16.8511967750666,-2.45346138139225,1.06121548103215));
#80016=CARTESIAN_POINT('Ctrl Pts',(16.7742286640186,-2.51153570855939,1.05622915259785));
#80017=CARTESIAN_POINT('Ctrl Pts',(16.6944679670887,-2.5660278319904,1.05124282416355));
#80018=CARTESIAN_POINT('Ctrl Pts',(16.6122848086959,-2.61666580702399,1.04625649572925));
#80019=CARTESIAN_POINT('Ctrl Pts',(16.5301313896643,-2.6672854578527,1.04127197168195));
#80020=CARTESIAN_POINT('Ctrl Pts',(16.4455576238991,-2.71405350170774,1.03628744763464));
#80021=CARTESIAN_POINT('Ctrl Pts',(16.3589623533002,-2.75674147723588,1.03130292358734));
#80022=CARTESIAN_POINT('Ctrl Pts',(16.2723748417191,-2.79942562788127,1.02631884615808));
#80023=CARTESIAN_POINT('Ctrl Pts',(16.1837665788222,-2.83803024338459,1.02133476872883));
#80024=CARTESIAN_POINT('Ctrl Pts',(16.0935597661888,-2.87237345896613,1.01635069129957));
#80025=CARTESIAN_POINT('Ctrl Pts',(16.0033364763351,-2.90672294769616,1.0113657034763));
#80026=CARTESIAN_POINT('Ctrl Pts',(15.9115144666329,-2.93680933462643,1.00638071565303));
#80027=CARTESIAN_POINT('Ctrl Pts',(15.8185336006982,-2.96249978810598,1.00139572782976));
#80028=CARTESIAN_POINT('Ctrl Pts',(15.7254532699317,-2.98821772354768,0.996405407393469));
#80029=CARTESIAN_POINT('Ctrl Pts',(15.6312120314289,-3.00953022070407,0.991415086957177));
#80030=CARTESIAN_POINT('Ctrl Pts',(15.5362622950073,-3.02635506855252,0.986424766520887));
#80031=CARTESIAN_POINT('Ctrl Pts',(15.4412564901616,-3.04318985158078,0.981431499268601));
#80032=CARTESIAN_POINT('Ctrl Pts',(15.345541788988,-3.05553165254109,0.976438232016316));
#80033=CARTESIAN_POINT('Ctrl Pts',(15.2495760194569,-3.06335013678033,0.97144496476403));
#80034=CARTESIAN_POINT('Ctrl Pts',(15.1534571521734,-3.07118109413753,0.966443731567249));
#80035=CARTESIAN_POINT('Ctrl Pts',(15.0570868546531,-3.07447431111347,0.961442498370468));
#80036=CARTESIAN_POINT('Ctrl Pts',(14.9609231734083,-3.07325157636395,0.956441265173687));
#80037=CARTESIAN_POINT('Ctrl Pts',(14.90778819723,-3.07257595765898,0.953677847599264));
#80038=CARTESIAN_POINT('Ctrl Pts',(14.8547162292643,-3.07052250404811,0.95091443002484));
#80039=CARTESIAN_POINT('Ctrl Pts',(14.8017835398299,-3.0671016424171,0.948151012450417));
#80040=CARTESIAN_POINT('Ctrl Pts',(14.7059710668605,-3.06090960464127,0.943149001887909));
#80041=CARTESIAN_POINT('Ctrl Pts',(14.6102826025438,-3.05021291769368,0.938146991325403));
#80042=CARTESIAN_POINT('Ctrl Pts',(14.5151751784807,-3.03502012224611,0.933144980762894));
#80043=CARTESIAN_POINT('Ctrl Pts',(14.4201959021657,-3.0198477975719,0.928149709909677));
#80044=CARTESIAN_POINT('Ctrl Pts',(14.3257965394092,-3.00019147337784,0.923154439056459));
#80045=CARTESIAN_POINT('Ctrl Pts',(14.232431163035,-2.97611161257776,0.918159168203242));
#80046=CARTESIAN_POINT('Ctrl Pts',(14.1391635207521,-2.95205695837359,0.91316912635757));
#80047=CARTESIAN_POINT('Ctrl Pts',(14.0469281354202,-2.92358808199884,0.908179084511899));
#80048=CARTESIAN_POINT('Ctrl Pts',(13.9561700024301,-2.89081669881942,0.903189042666227));
#80049=CARTESIAN_POINT('Ctrl Pts',(13.8654760443595,-2.85806848822858,0.898202529270548));
#80050=CARTESIAN_POINT('Ctrl Pts',(13.7762576732555,-2.82102396739934,0.893216015874868));
#80051=CARTESIAN_POINT('Ctrl Pts',(13.6889448638851,-2.77984472229418,0.888229502479189));
#80052=CARTESIAN_POINT('Ctrl Pts',(13.6016633716216,-2.73868024724197,0.883244777631761));
#80053=CARTESIAN_POINT('Ctrl Pts',(13.5162864791779,-2.69338418149762,0.878260052784337));
#80054=CARTESIAN_POINT('Ctrl Pts',(13.4332234124963,-2.64416591288258,0.873275327936909));
#80055=CARTESIAN_POINT('Ctrl Pts',(13.3501675300782,-2.59495190123789,0.868291034226667));
#80056=CARTESIAN_POINT('Ctrl Pts',(13.2694254525897,-2.54181658491102,0.863306740516423));
#80057=CARTESIAN_POINT('Ctrl Pts',(13.1913801241305,-2.48501436507108,0.858322446806182));
#80058=CARTESIAN_POINT('Ctrl Pts',(13.1133203034898,-2.42820159766742,0.853337227565992));
#80059=CARTESIAN_POINT('Ctrl Pts',(13.0379585808719,-2.36772083244518,0.848352008325803));
#80060=CARTESIAN_POINT('Ctrl Pts',(12.9656464668122,-2.30386804136134,0.843366789085613));
#80061=CARTESIAN_POINT('Ctrl Pts',(12.8932566914509,-2.23994667406553,0.838376215851565));
#80062=CARTESIAN_POINT('Ctrl Pts',(12.823923392296,-2.17264634182216,0.833385642617515));
#80063=CARTESIAN_POINT('Ctrl Pts',(12.7579625247845,-2.10230117008223,0.828395069383467));
#80064=CARTESIAN_POINT('Ctrl Pts',(12.6919625443282,-2.03191428562805,0.823401536879435));
#80065=CARTESIAN_POINT('Ctrl Pts',(12.6293392617936,-1.95847929996441,0.818408004375404));
#80066=CARTESIAN_POINT('Ctrl Pts',(12.5703681319383,-1.88236320504285,0.813414471871371));
#80067=CARTESIAN_POINT('Ctrl Pts',(12.5113027306581,-1.80612543070379,0.808412956691309));
#80068=CARTESIAN_POINT('Ctrl Pts',(12.4559013912022,-1.72719834772307,0.803411441511248));
#80069=CARTESIAN_POINT('Ctrl Pts',(12.4043960227106,-1.64597759495063,0.798409926331186));
#80070=CARTESIAN_POINT('Ctrl Pts',(12.3759596580807,-1.60113522202919,0.795648565457015));
#80071=CARTESIAN_POINT('Ctrl Pts',(12.3487100495383,-1.55559413528145,0.792887204582844));
#80072=CARTESIAN_POINT('Ctrl Pts',(12.3226800398894,-1.50942375799289,0.790125843708672));
#80073=CARTESIAN_POINT('Ctrl Pts',(12.2735423910071,-1.42226651838476,0.784913137954711));
#80074=CARTESIAN_POINT('Ctrl Pts',(12.2285939954989,-1.33258274597609,0.779700432200751));
#80075=CARTESIAN_POINT('Ctrl Pts',(12.188090757582,-1.24079356155826,0.77448772644679));
#80076=CARTESIAN_POINT('Ctrl Pts',(12.1476603528802,-1.14916943311491,0.76928439421797));
#80077=CARTESIAN_POINT('Ctrl Pts',(12.1116593496754,-1.0554477792978,0.76408106198915));
#80078=CARTESIAN_POINT('Ctrl Pts',(12.0802982731441,-0.960075036752079,
0.75887772976033));
#80079=CARTESIAN_POINT('Ctrl Pts',(12.0490053639031,-0.864909598998068,
0.753685707636213));
#80080=CARTESIAN_POINT('Ctrl Pts',(12.0223324057197,-0.76810058798344,0.748493685512095));
#80081=CARTESIAN_POINT('Ctrl Pts',(12.0004417921737,-0.670114026015082,
0.743301663387977));
#80082=CARTESIAN_POINT('Ctrl Pts',(11.9785799823023,-0.572256394787969,
0.73811647292779));
#80083=CARTESIAN_POINT('Ctrl Pts',(11.961488078542,-0.473224670510129,0.732931282467602));
#80084=CARTESIAN_POINT('Ctrl Pts',(11.9492787988412,-0.373500204551646,
0.727746092007415));
#80085=CARTESIAN_POINT('Ctrl Pts',(11.9370878120961,-0.273925154061226,
0.722568670429739));
#80086=CARTESIAN_POINT('Ctrl Pts',(11.9297649225634,-0.173659811268035,
0.717391248852062));
#80087=CARTESIAN_POINT('Ctrl Pts',(11.927371687701,-0.0731949756367123,
0.712213827274386));
#80088=CARTESIAN_POINT('Ctrl Pts',(11.9267876601978,-0.048678273149109,
0.710950367242076));
#80089=CARTESIAN_POINT('Ctrl Pts',(11.9264969631059,-0.0241497297134993,
0.709686907209766));
#80090=CARTESIAN_POINT('Ctrl Pts',(11.9265000239204,0.000383456645624363,
0.708423447177456));
#80091=CARTESIAN_POINT('Ctrl Pts',(11.93146095593,0.00038659779505148,0.708423253219806));
#80092=CARTESIAN_POINT('Ctrl Pts',(11.9310937115442,0.493586194944426,0.682982393802185));
#80093=CARTESIAN_POINT('Ctrl Pts',(12.275455933301,2.00734761848573,0.604866478137318));
#80094=CARTESIAN_POINT('Ctrl Pts',(14.4123128401962,3.45239818247855,0.486829844919761));
#80095=CARTESIAN_POINT('Ctrl Pts',(16.256580383956,2.90127052393581,0.394234071119828));
#80096=CARTESIAN_POINT('Ctrl Pts',(16.8725886476925,2.43775122616123,0.354313353567141));
#80097=CARTESIAN_POINT('',(11.9265000946077,0.000762596727450985,0.791576552865784));
#80098=CARTESIAN_POINT('Ctrl Pts',(11.9265000946079,0.000762597557556419,
0.791576552822547));
#80099=CARTESIAN_POINT('Ctrl Pts',(11.9265102684111,0.0417661159950146,
0.789440845722602));
#80100=CARTESIAN_POINT('Ctrl Pts',(11.9273409490568,0.0827585467976382,
0.787305138622661));
#80101=CARTESIAN_POINT('Ctrl Pts',(11.9289910136247,0.123717644668866,0.785169431522718));
#80102=CARTESIAN_POINT('Ctrl Pts',(11.9328555153485,0.219645105569208,0.780167540124415));
#80103=CARTESIAN_POINT('Ctrl Pts',(11.9412257044201,0.315558408633647,0.77516564872611));
#80104=CARTESIAN_POINT('Ctrl Pts',(11.9541042636064,0.411000502456114,0.770163757327807));
#80105=CARTESIAN_POINT('Ctrl Pts',(11.9669654222801,0.506313642307278,0.765168624098085));
#80106=CARTESIAN_POINT('Ctrl Pts',(11.9843227863911,0.601156407398729,0.760173490868364));
#80107=CARTESIAN_POINT('Ctrl Pts',(12.00612705987,0.695073426594247,0.755178357638643));
#80108=CARTESIAN_POINT('Ctrl Pts',(12.0279084296238,0.78889179312916,0.750188471415134));
#80109=CARTESIAN_POINT('Ctrl Pts',(12.0541273238847,0.881785922065945,0.745198585191627));
#80110=CARTESIAN_POINT('Ctrl Pts',(12.0846829867416,0.973308256518122,0.740208698968118));
#80111=CARTESIAN_POINT('Ctrl Pts',(12.1152168847939,1.0647653995936,0.73522236704154));
#80112=CARTESIAN_POINT('Ctrl Pts',(12.1500812718183,1.15485227599997,0.730236035114959));
#80113=CARTESIAN_POINT('Ctrl Pts',(12.1891251681878,1.24313512133021,0.725249703188382));
#80114=CARTESIAN_POINT('Ctrl Pts',(12.2281549355248,1.33138601925478,0.720265175693552));
#80115=CARTESIAN_POINT('Ctrl Pts',(12.271361029811,1.41783378265897,0.715280648198722));
#80116=CARTESIAN_POINT('Ctrl Pts',(12.3185441745335,1.50206421502933,0.710296120703892));
#80117=CARTESIAN_POINT('Ctrl Pts',(12.365723091145,1.58628709945819,0.705312039875675));
#80118=CARTESIAN_POINT('Ctrl Pts',(12.4168781351221,1.66829266547198,0.700327959047457));
#80119=CARTESIAN_POINT('Ctrl Pts',(12.471764384952,1.74769188497363,0.69534387821924));
#80120=CARTESIAN_POINT('Ctrl Pts',(12.526660659747,1.82710560673066,0.690358887049416));
#80121=CARTESIAN_POINT('Ctrl Pts',(12.5852892445217,1.90391167586761,0.685373895879593));
#80122=CARTESIAN_POINT('Ctrl Pts',(12.6473628880279,1.97775146804938,0.680388904709768));
#80123=CARTESIAN_POINT('Ctrl Pts',(12.7095029325691,2.05167024767821,0.675398581025936));
#80124=CARTESIAN_POINT('Ctrl Pts',(12.7750951102901,2.12261607957009,0.670408257342104));
#80125=CARTESIAN_POINT('Ctrl Pts',(12.8438131569517,2.19026494923906,0.665417933658272));
#80126=CARTESIAN_POINT('Ctrl Pts',(12.9125717813246,2.25795376527506,0.660424663209736));
#80127=CARTESIAN_POINT('Ctrl Pts',(12.9844596236029,2.32234145009085,0.6554313927612));
#80128=CARTESIAN_POINT('Ctrl Pts',(13.059116569471,2.38314367151833,0.650438122312663));
#80129=CARTESIAN_POINT('Ctrl Pts',(13.1338926166026,2.44404289157491,0.645436886030366));
#80130=CARTESIAN_POINT('Ctrl Pts',(13.2114462355921,2.50134496681132,0.640435649748068));
#80131=CARTESIAN_POINT('Ctrl Pts',(13.2913876071823,2.55480839616396,0.635434413465771));
#80132=CARTESIAN_POINT('Ctrl Pts',(13.3355584200923,2.5843490844019,0.632671029904176));
#80133=CARTESIAN_POINT('Ctrl Pts',(13.3804577527622,2.61271863442847,0.629907646342582));
#80134=CARTESIAN_POINT('Ctrl Pts',(13.4260168470823,2.63988243759665,0.627144262780988));
#80135=CARTESIAN_POINT('Ctrl Pts',(13.5084837698325,2.68905187985409,0.622142237562878));
#80136=CARTESIAN_POINT('Ctrl Pts',(13.5934001254049,2.73443876140458,0.617140212344768));
#80137=CARTESIAN_POINT('Ctrl Pts',(13.6803844323884,2.77579123921758,0.612138187126659));
#80138=CARTESIAN_POINT('Ctrl Pts',(13.7672515386383,2.81708799961554,0.607142901526823));
#80139=CARTESIAN_POINT('Ctrl Pts',(13.8561806658599,2.85436097341372,0.602147615926989));
#80140=CARTESIAN_POINT('Ctrl Pts',(13.9467633602653,2.88740278290375,0.597152330327153));
#80141=CARTESIAN_POINT('Ctrl Pts',(14.0372512350179,2.92041000507086,0.5921622736648));
#80142=CARTESIAN_POINT('Ctrl Pts',(14.1293888261519,2.94919471850926,0.587172217002445));
#80143=CARTESIAN_POINT('Ctrl Pts',(14.2227461292744,2.97359692467593,0.582182160340092));
#80144=CARTESIAN_POINT('Ctrl Pts',(14.3160374205969,2.99798187634294,0.57719563208539));
#80145=CARTESIAN_POINT('Ctrl Pts',(14.4105462863825,3.0179903706246,0.57220910383069));
#80146=CARTESIAN_POINT('Ctrl Pts',(14.5058268521429,3.03351201578913,0.567222575575988));
#80147=CARTESIAN_POINT('Ctrl Pts',(14.6010732434356,3.04902809377469,0.562237835849172));
#80148=CARTESIAN_POINT('Ctrl Pts',(14.6970903524384,3.0600604498773,0.557253096122355));
#80149=CARTESIAN_POINT('Ctrl Pts',(14.7934223269749,3.06654983898966,0.55226835639554));
#80150=CARTESIAN_POINT('Ctrl Pts',(14.88974596966,3.0730386668281,0.547284047803976));
#80151=CARTESIAN_POINT('Ctrl Pts',(14.9863839862799,3.07498527967503,0.542299739212411));
#80152=CARTESIAN_POINT('Ctrl Pts',(15.0828766862315,3.07238241514289,0.537315430620848));
#80153=CARTESIAN_POINT('Ctrl Pts',(15.1793873034701,3.06977906729678,0.532330196515882));
#80154=CARTESIAN_POINT('Ctrl Pts',(15.2757521121938,3.0626245761527,0.52734496241092));
#80155=CARTESIAN_POINT('Ctrl Pts',(15.3715137788867,3.05096374316335,0.522359728305954));
#80156=CARTESIAN_POINT('Ctrl Pts',(15.4673782885559,3.03929038705477,0.517369140322651));
#80157=CARTESIAN_POINT('Ctrl Pts',(15.5626379271535,3.02310108065177,0.512378552339349));
#80158=CARTESIAN_POINT('Ctrl Pts',(15.6568430504918,3.00249220765361,0.507387964356046));
#80159=CARTESIAN_POINT('Ctrl Pts',(15.7511040338299,2.98187111438971,0.502394417146811));
#80160=CARTESIAN_POINT('Ctrl Pts',(15.8443088336417,2.95682535001433,0.497400869937575));
#80161=CARTESIAN_POINT('Ctrl Pts',(15.9360225654421,2.9275013248474,0.49240732272834));
#80162=CARTESIAN_POINT('Ctrl Pts',(16.0278829067494,2.89813042359346,0.487405793055847));
#80163=CARTESIAN_POINT('Ctrl Pts',(16.1182470102679,2.86446775891739,0.482404263383352));
#80164=CARTESIAN_POINT('Ctrl Pts',(16.2066996507123,2.82670801516018,0.477402733710859));
#80165=CARTESIAN_POINT('Ctrl Pts',(16.2555320312988,2.80586185196218,0.474641520486987));
#80166=CARTESIAN_POINT('Ctrl Pts',(16.3037822453033,2.78376778355852,0.471880307263116));
#80167=CARTESIAN_POINT('Ctrl Pts',(16.3513839134321,2.76046441174612,0.469119094039244));
#80168=CARTESIAN_POINT('Ctrl Pts',(16.4374993846867,2.71830662769506,0.464123824180957));
#80169=CARTESIAN_POINT('Ctrl Pts',(16.5217927731749,2.67204060736011,0.459128554322671));
#80170=CARTESIAN_POINT('Ctrl Pts',(16.6038453090492,2.62184714936641,0.454133284464384));
#80171=CARTESIAN_POINT('Ctrl Pts',(16.6857774726772,2.57172732589509,0.449145342738585));
#80172=CARTESIAN_POINT('Ctrl Pts',(16.7654749475324,2.51769174789098,0.444157401012784));
#80173=CARTESIAN_POINT('Ctrl Pts',(16.842541521382,2.4599680875945,0.439169459286985));
#80174=CARTESIAN_POINT('Ctrl Pts',(16.8525088698863,2.45250244055218,0.438524347521702));
#80175=CARTESIAN_POINT('Ctrl Pts',(16.8624322437064,2.44497516489369,0.43787923575642));
#80176=CARTESIAN_POINT('Ctrl Pts',(16.8723108164276,2.43738680900022,0.437234123991137));
#80177=CARTESIAN_POINT('Ctrl Pts',(16.8723108164276,2.43738680900023,1.43740555432678));
#80178=CARTESIAN_POINT('Ctrl Pts',(16.9487418871335,2.37867527422642,1.43240470324732));
#80179=CARTESIAN_POINT('Ctrl Pts',(17.0223095105188,2.31644150982458,1.42740385216786));
#80180=CARTESIAN_POINT('Ctrl Pts',(17.0926908320212,2.251010291308,1.4224030010884));
#80181=CARTESIAN_POINT('Ctrl Pts',(17.1167707269066,2.22862399860322,1.42069203622215));
#80182=CARTESIAN_POINT('Ctrl Pts',(17.1404779828383,2.20586372150002,1.41898107135591));
#80183=CARTESIAN_POINT('Ctrl Pts',(17.163800751531,2.1827433558882,1.41727010648966));
#80184=CARTESIAN_POINT('Ctrl Pts',(17.2319678784332,2.11516780697037,1.41226934690146));
#80185=CARTESIAN_POINT('Ctrl Pts',(17.2970853426487,2.04427799071225,1.40726858731326));
#80186=CARTESIAN_POINT('Ctrl Pts',(17.3588141257413,1.97038020955432,1.40226782772507));
#80187=CARTESIAN_POINT('Ctrl Pts',(17.4204595366264,1.89658223631145,1.39727382226914));
#80188=CARTESIAN_POINT('Ctrl Pts',(17.4787250838348,1.81978470635024,1.39227981681321));
#80189=CARTESIAN_POINT('Ctrl Pts',(17.533308060935,1.74033115193675,1.38728581135728));
#80190=CARTESIAN_POINT('Ctrl Pts',(17.5878337497707,1.66096098902162,1.38229704742391));
#80191=CARTESIAN_POINT('Ctrl Pts',(17.6386843051097,1.57894070316164,1.37730828349053));
#80192=CARTESIAN_POINT('Ctrl Pts',(17.6855975113525,1.49464653246751,1.37231951955716));
#80193=CARTESIAN_POINT('Ctrl Pts',(17.7324774131216,1.41041220362208,1.36733429723116));
#80194=CARTESIAN_POINT('Ctrl Pts',(17.7754253098421,1.32390758132023,1.36234907490517));
#80195=CARTESIAN_POINT('Ctrl Pts',(17.814223055485,1.23553666233609,1.35736385257917));
#80196=CARTESIAN_POINT('Ctrl Pts',(17.853006822366,1.14719758324431,1.35238042642033));
#80197=CARTESIAN_POINT('Ctrl Pts',(17.8876432330553,1.05699394482163,1.34739700026148));
#80198=CARTESIAN_POINT('Ctrl Pts',(17.917961175185,0.965352179317362,1.34241357410264));
#80199=CARTESIAN_POINT('Ctrl Pts',(17.9482764581108,0.873718451764499,1.33743058504294));
#80200=CARTESIAN_POINT('Ctrl Pts',(17.9742738879916,0.780647264485796,1.33244759598325));
#80201=CARTESIAN_POINT('Ctrl Pts',(17.9958317302719,0.686581745967842,1.32746460692355));
#80202=CARTESIAN_POINT('Ctrl Pts',(18.0173935580156,0.592498837272972,1.32248069664359));
#80203=CARTESIAN_POINT('Ctrl Pts',(18.0345140701432,0.497421659861666,1.31749678636364));
#80204=CARTESIAN_POINT('Ctrl Pts',(18.0471225362022,0.401804055938678,1.31251287608368));
#80205=CARTESIAN_POINT('Ctrl Pts',(18.059744550821,0.306083705114281,1.30752361029054));
#80206=CARTESIAN_POINT('Ctrl Pts',(18.0678447826611,0.209822204081699,1.3025343444974));
#80207=CARTESIAN_POINT('Ctrl Pts',(18.0714043704515,0.113478822566934,1.29754507870427));
#80208=CARTESIAN_POINT('Ctrl Pts',(18.0749660687942,0.0170783170949871,
1.29255285467361));
#80209=CARTESIAN_POINT('Ctrl Pts',(18.0739817668327,-0.0794037270874671,
1.28756063064296));
#80210=CARTESIAN_POINT('Ctrl Pts',(18.0684847305754,-0.175509852218593,
1.28256840661231));
#80211=CARTESIAN_POINT('Ctrl Pts',(18.0629788920172,-0.271769870280725,
1.27756818862719));
#80212=CARTESIAN_POINT('Ctrl Pts',(18.052945936315,-0.367652331417721,1.27256797064207));
#80213=CARTESIAN_POINT('Ctrl Pts',(18.0384707819403,-0.462706772476012,
1.26756775265695));
#80214=CARTESIAN_POINT('Ctrl Pts',(18.0304395300363,-0.515445841156773,
1.26479348102061));
#80215=CARTESIAN_POINT('Ctrl Pts',(18.0210417158762,-0.567930216229394,
1.26201920938427));
#80216=CARTESIAN_POINT('Ctrl Pts',(18.0102984817983,-0.620084913929582,
1.25924493774793));
#80217=CARTESIAN_POINT('Ctrl Pts',(17.99093241947,-0.714100470050287,1.25424395601049));
#80218=CARTESIAN_POINT('Ctrl Pts',(17.9671240151282,-0.807371905796901,
1.24924297427306));
#80219=CARTESIAN_POINT('Ctrl Pts',(17.9389446606578,-0.899447903767208,
1.24424199253562));
#80220=CARTESIAN_POINT('Ctrl Pts',(17.9108033673361,-0.991399536991763,
1.23924776549904));
#80221=CARTESIAN_POINT('Ctrl Pts',(17.8783029846973,-1.08215852561021,1.23425353846245));
#80222=CARTESIAN_POINT('Ctrl Pts',(17.8415659243467,-1.17128363242723,1.22925931142587));
#80223=CARTESIAN_POINT('Ctrl Pts',(17.8048674264319,-1.26031518572674,1.22427032676737));
#80224=CARTESIAN_POINT('Ctrl Pts',(17.7639412580249,-1.34771586332309,1.21928134210886));
#80225=CARTESIAN_POINT('Ctrl Pts',(17.7189593437629,-1.43306047917184,1.21429235745036));
#80226=CARTESIAN_POINT('Ctrl Pts',(17.6740093810356,-1.51834447306863,1.20930691656536));
#80227=CARTESIAN_POINT('Ctrl Pts',(17.6250096035478,-1.60157492164121,1.20432147568036));
#80228=CARTESIAN_POINT('Ctrl Pts',(17.5721792599945,-1.68234838973802,1.19933603479537));
#80229=CARTESIAN_POINT('Ctrl Pts',(17.5193679653499,-1.76309273354149,1.19435239149869));
#80230=CARTESIAN_POINT('Ctrl Pts',(17.462729088836,-1.8413814903884,1.18936874820201));
#80231=CARTESIAN_POINT('Ctrl Pts',(17.4025263638967,-1.91683836584653,1.18438510490533));
#80232=CARTESIAN_POINT('Ctrl Pts',(17.3423289394216,-1.9922885978103,1.17940190038651));
#80233=CARTESIAN_POINT('Ctrl Pts',(17.2785685641232,-2.06490710135893,1.17441869586768));
#80234=CARTESIAN_POINT('Ctrl Pts',(17.2115499297707,-2.13434982093642,1.16943549134886));
#80235=CARTESIAN_POINT('Ctrl Pts',(17.1445189320766,-2.20380535104145,1.16445136754751));
#80236=CARTESIAN_POINT('Ctrl Pts',(17.0742287862168,-2.27008361804563,1.15946724374617));
#80237=CARTESIAN_POINT('Ctrl Pts',(17.0010210200543,-2.33287743512191,1.15448311994482));
#80238=CARTESIAN_POINT('Ctrl Pts',(16.9277346531377,-2.39573867184,1.14949364485481));
#80239=CARTESIAN_POINT('Ctrl Pts',(16.8515247457088,-2.45510770393165,1.14450416976479));
#80240=CARTESIAN_POINT('Ctrl Pts',(16.7727657065589,-2.51071782557272,1.13951469467478));
#80241=CARTESIAN_POINT('Ctrl Pts',(16.6939600044306,-2.56636089497363,1.13452226343179));
#80242=CARTESIAN_POINT('Ctrl Pts',(16.6126025329471,-2.61824038368877,1.12952983218879));
#80243=CARTESIAN_POINT('Ctrl Pts',(16.5290946600094,-2.66613423719263,1.1245374009458));
#80244=CARTESIAN_POINT('Ctrl Pts',(16.4454531613369,-2.71410472839716,1.11953698102737));
#80245=CARTESIAN_POINT('Ctrl Pts',(16.3596547806514,-2.75807665023309,1.11453656110893));
#80246=CARTESIAN_POINT('Ctrl Pts',(16.2721232444532,-2.79787503311384,1.1095361411905));
#80247=CARTESIAN_POINT('Ctrl Pts',(16.2235976642845,-2.81993839110969,1.10676401712906));
#80248=CARTESIAN_POINT('Ctrl Pts',(16.1745397518106,-2.84071994360021,1.10399189306762));
#80249=CARTESIAN_POINT('Ctrl Pts',(16.1250236863888,-2.86019648889098,1.10121976900619));
#80250=CARTESIAN_POINT('Ctrl Pts',(16.0356933907305,-2.89533347997462,1.09621867168757));
#80251=CARTESIAN_POINT('Ctrl Pts',(15.9445596851152,-2.9263427387285,1.09121757436896));
#80252=CARTESIAN_POINT('Ctrl Pts',(15.8520396290823,-2.95303754132475,1.08621647705035));
#80253=CARTESIAN_POINT('Ctrl Pts',(15.7596444867547,-2.97969630258196,1.08122213184176));
#80254=CARTESIAN_POINT('Ctrl Pts',(15.6658671319447,-3.0020520642932,1.07622778663316));
#80255=CARTESIAN_POINT('Ctrl Pts',(15.5711440478102,-3.01996634528449,1.07123344142456));
#80256=CARTESIAN_POINT('Ctrl Pts',(15.476520345553,-3.03786183091146,1.06624433619952));
#80257=CARTESIAN_POINT('Ctrl Pts',(15.3809533152628,-3.05132501860483,1.06125523097447));
#80258=CARTESIAN_POINT('Ctrl Pts',(15.2848930395133,-3.060267669018,1.05626612574943));
#80259=CARTESIAN_POINT('Ctrl Pts',(15.1889009372904,-3.06920397287417,1.05128056126893));
#80260=CARTESIAN_POINT('Ctrl Pts',(15.092416721016,-3.07362607677781,1.04629499678843));
#80261=CARTESIAN_POINT('Ctrl Pts',(14.9958981032323,-3.07349726280062,1.04130943230793));
#80262=CARTESIAN_POINT('Ctrl Pts',(14.8994142507982,-3.07336849522135,1.03632566359385));
#80263=CARTESIAN_POINT('Ctrl Pts',(14.8028964596618,-3.06869206737867,1.03134189487976));
#80264=CARTESIAN_POINT('Ctrl Pts',(14.7068040067704,-3.05948334846818,1.02635812616567));
#80265=CARTESIAN_POINT('Ctrl Pts',(14.610719982083,-3.0502754372482,1.02137479457457));
#80266=CARTESIAN_POINT('Ctrl Pts',(14.515061658071,-3.03653606739773,1.01639146298346));
#80267=CARTESIAN_POINT('Ctrl Pts',(14.4202836798045,-3.01833252609764,1.01140813139236));
#80268=CARTESIAN_POINT('Ctrl Pts',(14.3254881893817,-3.00012562132361,1.00642387902954));
#80269=CARTESIAN_POINT('Ctrl Pts',(14.2315737984917,-2.97745298969018,1.00143962666673));
#80270=CARTESIAN_POINT('Ctrl Pts',(14.138984390863,-2.95043291244225,0.996455374303908));
#80271=CARTESIAN_POINT('Ctrl Pts',(14.0462955485446,-2.92338381747979,0.991465769195024));
#80272=CARTESIAN_POINT('Ctrl Pts',(13.9549349519283,-2.89197807926445,0.98647616408614));
#80273=CARTESIAN_POINT('Ctrl Pts',(13.8653305375861,-2.85638363338424,0.981486558977256));
#80274=CARTESIAN_POINT('Ctrl Pts',(13.7756730178246,-2.82076809191418,0.976493996702998));
#80275=CARTESIAN_POINT('Ctrl Pts',(13.6877741521712,-2.78095908051636,0.971501434428742));
#80276=CARTESIAN_POINT('Ctrl Pts',(13.6020392023819,-2.73717150692516,0.966508872154485));
#80277=CARTESIAN_POINT('Ctrl Pts',(13.5161670619236,-2.69331386568329,0.961508320921701));
#80278=CARTESIAN_POINT('Ctrl Pts',(13.4324661316727,-2.64546516798433,0.956507769688916));
#80279=CARTESIAN_POINT('Ctrl Pts',(13.3513144472805,-2.59388476965609,0.951507218456132));
#80280=CARTESIAN_POINT('Ctrl Pts',(13.3063472068996,-2.56530337682445,0.948736345725575));
#80281=CARTESIAN_POINT('Ctrl Pts',(13.2621621416622,-2.53557694537095,0.945965472995017));
#80282=CARTESIAN_POINT('Ctrl Pts',(13.2188191240773,-2.50475486569991,0.94319460026446));
#80283=CARTESIAN_POINT('Ctrl Pts',(13.1411026375429,-2.44948913033611,0.938226268448822));
#80284=CARTESIAN_POINT('Ctrl Pts',(13.0658163178445,-2.39050011911477,0.933257936633185));
#80285=CARTESIAN_POINT('Ctrl Pts',(12.993341590778,-2.32803012839154,0.928289604817548));
#80286=CARTESIAN_POINT('Ctrl Pts',(12.9209650615504,-2.2656447798371,0.923328004720215));
#80287=CARTESIAN_POINT('Ctrl Pts',(12.851392890196,-2.19978811067773,0.918366404622881));
#80288=CARTESIAN_POINT('Ctrl Pts',(12.7849769697351,-2.13074522770695,0.913404804525548));
#80289=CARTESIAN_POINT('Ctrl Pts',(12.7170273221634,-2.06010795380276,0.908328627373058));
#80290=CARTESIAN_POINT('Ctrl Pts',(12.6523818995062,-1.98613574498245,0.903252450220569));
#80291=CARTESIAN_POINT('Ctrl Pts',(12.591381212228,-1.90917725347645,0.898176273068079));
#80292=CARTESIAN_POINT('Ctrl Pts',(12.5318614696195,-1.83408712235883,0.893223332846699));
#80293=CARTESIAN_POINT('Ctrl Pts',(12.4758117997149,-1.75615442742861,0.888270392625318));
#80294=CARTESIAN_POINT('Ctrl Pts',(12.423509743578,-1.67573870533634,0.883317452403938));
#80295=CARTESIAN_POINT('Ctrl Pts',(12.371224912302,-1.59534946689947,0.87836614335565));
#80296=CARTESIAN_POINT('Ctrl Pts',(12.3226854854737,-1.51247919856714,0.873414834307364));
#80297=CARTESIAN_POINT('Ctrl Pts',(12.2781261773748,-1.42751712553921,0.868463525259076));
#80298=CARTESIAN_POINT('Ctrl Pts',(12.233568985247,-1.34255908707331,0.863512451331738));
#80299=CARTESIAN_POINT('Ctrl Pts',(12.1929917421335,-1.25550983595175,0.858561377404399));
#80300=CARTESIAN_POINT('Ctrl Pts',(12.1565830637728,-1.16678291758856,0.853610303477062));
#80301=CARTESIAN_POINT('Ctrl Pts',(12.118568299928,-1.07414201437193,0.848440824259455));
#80302=CARTESIAN_POINT('Ctrl Pts',(12.0850985616984,-0.979672504177722,
0.843271345041847));
#80303=CARTESIAN_POINT('Ctrl Pts',(12.056331770515,-0.883866282149559,0.838101865824241));
#80304=CARTESIAN_POINT('Ctrl Pts',(12.0287437004715,-0.791985726300763,
0.833144206353827));
#80305=CARTESIAN_POINT('Ctrl Pts',(12.0054807933222,-0.698876309440068,
0.828186546883415));
#80306=CARTESIAN_POINT('Ctrl Pts',(11.9866303353989,-0.604983896035051,
0.823228887413001));
#80307=CARTESIAN_POINT('Ctrl Pts',(11.9677673215222,-0.511028942570008,
0.818267925734138));
#80308=CARTESIAN_POINT('Ctrl Pts',(11.9533226715503,-0.416290393835121,
0.813306964055275));
#80309=CARTESIAN_POINT('Ctrl Pts',(11.9433318910098,-0.321220051494601,
0.808346002376412));
#80310=CARTESIAN_POINT('Ctrl Pts',(11.9333265779387,-0.226011420394089,
0.803377824511912));
#80311=CARTESIAN_POINT('Ctrl Pts',(11.9277880803185,-0.130470475492244,
0.798409646647412));
#80312=CARTESIAN_POINT('Ctrl Pts',(11.92669985314,-0.035049355345871,0.793441468782912));
#80313=CARTESIAN_POINT('Ctrl Pts',(11.9265636897254,-0.023109876349453,
0.792819830143869));
#80314=CARTESIAN_POINT('Ctrl Pts',(11.9264971333298,-0.0111722661562855,
0.792198191504826));
#80315=CARTESIAN_POINT('Ctrl Pts',(11.9265000946077,0.00076259672746494,
0.791576552865783));
#80316=CARTESIAN_POINT('Origin',(15.,0.,8.20842344717745));
#80317=CARTESIAN_POINT('',(16.8723108164276,2.43738680900022,2.43734748439975));
#80318=CARTESIAN_POINT('',(16.8745674052796,2.44028174751842,2.35408151804441));
#80319=CARTESIAN_POINT('',(16.8723108164276,2.43738680900022,8.20842344717745));
#80320=CARTESIAN_POINT('',(11.9265010952115,-0.0025946606954943,1.70842344717746));
#80321=CARTESIAN_POINT('Ctrl Pts',(16.8745674052796,2.44028174751842,2.35408151804441));
#80322=CARTESIAN_POINT('Ctrl Pts',(17.5915515786301,1.8810510050653,2.30683846615771));
#80323=CARTESIAN_POINT('Ctrl Pts',(18.57195445782,-0.0162668050744201,2.20692035802376));
#80324=CARTESIAN_POINT('Ctrl Pts',(17.0556965627559,-2.98822639630323,2.05432719364256));
#80325=CARTESIAN_POINT('Ctrl Pts',(13.6199702038025,-3.35423301941131,1.89630202490083));
#80326=CARTESIAN_POINT('Ctrl Pts',(12.0268863100021,-1.40035468792022,1.78100077607913));
#80327=CARTESIAN_POINT('Ctrl Pts',(11.9234216648843,-0.194497604817307,
1.71837458350467));
#80328=CARTESIAN_POINT('Ctrl Pts',(11.9251450970424,-0.0025958054348495,
1.70842344717746));
#80329=CARTESIAN_POINT('Ctrl Pts',(11.9265010952115,-0.0025946606954943,
1.70842344717746));
#80330=CARTESIAN_POINT('Ctrl Pts',(11.9264210367132,0.0922384354117233,
1.70350363271174));
#80331=CARTESIAN_POINT('Ctrl Pts',(11.9307343098358,0.187216848308208,1.69858381824602));
#80332=CARTESIAN_POINT('Ctrl Pts',(11.9394546047295,0.281893833718155,1.69366400378031));
#80333=CARTESIAN_POINT('Ctrl Pts',(11.948166308935,0.376477549295093,1.6887490360075));
#80334=CARTESIAN_POINT('Ctrl Pts',(11.9612763661112,0.4707599788253,1.68383406823469));
#80335=CARTESIAN_POINT('Ctrl Pts',(11.9787464135551,0.564295150071033,1.67891910046188));
#80336=CARTESIAN_POINT('Ctrl Pts',(11.9962072615455,0.65778106716012,1.67400672083414));
#80337=CARTESIAN_POINT('Ctrl Pts',(12.0180234592683,0.750520063001247,1.6690943412064));
#80338=CARTESIAN_POINT('Ctrl Pts',(12.0441050153961,0.842073090647898,1.66418196157866));
#80339=CARTESIAN_POINT('Ctrl Pts',(12.0701804419867,0.933604602029459,1.65927073643008));
#80340=CARTESIAN_POINT('Ctrl Pts',(12.1005191119511,1.0239502635342,1.65435951128151));
#80341=CARTESIAN_POINT('Ctrl Pts',(12.1349806190297,1.11268423043766,1.64944828613293));
#80342=CARTESIAN_POINT('Ctrl Pts',(12.1694440749485,1.20142321535485,1.64453678324859));
#80343=CARTESIAN_POINT('Ctrl Pts',(12.2080306654003,1.28854990321406,1.63962528036426));
#80344=CARTESIAN_POINT('Ctrl Pts',(12.250551564298,1.37365772644274,1.63471377747993));
#80345=CARTESIAN_POINT('Ctrl Pts',(12.293113726129,1.4588481396102,1.62979750839777));
#80346=CARTESIAN_POINT('Ctrl Pts',(12.3396176159273,1.54201537104518,1.6248812393156));
#80347=CARTESIAN_POINT('Ctrl Pts',(12.3898282804378,1.62277720109616,1.61996497023344));
#80348=CARTESIAN_POINT('Ctrl Pts',(12.4400646730544,1.70358041376894,1.61504618203917));
#80349=CARTESIAN_POINT('Ctrl Pts',(12.4940113630609,1.78197539972019,1.61012739384489));
#80350=CARTESIAN_POINT('Ctrl Pts',(12.5513911754764,1.8576105820288,1.60520860565062));
#80351=CARTESIAN_POINT('Ctrl Pts',(12.6088638310716,1.93336814554642,1.60028185863047));
#80352=CARTESIAN_POINT('Ctrl Pts',(12.6697804092842,2.0063566429471,1.59535511161032));
#80353=CARTESIAN_POINT('Ctrl Pts',(12.7338248711224,2.07625926494174,1.59042836459017));
#80354=CARTESIAN_POINT('Ctrl Pts',(12.7779215682039,2.12438949601602,1.5870361388659));
#80355=CARTESIAN_POINT('Ctrl Pts',(12.8235003370015,2.17105754874544,1.58364391314163));
#80356=CARTESIAN_POINT('Ctrl Pts',(12.870448969525,2.21617117087174,1.58025168741736));
#80357=CARTESIAN_POINT('Ctrl Pts',(12.939662886243,2.28267982760693,1.57525070621411));
#80358=CARTESIAN_POINT('Ctrl Pts',(13.0121162445308,2.34605892694005,1.57024972501086));
#80359=CARTESIAN_POINT('Ctrl Pts',(13.0874945653347,2.40597697669279,1.56524874380762));
#80360=CARTESIAN_POINT('Ctrl Pts',(13.1627710746291,2.46581409671629,1.56025451729776));
#80361=CARTESIAN_POINT('Ctrl Pts',(13.2409643540982,2.52219918746141,1.55526029078791));
#80362=CARTESIAN_POINT('Ctrl Pts',(13.3217235890849,2.57483796355539,1.55026606427806));
#80363=CARTESIAN_POINT('Ctrl Pts',(13.4023980522268,2.62742148545873,1.54527708013826));
#80364=CARTESIAN_POINT('Ctrl Pts',(13.4856327508062,2.67626627209292,1.54028809599846));
#80365=CARTESIAN_POINT('Ctrl Pts',(13.5710451584194,2.72111931210729,1.53529911185867));
#80366=CARTESIAN_POINT('Ctrl Pts',(13.6563968961586,2.76594049225077,1.53031367147846));
#80367=CARTESIAN_POINT('Ctrl Pts',(13.7439228805237,2.80677535915943,1.52532823109825));
#80368=CARTESIAN_POINT('Ctrl Pts',(13.8332139058721,2.84341563274694,1.52034279071804));
#80369=CARTESIAN_POINT('Ctrl Pts',(13.922472735926,2.88004269510308,1.51535914791738));
#80370=CARTESIAN_POINT('Ctrl Pts',(14.0134949370345,2.91247800289763,1.51037550511672));
#80371=CARTESIAN_POINT('Ctrl Pts',(14.1058500172198,2.9405608407741,1.50539186231606));
#80372=CARTESIAN_POINT('Ctrl Pts',(14.1981969663038,2.96864120618887,1.50040865828394));
#80373=CARTESIAN_POINT('Ctrl Pts',(14.2918761414045,2.9923697361742,1.49542545425183));
#80374=CARTESIAN_POINT('Ctrl Pts',(14.386441558151,3.01163548399135,1.49044225021972));
#80375=CARTESIAN_POINT('Ctrl Pts',(14.4810244201531,3.03090478591852,1.48545812689521));
#80376=CARTESIAN_POINT('Ctrl Pts',(14.5764934186825,3.04570958307655,1.4804740035707));
#80377=CARTESIAN_POINT('Ctrl Pts',(14.6723930966562,3.05599017781168,1.4754898802462));
#80378=CARTESIAN_POINT('Ctrl Pts',(14.7683957392884,3.06628181051847,1.47050040561533));
#80379=CARTESIAN_POINT('Ctrl Pts',(14.864829547641,3.07203949665644,1.46551093098446));
#80380=CARTESIAN_POINT('Ctrl Pts',(14.9612348975193,3.07325552416809,1.46052145635359));
#80381=CARTESIAN_POINT('Ctrl Pts',(15.0576973656084,3.07447227215133,1.4555290255604));
#80382=CARTESIAN_POINT('Ctrl Pts',(15.1541309034876,3.07114201867648,1.4505365947672));
#80383=CARTESIAN_POINT('Ctrl Pts',(15.2500789622654,3.06330911966655,1.44554416397401));
#80384=CARTESIAN_POINT('Ctrl Pts',(15.3461805534101,3.05546368675505,1.44054374448645));
#80385=CARTESIAN_POINT('Ctrl Pts',(15.4417946796475,3.04310127835409,1.4355433249989));
#80386=CARTESIAN_POINT('Ctrl Pts',(15.5364730371926,3.02631771801399,1.43054290551135));
#80387=CARTESIAN_POINT('Ctrl Pts',(15.5889607566914,3.01701325995024,1.4277707765661));
#80388=CARTESIAN_POINT('Ctrl Pts',(15.6411611034272,3.00635092360513,1.42499864762086));
#80389=CARTESIAN_POINT('Ctrl Pts',(15.6929998032508,2.99435360682307,1.42222651867561));
#80390=CARTESIAN_POINT('Ctrl Pts',(15.7865289946372,2.97270762917992,1.41722494688563));
#80391=CARTESIAN_POINT('Ctrl Pts',(15.8792061005138,2.94663761271737,1.41222337509564));
#80392=CARTESIAN_POINT('Ctrl Pts',(15.9705815251702,2.91622594340671,1.40722180330566));
#80393=CARTESIAN_POINT('Ctrl Pts',(16.0618102063975,2.88586311340545,1.40222826373875));
#80394=CARTESIAN_POINT('Ctrl Pts',(16.1517409521813,2.85117263825007,1.39723472417185));
#80395=CARTESIAN_POINT('Ctrl Pts',(16.23993582613,2.81228757368079,1.39224118460495));
#80396=CARTESIAN_POINT('Ctrl Pts',(16.3280487064443,2.77343866005341,1.38725228746723));
#80397=CARTESIAN_POINT('Ctrl Pts',(16.4144285216831,2.73040307941623,1.38226339032952));
#80398=CARTESIAN_POINT('Ctrl Pts',(16.4986544260729,2.68336303194557,1.3772744931918));
#80399=CARTESIAN_POINT('Ctrl Pts',(16.5828202222499,2.63635655482602,1.37228915640399));
#80400=CARTESIAN_POINT('Ctrl Pts',(16.6648347817327,2.5853515055851,1.36730381961618));
#80401=CARTESIAN_POINT('Ctrl Pts',(16.7443001550306,2.53057685501947,1.36231848282837));
#80402=CARTESIAN_POINT('Ctrl Pts',(16.7877527159398,2.50062545932088,1.35959244453729));
#80403=CARTESIAN_POINT('Ctrl Pts',(16.8304434838481,2.46954775257882,1.35686640624621));
#80404=CARTESIAN_POINT('Ctrl Pts',(16.8723108164276,2.43738680900022,1.35414036795513));
#80405=CARTESIAN_POINT('',(11.9265006184838,0.00194982547800578,1.79157655278712));
#80406=CARTESIAN_POINT('Ctrl Pts',(11.9265006184838,0.00194982547801677,
1.79157655278712));
#80407=CARTESIAN_POINT('Ctrl Pts',(11.9265698355604,0.111056329985969,1.78594824763792));
#80408=CARTESIAN_POINT('Ctrl Pts',(11.9324528884889,0.219943981301199,1.78031994248873));
#80409=CARTESIAN_POINT('Ctrl Pts',(11.944055790133,0.328035419093971,1.77469163733954));
#80410=CARTESIAN_POINT('Ctrl Pts',(11.9557100333901,0.436605150071001,1.76903842753511));
#80411=CARTESIAN_POINT('Ctrl Pts',(11.9731347345555,0.544371404507665,1.76338521773069));
#80412=CARTESIAN_POINT('Ctrl Pts',(11.996184973256,0.650766882306438,1.75773200792626));
#80413=CARTESIAN_POINT('Ctrl Pts',(12.0193615261158,0.757745402020997,1.75204781881385));
#80414=CARTESIAN_POINT('Ctrl Pts',(12.0482253298664,0.863337884085554,1.74636362970144));
#80415=CARTESIAN_POINT('Ctrl Pts',(12.0825807013878,0.966988565643491,1.74067944058904));
#80416=CARTESIAN_POINT('Ctrl Pts',(12.0974066837613,1.01171878131936,1.73822644171707));
#80417=CARTESIAN_POINT('Ctrl Pts',(12.113254780959,1.05608764941845,1.7357734428451));
#80418=CARTESIAN_POINT('Ctrl Pts',(12.1301065854665,1.1000518347865,1.73332044397313));
#80419=CARTESIAN_POINT('Ctrl Pts',(12.164462065989,1.18968085424443,1.72831955787038));
#80420=CARTESIAN_POINT('Ctrl Pts',(12.2030802784572,1.2778552664331,1.72331867176762));
#80421=CARTESIAN_POINT('Ctrl Pts',(12.2458175953055,1.36414131660581,1.71831778566487));
#80422=CARTESIAN_POINT('Ctrl Pts',(12.2884971917689,1.4503108301219,1.71332365368454));
#80423=CARTESIAN_POINT('Ctrl Pts',(12.3352846428408,1.53459666069137,1.70832952170421));
#80424=CARTESIAN_POINT('Ctrl Pts',(12.3859876110696,1.61658327361088,1.70333538972388));
#80425=CARTESIAN_POINT('Ctrl Pts',(12.4366373630816,1.69848383599879,1.69834649942505));
#80426=CARTESIAN_POINT('Ctrl Pts',(12.491194232924,1.77808960697265,1.69335760912621));
#80427=CARTESIAN_POINT('Ctrl Pts',(12.5494196283456,1.85500891967181,1.68836871882738));
#80428=CARTESIAN_POINT('Ctrl Pts',(12.6076036808387,1.93187361583092,1.68338337088894));
#80429=CARTESIAN_POINT('Ctrl Pts',(12.6694508165293,2.00605529705837,1.6783980229505));
#80430=CARTESIAN_POINT('Ctrl Pts',(12.7346792726769,2.07719143372977,1.67341267501206));
#80431=CARTESIAN_POINT('Ctrl Pts',(12.7998842210012,2.14830193349622,1.66842912375387));
#80432=CARTESIAN_POINT('Ctrl Pts',(12.8684677723131,2.21636874656426,1.66344557249567));
#80433=CARTESIAN_POINT('Ctrl Pts',(12.9401086694023,2.28106333891201,1.65846202123747));
#80434=CARTESIAN_POINT('Ctrl Pts',(13.011743273447,2.34575224838913,1.65347890774194));
#80435=CARTESIAN_POINT('Ctrl Pts',(13.0864343635891,2.40706923226672,1.64849579424641));
#80436=CARTESIAN_POINT('Ctrl Pts',(13.1638254948465,2.46472421106789,1.64351268075087));
#80437=CARTESIAN_POINT('Ctrl Pts',(13.2412309206289,2.52238983902899,1.63852864684961));
#80438=CARTESIAN_POINT('Ctrl Pts',(13.3213370261886,2.57639185654604,1.63354461294836));
#80439=CARTESIAN_POINT('Ctrl Pts',(13.4037569974814,2.62648253885505,1.6285605790471));
#80440=CARTESIAN_POINT('Ctrl Pts',(13.4862654990349,2.67662702537064,1.62357119161545));
#80441=CARTESIAN_POINT('Ctrl Pts',(13.5710924526084,2.72285156117808,1.61858180418381));
#80442=CARTESIAN_POINT('Ctrl Pts',(13.6578251637094,2.76495369921961,1.61359241675217));
#80443=CARTESIAN_POINT('Ctrl Pts',(13.744609282735,2.80708079190066,1.60860007202737));
#80444=CARTESIAN_POINT('Ctrl Pts',(13.8333010054676,2.84508044886725,1.60360772730257));
#80445=CARTESIAN_POINT('Ctrl Pts',(13.9234682772436,2.87879865567203,1.59861538257777));
#80446=CARTESIAN_POINT('Ctrl Pts',(14.0137798807211,2.91257083556553,1.59361504655419));
#80447=CARTESIAN_POINT('Ctrl Pts',(14.1055713319809,2.94204774716723,1.58861471053061));
#80448=CARTESIAN_POINT('Ctrl Pts',(14.1983961503845,2.96712546385918,1.58361437450704));
#80449=CARTESIAN_POINT('Ctrl Pts',(14.2498739494698,2.98103279687194,1.58084134141516));
#80450=CARTESIAN_POINT('Ctrl Pts',(14.3016693755805,2.99358808204046,1.57806830832328));
#80451=CARTESIAN_POINT('Ctrl Pts',(14.3537053912393,3.00478044600382,1.5752952752314));
#80452=CARTESIAN_POINT('Ctrl Pts',(14.4475558636107,3.02496663112224,1.57029392256673));
#80453=CARTESIAN_POINT('Ctrl Pts',(14.5425166949139,3.04078686829603,1.56529256990206));
#80454=CARTESIAN_POINT('Ctrl Pts',(14.6381459848649,3.05212449315729,1.56029121723738));
#80455=CARTESIAN_POINT('Ctrl Pts',(14.7360484047801,3.06373161593919,1.55517098128278));
#80456=CARTESIAN_POINT('Ctrl Pts',(14.834651037717,3.07064013422976,1.55005074532817));
#80457=CARTESIAN_POINT('Ctrl Pts',(14.9334654360006,3.07277975159194,1.54493050937356));
#80458=CARTESIAN_POINT('Ctrl Pts',(15.0297349728532,3.07486426534779,1.53994213973828));
#80459=CARTESIAN_POINT('Ctrl Pts',(15.1262050293233,3.07242250789681,1.534953770103));
#80460=CARTESIAN_POINT('Ctrl Pts',(15.2224172674361,3.06544169886597,1.52996540046772));
#80461=CARTESIAN_POINT('Ctrl Pts',(15.3185662289433,3.0584654809548,1.52498031156994));
#80462=CARTESIAN_POINT('Ctrl Pts',(15.4144572728825,3.04695617520024,1.51999522267215));
#80463=CARTESIAN_POINT('Ctrl Pts',(15.5096329791833,3.03095306405902,1.51501013377437));
#80464=CARTESIAN_POINT('Ctrl Pts',(15.6047720307396,3.01495611614971,1.51002696476946));
#80465=CARTESIAN_POINT('Ctrl Pts',(15.6991958603445,2.99446887633508,1.50504379576455));
#80466=CARTESIAN_POINT('Ctrl Pts',(15.7924541456017,2.96958223949409,1.50006062675964));
#80467=CARTESIAN_POINT('Ctrl Pts',(15.8901681473408,2.94350656301284,1.49483937072356));
#80468=CARTESIAN_POINT('Ctrl Pts',(15.9866019507966,2.91260073338112,1.48961811468749));
#80469=CARTESIAN_POINT('Ctrl Pts',(16.0812530067942,2.87702870776404,1.48439685865142));
#80470=CARTESIAN_POINT('Ctrl Pts',(16.1716282965709,2.84306361261318,1.47941146760338));
#80471=CARTESIAN_POINT('Ctrl Pts',(16.2603779902462,2.80484495110589,1.47442607655533));
#80472=CARTESIAN_POINT('Ctrl Pts',(16.3470845853442,2.76256499831732,1.46944068550729));
#80473=CARTESIAN_POINT('Ctrl Pts',(16.4338218336145,2.7202700983996,1.46445353198604));
#80474=CARTESIAN_POINT('Ctrl Pts',(16.5185141581414,2.67391125463293,1.45946637846479));
#80475=CARTESIAN_POINT('Ctrl Pts',(16.60076913139,2.62372644114989,1.45447922494355));
#80476=CARTESIAN_POINT('Ctrl Pts',(16.6831075506654,2.57349071617627,1.4494870120547));
#80477=CARTESIAN_POINT('Ctrl Pts',(16.7630033204026,2.51942151976691,1.44449479916585));
#80478=CARTESIAN_POINT('Ctrl Pts',(16.8400938804713,2.46179949651716,1.439502586277));
#80479=CARTESIAN_POINT('Ctrl Pts',(16.8508881161555,2.45373124926347,1.43880357562692));
#80480=CARTESIAN_POINT('Ctrl Pts',(16.8616274084294,2.44559340972417,1.43810456497685));
#80481=CARTESIAN_POINT('Ctrl Pts',(16.8723108164276,2.43738680900023,1.43740555432678));
#80482=CARTESIAN_POINT('Ctrl Pts',(16.8723108164276,2.43738680900022,2.43734748439974));
#80483=CARTESIAN_POINT('Ctrl Pts',(16.9488595251288,2.37858490904914,2.43236381332471));
#80484=CARTESIAN_POINT('Ctrl Pts',(17.0226234707783,2.31618266128806,2.42738014224968));
#80485=CARTESIAN_POINT('Ctrl Pts',(17.0932575334937,2.25048331441755,2.42239647117465));
#80486=CARTESIAN_POINT('Ctrl Pts',(17.1639647946043,2.18471588301997,2.41740763549899));
#80487=CARTESIAN_POINT('Ctrl Pts',(17.2315353734165,2.11564482830248,2.41241879982333));
#80488=CARTESIAN_POINT('Ctrl Pts',(17.2956604304822,2.04361088221767,2.40742996414767));
#80489=CARTESIAN_POINT('Ctrl Pts',(17.359819608922,1.97153860638563,2.40243847387899));
#80490=CARTESIAN_POINT('Ctrl Pts',(17.4205293379208,1.89650064017566,2.39744698361031));
#80491=CARTESIAN_POINT('Ctrl Pts',(17.4775219314432,1.81886979446515,2.39245549334163));
#80492=CARTESIAN_POINT('Ctrl Pts',(17.534609958825,1.7411089562284,2.38745564484339));
#80493=CARTESIAN_POINT('Ctrl Pts',(17.5879681735439,1.66074693078762,2.38245579634514));
#80494=CARTESIAN_POINT('Ctrl Pts',(17.6373729259274,1.57818449478665,2.3774559478469));
#80495=CARTESIAN_POINT('Ctrl Pts',(17.6770126431661,1.51194083482035,2.37344433821129));
#80496=CARTESIAN_POINT('Ctrl Pts',(17.7141081258761,1.4442812245987,2.36943272857568));
#80497=CARTESIAN_POINT('Ctrl Pts',(17.748566182052,1.37542218714116,2.36542111894007));
#80498=CARTESIAN_POINT('Ctrl Pts',(17.7915216125909,1.28958247565582,2.36042024430652));
#80499=CARTESIAN_POINT('Ctrl Pts',(17.8305268726252,1.20157879439895,2.35541936967296));
#80500=CARTESIAN_POINT('Ctrl Pts',(17.8653588069058,1.11180985680425,2.35041849503941));
#80501=CARTESIAN_POINT('Ctrl Pts',(17.9001436983387,1.02216215814038,2.34542437442022));
#80502=CARTESIAN_POINT('Ctrl Pts',(17.9307663087813,0.930754346975528,2.34043025380103));
#80503=CARTESIAN_POINT('Ctrl Pts',(17.9570498009236,0.838008785668726,2.33543613318183));
#80504=CARTESIAN_POINT('Ctrl Pts',(17.9833057073287,0.745360565105695,2.33044725412255));
#80505=CARTESIAN_POINT('Ctrl Pts',(18.005231429926,0.651377805421232,2.32545837506326));
#80506=CARTESIAN_POINT('Ctrl Pts',(18.0226989602409,0.556500894661161,2.32046949600397));
#80507=CARTESIAN_POINT('Ctrl Pts',(18.0401540885004,0.461691347098805,2.31548415907989));
#80508=CARTESIAN_POINT('Ctrl Pts',(18.0531572379258,0.365989340739401,2.31049882215582));
#80509=CARTESIAN_POINT('Ctrl Pts',(18.0616310358816,0.269847457142608,2.30551348523175));
#80510=CARTESIAN_POINT('Ctrl Pts',(18.070101780184,0.173740219640054,2.30052994484469));
#80511=CARTESIAN_POINT('Ctrl Pts',(18.0740463776682,0.0771938564023398,
2.29554640445763));
#80512=CARTESIAN_POINT('Ctrl Pts',(18.0734391959091,-0.0193328489793903,
2.29056286407058));
#80513=CARTESIAN_POINT('Ctrl Pts',(18.0728320674669,-0.11585107830551,2.28557976129056));
#80514=CARTESIAN_POINT('Ctrl Pts',(18.0676739574472,-0.212349214546744,
2.28059665851053));
#80515=CARTESIAN_POINT('Ctrl Pts',(18.0579913576166,-0.308368459383391,
2.27561355573051));
#80516=CARTESIAN_POINT('Ctrl Pts',(18.0483069690312,-0.404405442728394,
2.2706295323766));
#80517=CARTESIAN_POINT('Ctrl Pts',(18.0340964746571,-0.499962922521446,
2.26564550902268));
#80518=CARTESIAN_POINT('Ctrl Pts',(18.0154381165457,-0.594588273751947,
2.26066148566876));
#80519=CARTESIAN_POINT('Ctrl Pts',(17.9967597155873,-0.689315271731034,
2.25567210846662));
#80520=CARTESIAN_POINT('Ctrl Pts',(17.9736239974891,-0.783107711128687,
2.25068273126448));
#80521=CARTESIAN_POINT('Ctrl Pts',(17.9461600823604,-0.875524425191021,
2.24569335406234));
#80522=CARTESIAN_POINT('Ctrl Pts',(17.9186798879704,-0.967995919346955,
2.2407010194022));
#80523=CARTESIAN_POINT('Ctrl Pts',(17.8868665326475,-1.05908965050869,2.23570868474206));
#80524=CARTESIAN_POINT('Ctrl Pts',(17.8508979423385,-1.14838285095618,2.23071635008192));
#80525=CARTESIAN_POINT('Ctrl Pts',(17.8148717740528,-1.23781899061168,2.22571602376778));
#80526=CARTESIAN_POINT('Ctrl Pts',(17.774677272193,-1.32544844613389,2.22071569745364));
#80527=CARTESIAN_POINT('Ctrl Pts',(17.7305390600662,-1.41087160700504,2.2157153711395));
#80528=CARTESIAN_POINT('Ctrl Pts',(17.7060603665301,-1.45824659740661,2.21294223082578));
#80529=CARTESIAN_POINT('Ctrl Pts',(17.6803694935711,-1.50494347420096,2.21016909051206));
#80530=CARTESIAN_POINT('Ctrl Pts',(17.653510412745,-1.55089804289437,2.20739595019834));
#80531=CARTESIAN_POINT('Ctrl Pts',(17.6050747227622,-1.63376913058891,2.2023950730133));
#80532=CARTESIAN_POINT('Ctrl Pts',(17.5526686296632,-1.71451359020438,2.19739419582825));
#80533=CARTESIAN_POINT('Ctrl Pts',(17.4965042006414,-1.79272670147452,2.19239331864321));
#80534=CARTESIAN_POINT('Ctrl Pts',(17.4404156255765,-1.87083418051327,2.18739919548965));
#80535=CARTESIAN_POINT('Ctrl Pts',(17.3805790565024,-1.94641675259952,2.18240507233609));
#80536=CARTESIAN_POINT('Ctrl Pts',(17.3172516710118,-2.01909557554691,2.17741094918253));
#80537=CARTESIAN_POINT('Ctrl Pts',(17.2539907507559,-2.09169811846171,2.17242206760914));
#80538=CARTESIAN_POINT('Ctrl Pts',(17.1872465842831,-2.16140264186641,2.16743318603574));
#80539=CARTESIAN_POINT('Ctrl Pts',(17.1173181210884,-2.22786135657286,2.16244430446235));
#80540=CARTESIAN_POINT('Ctrl Pts',(17.0474393080759,-2.29427288466681,2.15745896506431));
#80541=CARTESIAN_POINT('Ctrl Pts',(16.9743810100404,-2.35744288416394,2.15247362566628));
#80542=CARTESIAN_POINT('Ctrl Pts',(16.8984800503645,-2.41705931833873,2.14748828626824));
#80543=CARTESIAN_POINT('Ctrl Pts',(16.8226064430564,-2.47665426858703,2.14250474343296));
#80544=CARTESIAN_POINT('Ctrl Pts',(16.7438925541852,-2.53269792729628,2.13752120059768));
#80545=CARTESIAN_POINT('Ctrl Pts',(16.6627086657526,-2.58491820815115,2.1325376577624));
#80546=CARTESIAN_POINT('Ctrl Pts',(16.5815319065773,-2.63713390322139,2.12755455256272));
#80547=CARTESIAN_POINT('Ctrl Pts',(16.497885948157,-2.68552665086909,2.12257144736304));
#80548=CARTESIAN_POINT('Ctrl Pts',(16.4121695582981,-2.72986801670265,2.11758834216336));
#80549=CARTESIAN_POINT('Ctrl Pts',(16.3264373338193,-2.77421757383632,2.11260431642122));
#80550=CARTESIAN_POINT('Ctrl Pts',(16.2386343079239,-2.81451406124734,2.10762029067908));
#80551=CARTESIAN_POINT('Ctrl Pts',(16.1491823467888,-2.85057576356584,2.10263626493694));
#80552=CARTESIAN_POINT('Ctrl Pts',(16.0596342973297,-2.88667620297287,2.09764688540854));
#80553=CARTESIAN_POINT('Ctrl Pts',(15.9684341840563,-2.9185326116556,2.09265750588014));
#80554=CARTESIAN_POINT('Ctrl Pts',(15.8760220683032,-2.94601214964327,2.08766812635174));
#80555=CARTESIAN_POINT('Ctrl Pts',(15.7835551757941,-2.9735079759708,2.08267578939699));
#80556=CARTESIAN_POINT('Ctrl Pts',(15.6898752760018,-2.99662166072452,2.07768345244225));
#80557=CARTESIAN_POINT('Ctrl Pts',(15.5954336797639,-3.01527129509151,2.07269111548751));
#80558=CARTESIAN_POINT('Ctrl Pts',(15.500840904271,-3.03395078322995,2.06769078695054));
#80559=CARTESIAN_POINT('Ctrl Pts',(15.4054844312867,-3.04815188815817,2.06269045841358));
#80560=CARTESIAN_POINT('Ctrl Pts',(15.3098216838575,-3.0578444653402,2.05769012987661));
#80561=CARTESIAN_POINT('Ctrl Pts',(15.2567683880726,-3.06321984058265,2.05491701373661));
#80562=CARTESIAN_POINT('Ctrl Pts',(15.2036209243158,-3.0672094732637,2.0521438975966));
#80563=CARTESIAN_POINT('Ctrl Pts',(15.1504570807384,-3.06981512747196,2.0493707814566));
#80564=CARTESIAN_POINT('Ctrl Pts',(15.0545843771295,-3.07451401861313,2.04436989882898));
#80565=CARTESIAN_POINT('Ctrl Pts',(14.9583240901873,-3.07472553622669,2.03936901620135));
#80566=CARTESIAN_POINT('Ctrl Pts',(14.8621310646495,-3.07040622828077,2.03436813357373));
#80567=CARTESIAN_POINT('Ctrl Pts',(14.7660679534245,-3.0660927538131,2.02937400493088));
#80568=CARTESIAN_POINT('Ctrl Pts',(14.6700723575853,-3.05726063493976,2.02437987628803));
#80569=CARTESIAN_POINT('Ctrl Pts',(14.5746020880084,-3.04391834096665,2.01938574764518));
#80570=CARTESIAN_POINT('Ctrl Pts',(14.4792320183685,-3.03059005027459,2.01439686054379));
#80571=CARTESIAN_POINT('Ctrl Pts',(14.3843866110825,-3.01276105520946,2.0094079734424));
#80572=CARTESIAN_POINT('Ctrl Pts',(14.2905204849002,-2.99049177689118,2.00441908634101));
#80573=CARTESIAN_POINT('Ctrl Pts',(14.1967210042557,-2.96823830990006,1.99943374138073));
#80574=CARTESIAN_POINT('Ctrl Pts',(14.1038998480948,-2.94155092800557,1.99444839642044));
#80575=CARTESIAN_POINT('Ctrl Pts',(14.0125023773816,-2.91054130623893,1.98946305146016));
#80576=CARTESIAN_POINT('Ctrl Pts',(13.9211378431163,-2.87954285925408,1.98447950304362));
#80577=CARTESIAN_POINT('Ctrl Pts',(13.8311963898972,-2.84422540803508,1.97949595462709));
#80578=CARTESIAN_POINT('Ctrl Pts',(13.7431081927623,-2.80475047640585,1.97451240621055));
#80579=CARTESIAN_POINT('Ctrl Pts',(13.6550277309741,-2.7652790112147,1.96952929541762));
#80580=CARTESIAN_POINT('Ctrl Pts',(13.5688006019236,-2.72165097107885,1.96454618462469));
#80581=CARTESIAN_POINT('Ctrl Pts',(13.4848359778387,-2.67407558530942,1.95956307383176));
#80582=CARTESIAN_POINT('Ctrl Pts',(13.4008558426759,-2.62649141077304,1.9545790424914));
#80583=CARTESIAN_POINT('Ctrl Pts',(13.3191394241955,-2.57495865865483,1.94959501115103));
#80584=CARTESIAN_POINT('Ctrl Pts',(13.2400693798354,-2.51973142660226,1.94461097981066));
#80585=CARTESIAN_POINT('Ctrl Pts',(13.1609143998115,-2.4644448704194,1.93962159471068));
#80586=CARTESIAN_POINT('Ctrl Pts',(13.0844118291418,-2.4054561632609,1.9346322096107));
#80587=CARTESIAN_POINT('Ctrl Pts',(13.0109133258318,-2.34306134205798,1.92964282451072));
#80588=CARTESIAN_POINT('Ctrl Pts',(12.9373712568537,-2.28062953680839,1.92465048199139));
#80589=CARTESIAN_POINT('Ctrl Pts',(12.8668371213099,-2.21478789660277,1.91965813947206));
#80590=CARTESIAN_POINT('Ctrl Pts',(12.7996260617113,-2.14586970287109,1.91466579695273));
#80591=CARTESIAN_POINT('Ctrl Pts',(12.7323074136824,-2.07684118800574,1.90966546291685));
#80592=CARTESIAN_POINT('Ctrl Pts',(12.6683227538112,-2.00472661410948,1.90466512888096));
#80593=CARTESIAN_POINT('Ctrl Pts',(12.6079472049745,-1.92989265914212,1.89966479484507));
#80594=CARTESIAN_POINT('Ctrl Pts',(12.5744644293987,-1.88839161165023,1.89689173413501));
#80595=CARTESIAN_POINT('Ctrl Pts',(12.5420908874423,-1.84605474329759,1.89411867342494));
#80596=CARTESIAN_POINT('Ctrl Pts',(12.5108675917382,-1.80294817012053,1.89134561271488));
#80597=CARTESIAN_POINT('Ctrl Pts',(12.4541870026739,-1.72469550956294,1.88631159208979));
#80598=CARTESIAN_POINT('Ctrl Pts',(12.4011017867308,-1.64363183337957,1.8812775714647));
#80599=CARTESIAN_POINT('Ctrl Pts',(12.3519001953372,-1.56011848093183,1.87624355083961));
#80600=CARTESIAN_POINT('Ctrl Pts',(12.3027665260435,-1.47672041748381,1.87121647960866));
#80601=CARTESIAN_POINT('Ctrl Pts',(12.2575060428062,-1.39087976641773,1.86618940837772));
#80602=CARTESIAN_POINT('Ctrl Pts',(12.2163652628411,-1.30298883344488,1.86116233714677));
#80603=CARTESIAN_POINT('Ctrl Pts',(12.1752705752684,-1.21519636976166,1.85614089803414));
#80604=CARTESIAN_POINT('Ctrl Pts',(12.1382865969624,-1.12535857852669,1.8511194589215));
#80605=CARTESIAN_POINT('Ctrl Pts',(12.1056147224448,-1.03389366719782,1.84609801980887));
#80606=CARTESIAN_POINT('Ctrl Pts',(12.0729730496365,-0.942513305552657,
1.84108122248818));
#80607=CARTESIAN_POINT('Ctrl Pts',(12.0446356948167,-0.849509220498868,
1.83606442516749));
#80608=CARTESIAN_POINT('Ctrl Pts',(12.0207561451115,-0.755320000469499,
1.8310476278468));
#80609=CARTESIAN_POINT('Ctrl Pts',(11.9968896807392,-0.661182393528222,
1.82603357959232));
#80610=CARTESIAN_POINT('Ctrl Pts',(11.9774762692274,-0.565861359986251,
1.82101953133784));
#80611=CARTESIAN_POINT('Ctrl Pts',(11.96261946134,-0.469810295086867,1.81600548308336));
#80612=CARTESIAN_POINT('Ctrl Pts',(11.9477647807859,-0.373772983654849,
1.81099215278603));
#80613=CARTESIAN_POINT('Ctrl Pts',(11.9374654783482,-0.277006273422207,
1.80597882248871));
#80614=CARTESIAN_POINT('Ctrl Pts',(11.9317737860968,-0.179972637690354,
1.80096549219138));
#80615=CARTESIAN_POINT('Ctrl Pts',(11.9282206620398,-0.11939793859866,1.7978358457351));
#80616=CARTESIAN_POINT('Ctrl Pts',(11.9264621300047,-0.0587193777735862,
1.79470619927883));
#80617=CARTESIAN_POINT('Ctrl Pts',(11.9265006184833,0.00194982479121544,
1.79157655282255));
#80618=CARTESIAN_POINT('Origin',(15.,0.,8.20842344717745));
#80619=CARTESIAN_POINT('',(16.8723108164276,2.43738680900022,3.43723392788203));
#80620=CARTESIAN_POINT('',(16.8723108164276,2.43738680900022,3.35426497682436));
#80621=CARTESIAN_POINT('',(16.8723108164276,2.43738680900022,8.20842344717745));
#80622=CARTESIAN_POINT('',(11.9265007775872,0.00218628177021425,2.70842344717746));
#80623=CARTESIAN_POINT('Ctrl Pts',(16.8723108164276,2.43738680900022,3.35426497682436));
#80624=CARTESIAN_POINT('Ctrl Pts',(16.9487990501378,2.37863136371089,3.34927201212424));
#80625=CARTESIAN_POINT('Ctrl Pts',(17.0224461613876,2.31632796124631,3.34427904742411));
#80626=CARTESIAN_POINT('Ctrl Pts',(17.0929223199439,2.25079506234593,3.33928608272398));
#80627=CARTESIAN_POINT('Ctrl Pts',(17.1635078534999,2.1851604601043,3.3342853692259));
#80628=CARTESIAN_POINT('Ctrl Pts',(17.2309123057041,2.11628667045165,3.32928465572782));
#80629=CARTESIAN_POINT('Ctrl Pts',(17.2948444052853,2.04452718385714,3.32428394222975));
#80630=CARTESIAN_POINT('Ctrl Pts',(17.3193712199737,2.01699748216784,3.32236547601198));
#80631=CARTESIAN_POINT('Ctrl Pts',(17.3433874196244,1.98904339107765,3.32044700979421));
#80632=CARTESIAN_POINT('Ctrl Pts',(17.3668782451022,1.96068600822823,3.31852854357645));
#80633=CARTESIAN_POINT('Ctrl Pts',(17.428111909547,1.88676666181879,3.31352766709645));
#80634=CARTESIAN_POINT('Ctrl Pts',(17.4859862459092,1.80984705629152,3.30852679061646));
#80635=CARTESIAN_POINT('Ctrl Pts',(17.540193809841,1.73026519887715,3.30352591413646));
#80636=CARTESIAN_POINT('Ctrl Pts',(17.5943281628246,1.65079082209502,3.29853179167533));
#80637=CARTESIAN_POINT('Ctrl Pts',(17.6448053409217,1.56866169897679,3.29353766921419));
#80638=CARTESIAN_POINT('Ctrl Pts',(17.6913576793253,1.48424933617532,3.28854354675306));
#80639=CARTESIAN_POINT('Ctrl Pts',(17.7378611588566,1.39992556812542,3.28355466585873));
#80640=CARTESIAN_POINT('Ctrl Pts',(17.7804477770603,1.31332370643703,3.2785657849644));
#80641=CARTESIAN_POINT('Ctrl Pts',(17.8188933647738,1.22484384638785,3.27357690407007));
#80642=CARTESIAN_POINT('Ctrl Pts',(17.8573116557536,1.13642680788265,3.26859156532873));
#80643=CARTESIAN_POINT('Ctrl Pts',(17.8915945869304,1.04613482298226,3.26360622658738));
#80644=CARTESIAN_POINT('Ctrl Pts',(17.9215645623794,0.954391302270142,3.25862088784604));
#80645=CARTESIAN_POINT('Ctrl Pts',(17.9515237376556,0.862680842842486,3.25363734565339));
#80646=CARTESIAN_POINT('Ctrl Pts',(17.977172909325,0.769520303512664,3.24865380346074));
#80647=CARTESIAN_POINT('Ctrl Pts',(17.9983834837999,0.675350822962396,3.24367026126809));
#80648=CARTESIAN_POINT('Ctrl Pts',(18.0195921957061,0.581189611737178,3.23868715669631));
#80649=CARTESIAN_POINT('Ctrl Pts',(18.0363629891924,0.486020063444048,3.23370405212454));
#80650=CARTESIAN_POINT('Ctrl Pts',(18.0486180445656,0.39029510418242,3.22872094755276));
#80651=CARTESIAN_POINT('Ctrl Pts',(18.0608753638864,0.294552461092729,3.22373692242312));
#80652=CARTESIAN_POINT('Ctrl Pts',(18.0686152326411,0.198254638372426,3.21875289729347));
#80653=CARTESIAN_POINT('Ctrl Pts',(18.0718116384515,0.101860236961538,3.21376887216383));
#80654=CARTESIAN_POINT('Ctrl Pts',(18.0750114778239,0.00536228919936145,
3.208779493221));
#80655=CARTESIAN_POINT('Ctrl Pts',(18.073658096343,-0.0912320052277161,
3.20379011427817));
#80656=CARTESIAN_POINT('Ctrl Pts',(18.0677776329475,-0.187463715921185,
3.19880073533534));
#80657=CARTESIAN_POINT('Ctrl Pts',(18.0618936839234,-0.283752467697744,
3.19380839895181));
#80658=CARTESIAN_POINT('Ctrl Pts',(18.0514773571495,-0.379677771915711,
3.18881606256827));
#80659=CARTESIAN_POINT('Ctrl Pts',(18.0366064918961,-0.474787598168444,
3.18382372618473));
#80660=CARTESIAN_POINT('Ctrl Pts',(18.0217118217248,-0.570049673907353,
3.17882339819108));
#80661=CARTESIAN_POINT('Ctrl Pts',(18.0023484632009,-0.664493235810517,
3.17382307019743));
#80662=CARTESIAN_POINT('Ctrl Pts',(17.978644976644,-0.757678264907645,3.16882274220378));
#80663=CARTESIAN_POINT('Ctrl Pts',(17.9654993048104,-0.809357574167647,
3.16604961974743));
#80664=CARTESIAN_POINT('Ctrl Pts',(17.9510196326832,-0.860650087983236,
3.16327649729108));
#80665=CARTESIAN_POINT('Ctrl Pts',(17.9352342955905,-0.911483340489089,
3.16050337483472));
#80666=CARTESIAN_POINT('Ctrl Pts',(17.9067680010694,-1.00315286447835,3.1555024983807));
#80667=CARTESIAN_POINT('Ctrl Pts',(17.8739535732588,-1.09364749386917,3.15050162192668));
#80668=CARTESIAN_POINT('Ctrl Pts',(17.8369061867942,-1.18252506837228,3.14550074547265));
#80669=CARTESIAN_POINT('Ctrl Pts',(17.7999088352689,-1.27128260784792,3.14050662303218));
#80670=CARTESIAN_POINT('Ctrl Pts',(17.7586900546112,-1.35842703147765,3.13551250059171));
#80671=CARTESIAN_POINT('Ctrl Pts',(17.7134148091021,-1.44353119943615,3.13051837815124));
#80672=CARTESIAN_POINT('Ctrl Pts',(17.6681870820484,-1.52854604665064,3.12552949727229));
#80673=CARTESIAN_POINT('Ctrl Pts',(17.6189115588135,-1.61152450989622,3.12054061639334));
#80674=CARTESIAN_POINT('Ctrl Pts',(17.5658009099349,-1.69206026505481,3.11555173551439));
#80675=CARTESIAN_POINT('Ctrl Pts',(17.512727970039,-1.77253883918726,3.1105663967805));
#80676=CARTESIAN_POINT('Ctrl Pts',(17.4558255585379,-1.85057778790208,3.10558105804662));
#80677=CARTESIAN_POINT('Ctrl Pts',(17.3953513163893,-1.92579706123772,3.10059571931274));
#80678=CARTESIAN_POINT('Ctrl Pts',(17.3348988670677,-2.00098922814678,3.09561217712265));
#80679=CARTESIAN_POINT('Ctrl Pts',(17.2708774192136,-2.07336339710243,3.09062863493255));
#80680=CARTESIAN_POINT('Ctrl Pts',(17.2035862312026,-2.142570879027,3.08564509274246));
#80681=CARTESIAN_POINT('Ctrl Pts',(17.1363009521811,-2.21177228368797,3.08066198816834));
#80682=CARTESIAN_POINT('Ctrl Pts',(17.0657468098319,-2.27780723983766,3.07567888359422));
#80683=CARTESIAN_POINT('Ctrl Pts',(16.9922606716825,-2.34036314833129,3.0706957790201));
#80684=CARTESIAN_POINT('Ctrl Pts',(16.9187609579395,-2.40293061320298,3.06571175388321));
#80685=CARTESIAN_POINT('Ctrl Pts',(16.8423285067147,-2.46201746966545,3.06072772874632));
#80686=CARTESIAN_POINT('Ctrl Pts',(16.7633332392227,-2.51735141318259,3.05574370360943));
#80687=CARTESIAN_POINT('Ctrl Pts',(16.6842531153189,-2.57274479620856,3.05075432465195));
#80688=CARTESIAN_POINT('Ctrl Pts',(16.6026050391149,-2.62437696616575,3.04576494569447));
#80689=CARTESIAN_POINT('Ctrl Pts',(16.5187876960584,-2.67201912124551,3.04077556673699));
#80690=CARTESIAN_POINT('Ctrl Pts',(16.4349206704307,-2.71968951612242,3.03578323033459));
#80691=CARTESIAN_POINT('Ctrl Pts',(16.3488822085863,-2.76336498837243,3.03079089393219));
#80692=CARTESIAN_POINT('Ctrl Pts',(16.2610934583573,-2.8028638103355,3.02579855752978));
#80693=CARTESIAN_POINT('Ctrl Pts',(16.1731641779293,-2.84242586109833,3.02079822951084));
#80694=CARTESIAN_POINT('Ctrl Pts',(16.0834794224651,-2.87779775104511,3.01579790149191));
#80695=CARTESIAN_POINT('Ctrl Pts',(15.9924779858168,-2.9088467985903,3.01079757347297));
#80696=CARTESIAN_POINT('Ctrl Pts',(15.9420096711571,-2.92606623115213,3.00802445101297));
#80697=CARTESIAN_POINT('Ctrl Pts',(15.891136628461,-2.94195699421057,3.00525132855297));
#80698=CARTESIAN_POINT('Ctrl Pts',(15.8399350346931,-2.95650323651018,3.00247820609297));
#80699=CARTESIAN_POINT('Ctrl Pts',(15.7476012654901,-2.98273502502342,2.99747732955086));
#80700=CARTESIAN_POINT('Ctrl Pts',(15.6538763853701,-3.00468295413782,2.99247645300875));
#80701=CARTESIAN_POINT('Ctrl Pts',(15.5591936696892,-3.02220196045525,2.98747557646664));
#80702=CARTESIAN_POINT('Ctrl Pts',(15.4646388293375,-3.03969730618494,2.98248145394219));
#80703=CARTESIAN_POINT('Ctrl Pts',(15.3691291521665,-3.05277553816698,2.97748733141774));
#80704=CARTESIAN_POINT('Ctrl Pts',(15.2731125303631,-3.06134150263551,2.9724932088933));
#80705=CARTESIAN_POINT('Ctrl Pts',(15.177196682505,-3.06989847672282,2.96750432793453));
#80706=CARTESIAN_POINT('Ctrl Pts',(15.080775382386,-3.07395255927076,2.96251544697577));
#80707=CARTESIAN_POINT('Ctrl Pts',(14.9843051467686,-3.07345992678968,2.95752656601701));
#80708=CARTESIAN_POINT('Ctrl Pts',(14.8879034059093,-3.07296764408222,2.95254122720979));
#80709=CARTESIAN_POINT('Ctrl Pts',(14.7914532360493,-3.06793506620663,2.94755588840257));
#80710=CARTESIAN_POINT('Ctrl Pts',(14.6954137119675,-3.0583703901167,2.94257054959536));
#80711=CARTESIAN_POINT('Ctrl Pts',(14.5994087972882,-3.04880916081317,2.93758700733596));
#80712=CARTESIAN_POINT('Ctrl Pts',(14.5038146704269,-3.03471912183679,2.93260346507656));
#80713=CARTESIAN_POINT('Ctrl Pts',(14.409086871846,-3.01616046074728,2.92761992281716));
#80714=CARTESIAN_POINT('Ctrl Pts',(14.3143673916023,-2.99760342935046,2.92263681817782));
#80715=CARTESIAN_POINT('Ctrl Pts',(14.2205145188283,-2.97457864058691,2.91765371353848));
#80716=CARTESIAN_POINT('Ctrl Pts',(14.1279741089871,-2.94719749854046,2.91267060889915));
#80717=CARTESIAN_POINT('Ctrl Pts',(14.0354166036046,-2.9198112982125,2.9076865837012));
#80718=CARTESIAN_POINT('Ctrl Pts',(13.9441724633098,-2.88806727078575,2.90270255850325));
#80719=CARTESIAN_POINT('Ctrl Pts',(13.8546718481927,-2.8521265179998,2.8977185333053));
#80720=CARTESIAN_POINT('Ctrl Pts',(13.7650750919802,-2.81614715784409,2.8927291542934));
#80721=CARTESIAN_POINT('Ctrl Pts',(13.6772260076248,-2.77596223628351,2.8877397752815));
#80722=CARTESIAN_POINT('Ctrl Pts',(13.591534029511,-2.73178071227809,2.8827503962696));
#80723=CARTESIAN_POINT('Ctrl Pts',(13.5057912577034,-2.68757299979087,2.87775805981645));
#80724=CARTESIAN_POINT('Ctrl Pts',(13.422208517895,-2.63936418685725,2.8727657233633));
#80725=CARTESIAN_POINT('Ctrl Pts',(13.3411680848319,-2.58740776206991,2.86777338691015));
#80726=CARTESIAN_POINT('Ctrl Pts',(13.259997924222,-2.53536816670624,2.86277305884669));
#80727=CARTESIAN_POINT('Ctrl Pts',(13.1813785536951,-2.47956923479637,2.85777273078323));
#80728=CARTESIAN_POINT('Ctrl Pts',(13.1056608056481,-2.42030602749783,2.85277240271977));
#80729=CARTESIAN_POINT('Ctrl Pts',(13.063668653474,-2.38743936567286,2.84999928093026));
#80730=CARTESIAN_POINT('Ctrl Pts',(13.022568326117,-2.35350789677246,2.84722615914075));
#80731=CARTESIAN_POINT('Ctrl Pts',(12.9824147133544,-2.31856676874125,2.84445303735124));
#80732=CARTESIAN_POINT('Ctrl Pts',(12.9110410684898,-2.2564583931385,2.83952377205846));
#80733=CARTESIAN_POINT('Ctrl Pts',(12.8423960887178,-2.19092748208239,2.83459450676568));
#80734=CARTESIAN_POINT('Ctrl Pts',(12.7768328506208,-2.12224646917393,2.82966524147289));
#80735=CARTESIAN_POINT('Ctrl Pts',(12.7096405802844,-2.05185895750933,2.82461350004392));
#80736=CARTESIAN_POINT('Ctrl Pts',(12.6456856417414,-1.97816296524106,2.81956175861494));
#80737=CARTESIAN_POINT('Ctrl Pts',(12.5853131208015,-1.90149665406668,2.81451001718596));
#80738=CARTESIAN_POINT('Ctrl Pts',(12.5265519994705,-1.82687663915281,2.80959311150735));
#80739=CARTESIAN_POINT('Ctrl Pts',(12.4711847807881,-1.74944324348275,2.80467620582875));
#80740=CARTESIAN_POINT('Ctrl Pts',(12.4194921084729,-1.66954522902682,2.79975930015014));
#80741=CARTESIAN_POINT('Ctrl Pts',(12.3678305275951,-1.58969527059142,2.79484535182813));
#80742=CARTESIAN_POINT('Ctrl Pts',(12.3198393500791,-1.5073840154634,2.78993140350612));
#80743=CARTESIAN_POINT('Ctrl Pts',(12.2757571653357,-1.4229909443774,2.78501745518411));
#80744=CARTESIAN_POINT('Ctrl Pts',(12.2316886534711,-1.33862404931331,2.78010503101115));
#80745=CARTESIAN_POINT('Ctrl Pts',(12.1915269348586,-1.25217702194179,2.77519260683818));
#80746=CARTESIAN_POINT('Ctrl Pts',(12.1554650790604,-1.16405469525924,2.77028018266522));
#80747=CARTESIAN_POINT('Ctrl Pts',(12.1176244835151,-1.07158576240239,2.76512545470791));
#80748=CARTESIAN_POINT('Ctrl Pts',(12.084298822646,-0.977272503217062,2.75997072675059));
#80749=CARTESIAN_POINT('Ctrl Pts',(12.0556539747487,-0.881605769937465,
2.75481599879328));
#80750=CARTESIAN_POINT('Ctrl Pts',(12.0283356592049,-0.790369327832824,
2.74989998438869));
#80751=CARTESIAN_POINT('Ctrl Pts',(12.0052743578697,-0.697902448005611,
2.7449839699841));
#80752=CARTESIAN_POINT('Ctrl Pts',(11.9865621544327,-0.604644193640178,
2.74006795557951));
#80753=CARTESIAN_POINT('Ctrl Pts',(11.9678412361408,-0.511342506006135,
2.73514965163416));
#80754=CARTESIAN_POINT('Ctrl Pts',(11.9534735149745,-0.417249157219473,
2.73023134768882));
#80755=CARTESIAN_POINT('Ctrl Pts',(11.9434993964955,-0.322810022732573,
2.72531304374347));
#80756=CARTESIAN_POINT('Ctrl Pts',(11.9335132389539,-0.228256897355436,
2.72038880325658));
#80757=CARTESIAN_POINT('Ctrl Pts',(11.9279312866406,-0.133357604235048,
2.71546456276969));
#80758=CARTESIAN_POINT('Ctrl Pts',(11.9267418836813,-0.038559051874358,
2.71054032228281));
#80759=CARTESIAN_POINT('Ctrl Pts',(11.9265714467364,-0.0249747779103842,
2.70983469724769));
#80760=CARTESIAN_POINT('Ctrl Pts',(11.926491118504,-0.0113925648463264,
2.70912907221258));
#80761=CARTESIAN_POINT('Ctrl Pts',(11.9265007775872,0.00218628177021425,
2.70842344717746));
#80762=CARTESIAN_POINT('Ctrl Pts',(11.9237226922662,0.00218825791429551,
2.70842344717746));
#80763=CARTESIAN_POINT('Ctrl Pts',(11.9225818664433,0.14340888213774,2.70109158765481));
#80764=CARTESIAN_POINT('Ctrl Pts',(11.9953557666493,1.29803405602119,2.64108467188491));
#80765=CARTESIAN_POINT('Ctrl Pts',(13.4561116265877,3.28204067332613,2.52840269986777));
#80766=CARTESIAN_POINT('Ctrl Pts',(15.8744262025005,3.14463381132417,2.41762058301274));
#80767=CARTESIAN_POINT('Ctrl Pts',(16.7921285915167,2.50458207762493,2.35951352240495));
#80768=CARTESIAN_POINT('Ctrl Pts',(16.8745674052796,2.44028174751842,2.35408151804441));
#80769=CARTESIAN_POINT('',(11.9265010538313,-0.00254517192390105,2.79157655284934));
#80770=CARTESIAN_POINT('Ctrl Pts',(11.9265010538309,-0.00254517140556233,
2.79157655282255));
#80771=CARTESIAN_POINT('Ctrl Pts',(11.9264216029999,0.0933980899065408,
2.7866185005732));
#80772=CARTESIAN_POINT('Ctrl Pts',(11.9308389262345,0.18941702310935,2.78166044832386));
#80773=CARTESIAN_POINT('Ctrl Pts',(11.9397475440067,0.285056407727899,2.77670239607451));
#80774=CARTESIAN_POINT('Ctrl Pts',(11.9486532096028,0.380664098956192,2.77174598684583));
#80775=CARTESIAN_POINT('Ctrl Pts',(11.9620471721085,0.475892049971424,2.76678957761714));
#80776=CARTESIAN_POINT('Ctrl Pts',(11.9798719422631,0.570288317319068,2.76183316838845));
#80777=CARTESIAN_POINT('Ctrl Pts',(11.9976957965019,0.664679734166605,2.75687701384212));
#80778=CARTESIAN_POINT('Ctrl Pts',(12.019949922976,0.758239116294989,2.75192085929579));
#80779=CARTESIAN_POINT('Ctrl Pts',(12.0465255813558,0.850524019892715,2.74696470474945));
#80780=CARTESIAN_POINT('Ctrl Pts',(12.0731073154434,0.942830021598326,2.74200741713065));
#80781=CARTESIAN_POINT('Ctrl Pts',(12.1040124203163,1.03386053986693,2.73705012951185));
#80782=CARTESIAN_POINT('Ctrl Pts',(12.1390824255821,1.12318871183192,2.73209284189306));
#80783=CARTESIAN_POINT('Ctrl Pts',(12.1741916518084,1.21261678502838,2.72713001023225));
#80784=CARTESIAN_POINT('Ctrl Pts',(12.2134749116354,1.30033829888587,2.72216717857144));
#80785=CARTESIAN_POINT('Ctrl Pts',(12.256725873535,1.38594708306904,2.71720434691064));
#80786=CARTESIAN_POINT('Ctrl Pts',(12.3000047118528,1.47161104443597,2.71223831657019));
#80787=CARTESIAN_POINT('Ctrl Pts',(12.347256123295,1.55515918055392,2.70727228622975));
#80788=CARTESIAN_POINT('Ctrl Pts',(12.3982292736095,1.6362124975985,2.70230625588931));
#80789=CARTESIAN_POINT('Ctrl Pts',(12.4492835184772,1.71739476454095,2.69733232495789));
#80790=CARTESIAN_POINT('Ctrl Pts',(12.5040710654416,1.79607392841595,2.69235839402647));
#80791=CARTESIAN_POINT('Ctrl Pts',(12.5622996527535,1.87190257947215,2.68738446309506));
#80792=CARTESIAN_POINT('Ctrl Pts',(12.5853736915098,1.90195093396744,2.68541346087122));
#80793=CARTESIAN_POINT('Ctrl Pts',(12.6089876478043,1.93155207612388,2.68344245864738));
#80794=CARTESIAN_POINT('Ctrl Pts',(12.6331217549488,1.96068600828974,2.68147145642354));
#80795=CARTESIAN_POINT('Ctrl Pts',(12.6943554201245,2.03460535557759,2.67647057988345));
#80796=CARTESIAN_POINT('Ctrl Pts',(12.759162058285,2.10578234896022,2.67146970334336));
#80797=CARTESIAN_POINT('Ctrl Pts',(12.8272667762959,2.17385201626343,2.66646882680326));
#80798=CARTESIAN_POINT('Ctrl Pts',(12.8952795143374,2.2418297509354,2.66147470428089));
#80799=CARTESIAN_POINT('Ctrl Pts',(12.9665811718247,2.30670819277677,2.65648058175851));
#80800=CARTESIAN_POINT('Ctrl Pts',(13.0408565389775,2.36815522065864,2.65148645923613));
#80801=CARTESIAN_POINT('Ctrl Pts',(13.1150539506503,2.42953775700402,2.64649757827947));
#80802=CARTESIAN_POINT('Ctrl Pts',(13.1922185311815,2.4874957608074,2.64150869732281));
#80803=CARTESIAN_POINT('Ctrl Pts',(13.2719988876619,2.5417345270028,2.63651981636615));
#80804=CARTESIAN_POINT('Ctrl Pts',(13.3517225993516,2.59593478317276,2.63153447756109));
#80805=CARTESIAN_POINT('Ctrl Pts',(13.4340580331092,2.64642080545337,2.62654913875604));
#80806=CARTESIAN_POINT('Ctrl Pts',(13.5186222214209,2.69293930996079,2.62156379995098));
#80807=CARTESIAN_POINT('Ctrl Pts',(13.6031559356531,2.7394410507691,2.61658025769378));
#80808=CARTESIAN_POINT('Ctrl Pts',(13.6899164246177,2.78197790344047,2.61159671543658));
#80809=CARTESIAN_POINT('Ctrl Pts',(13.7784941838012,2.8203414316342,2.60661317317938));
#80810=CARTESIAN_POINT('Ctrl Pts',(13.8670641647007,2.85870159100919,2.60163006854227));
#80811=CARTESIAN_POINT('Ctrl Pts',(13.9574506959103,2.89288898040133,2.59664696390515));
#80812=CARTESIAN_POINT('Ctrl Pts',(14.0492232431778,2.92274285709274,2.59166385926804));
#80813=CARTESIAN_POINT('Ctrl Pts',(14.1410127441345,2.95260224886859,2.58667983407233));
#80814=CARTESIAN_POINT('Ctrl Pts',(14.2341883525122,2.97812640235122,2.58169580887662));
#80815=CARTESIAN_POINT('Ctrl Pts',(14.3283043178312,2.99920442126837,2.57671178368091));
#80816=CARTESIAN_POINT('Ctrl Pts',(14.42252138203,3.0203050820837,2.57172240467128));
#80817=CARTESIAN_POINT('Ctrl Pts',(14.5176803909867,3.03694997767989,2.56673302566166));
#80818=CARTESIAN_POINT('Ctrl Pts',(14.6133255659997,3.04907939091302,2.56174364665203));
#80819=CARTESIAN_POINT('Ctrl Pts',(14.7090274344377,3.06121599382383,2.55675131020117));
#80820=CARTESIAN_POINT('Ctrl Pts',(14.8052156056642,3.06883175028921,2.5517589737503));
#80821=CARTESIAN_POINT('Ctrl Pts',(14.9014314598568,3.07191902446891,2.54676663729944));
#80822=CARTESIAN_POINT('Ctrl Pts',(14.9978013340396,3.07501124068175,2.54176630923828));
#80823=CARTESIAN_POINT('Ctrl Pts',(15.0941985414059,3.07356050695242,2.53676598117711));
#80824=CARTESIAN_POINT('Ctrl Pts',(15.1901668254077,3.06761125772389,2.53176565311594));
#80825=CARTESIAN_POINT('Ctrl Pts',(15.2433896816504,3.06431187564433,2.52899253130457));
#80826=CARTESIAN_POINT('Ctrl Pts',(15.2964807342468,3.05962981736536,2.52621940949319));
#80827=CARTESIAN_POINT('Ctrl Pts',(15.3493635103379,3.05357943856786,2.52344628768182));
#80828=CARTESIAN_POINT('Ctrl Pts',(15.4447236617431,3.0426691747573,2.5184456932474));
#80829=CARTESIAN_POINT('Ctrl Pts',(15.5397385953953,3.02726860088142,2.51344509881299));
#80830=CARTESIAN_POINT('Ctrl Pts',(15.6339525189152,3.00740859441499,2.50844450437857));
#80831=CARTESIAN_POINT('Ctrl Pts',(15.7280447702709,2.98757423606801,2.50345036794022));
#80832=CARTESIAN_POINT('Ctrl Pts',(15.8213376413766,2.96329197781237,2.49845623150185));
#80833=CARTESIAN_POINT('Ctrl Pts',(15.9133807516656,2.93464441670313,2.4934620950635));
#80834=CARTESIAN_POINT('Ctrl Pts',(16.0053187419076,2.90602957322977,2.48847366229872));
#80835=CARTESIAN_POINT('Ctrl Pts',(16.0960093935895,2.8730594723877,2.48348522953395));
#80836=CARTESIAN_POINT('Ctrl Pts',(16.1850140219671,2.83586741892873,2.47849679676917));
#80837=CARTESIAN_POINT('Ctrl Pts',(16.2739586339688,2.79870044430329,2.47351172773571));
#80838=CARTESIAN_POINT('Ctrl Pts',(16.3612190785803,2.75731734333633,2.46852665870225));
#80839=CARTESIAN_POINT('Ctrl Pts',(16.4463740661562,2.71190049794435,2.46354158966879));
#80840=CARTESIAN_POINT('Ctrl Pts',(16.5315057777478,2.6664960666435,2.45855788323771));
#80841=CARTESIAN_POINT('Ctrl Pts',(16.6145327864978,2.61706028285798,2.45357417680662));
#80842=CARTESIAN_POINT('Ctrl Pts',(16.6950567625211,2.56382230699233,2.44859047037553));
#80843=CARTESIAN_POINT('Ctrl Pts',(16.7556094151612,2.52378825975504,2.4448428083836));
#80844=CARTESIAN_POINT('Ctrl Pts',(16.8147470884424,2.48160514568058,2.44109514639167));
#80845=CARTESIAN_POINT('Ctrl Pts',(16.8723108164276,2.43738680900022,2.43734748439974));
#80846=CARTESIAN_POINT('Ctrl Pts',(16.8723108164276,2.43738680900022,3.43723392788203));
#80847=CARTESIAN_POINT('Ctrl Pts',(16.9512302592254,2.37676379839261,3.43208135302821));
#80848=CARTESIAN_POINT('Ctrl Pts',(17.0272819369425,2.31224276762403,3.4269287781744));
#80849=CARTESIAN_POINT('Ctrl Pts',(17.1000649707149,2.24413220839957,3.42177620332058));
#80850=CARTESIAN_POINT('Ctrl Pts',(17.1704753050321,2.17824202772195,3.41679160046401));
#80851=CARTESIAN_POINT('Ctrl Pts',(17.2378264618397,2.10899305298184,3.41180699760745));
#80852=CARTESIAN_POINT('Ctrl Pts',(17.301789126522,2.03670544434512,3.40682239475088));
#80853=CARTESIAN_POINT('Ctrl Pts',(17.3657344160622,1.96443747228039,3.40183914593706));
#80854=CARTESIAN_POINT('Ctrl Pts',(17.4262927521021,1.88913283495649,3.39685589712325));
#80855=CARTESIAN_POINT('Ctrl Pts',(17.4831730360029,1.81114712910573,3.39187264830943));
#80856=CARTESIAN_POINT('Ctrl Pts',(17.5400533715129,1.73316135249643,3.38688939497419));
#80857=CARTESIAN_POINT('Ctrl Pts',(17.5932553903981,1.65249485746842,3.38190614163894));
#80858=CARTESIAN_POINT('Ctrl Pts',(17.6425301527128,1.56953389323185,3.37692288830369));
#80859=CARTESIAN_POINT('Ctrl Pts',(17.6918183894875,1.4865502428547,3.37193827226989));
#80860=CARTESIAN_POINT('Ctrl Pts',(17.7371770124854,1.40127125400007,3.36695365623609));
#80861=CARTESIAN_POINT('Ctrl Pts',(17.7784025697423,1.31410859918402,3.36196904020229));
#80862=CARTESIAN_POINT('Ctrl Pts',(17.8196743521061,1.22684821123074,3.35697883505278));
#80863=CARTESIAN_POINT('Ctrl Pts',(17.8568036333464,1.13770033958764,3.35198862990328));
#80864=CARTESIAN_POINT('Ctrl Pts',(17.889634861312,1.04709723440101,3.34699842475377));
#80865=CARTESIAN_POINT('Ctrl Pts',(17.9224881621865,0.956433215437768,3.34200486461725));
#80866=CARTESIAN_POINT('Ctrl Pts',(17.9510375280809,0.864312433644861,3.33701130448073));
#80867=CARTESIAN_POINT('Ctrl Pts',(17.975177680863,0.771180923840089,3.33201774434421));
#80868=CARTESIAN_POINT('Ctrl Pts',(17.9993542688009,0.677908849014769,3.32701664733982));
#80869=CARTESIAN_POINT('Ctrl Pts',(18.0191082754717,0.583623430262389,3.32201555033544));
#80870=CARTESIAN_POINT('Ctrl Pts',(18.0343857991061,0.488779165046244,3.31701445333105));
#80871=CARTESIAN_POINT('Ctrl Pts',(18.0378910403734,0.467018306391696,3.3158670126842));
#80872=CARTESIAN_POINT('Ctrl Pts',(18.0411608484674,0.445228040187508,3.31471957203734));
#80873=CARTESIAN_POINT('Ctrl Pts',(18.0441949589413,0.423413866041879,3.31357213139049));
#80874=CARTESIAN_POINT('Ctrl Pts',(18.0574184878613,0.32834140076324,3.30857125396422));
#80875=CARTESIAN_POINT('Ctrl Pts',(18.0662070432973,0.232483017404805,3.30357037653796));
#80876=CARTESIAN_POINT('Ctrl Pts',(18.0704768138282,0.136287878197188,3.2985694991117));
#80877=CARTESIAN_POINT('Ctrl Pts',(18.0747408177609,0.0402226566778314,
3.29357537569027));
#80878=CARTESIAN_POINT('Ctrl Pts',(18.0744981468719,-0.0561779822314671,
3.28858125226883));
#80879=CARTESIAN_POINT('Ctrl Pts',(18.0697164401893,-0.152457295107154,
3.2835871288474));
#80880=CARTESIAN_POINT('Ctrl Pts',(18.0649397521201,-0.248635558570522,
3.27859824698016));
#80881=CARTESIAN_POINT('Ctrl Pts',(18.0556335204819,-0.344692313312812,
3.27360936511292));
#80882=CARTESIAN_POINT('Ctrl Pts',(18.0418174138874,-0.440169365779964,
3.26862048324569));
#80883=CARTESIAN_POINT('Ctrl Pts',(18.0280111168177,-0.535578628924582,
3.26363514351673));
#80884=CARTESIAN_POINT('Ctrl Pts',(18.0097013730412,-0.630408575110616,
3.25864980378777));
#80885=CARTESIAN_POINT('Ctrl Pts',(17.9869597261553,-0.724205664384442,
3.25366446405881));
#80886=CARTESIAN_POINT('Ctrl Pts',(17.9642262745538,-0.817968952507546,
3.24868092086982));
#80887=CARTESIAN_POINT('Ctrl Pts',(17.9370641964582,-0.910699697378456,
3.24369737768082));
#80888=CARTESIAN_POINT('Ctrl Pts',(17.9055960391893,-1.00195504242819,3.23871383449183));
#80889=CARTESIAN_POINT('Ctrl Pts',(17.8741306451927,-1.09320237419135,3.23373072891621));
#80890=CARTESIAN_POINT('Ctrl Pts',(17.8383600670373,-1.1829741490899,3.2287476233406));
#80891=CARTESIAN_POINT('Ctrl Pts',(17.7984562393385,-1.27084417868895,3.22376451776498));
#80892=CARTESIAN_POINT('Ctrl Pts',(17.7585450399249,-1.35873044113655,3.21878049162523));
#80893=CARTESIAN_POINT('Ctrl Pts',(17.714499255917,-1.44471386115675,3.21379646548547));
#80894=CARTESIAN_POINT('Ctrl Pts',(17.6665378745369,-1.52839066133637,3.20881243934572));
#80895=CARTESIAN_POINT('Ctrl Pts',(17.6185249732746,-1.61215734672715,3.20382305938936));
#80896=CARTESIAN_POINT('Ctrl Pts',(17.5665882962256,-1.69361208458467,3.19883367943301));
#80897=CARTESIAN_POINT('Ctrl Pts',(17.5109913654501,-1.77237823633529,3.19384429947665));
#80898=CARTESIAN_POINT('Ctrl Pts',(17.4553614797148,-1.85119107655109,3.18885196207617));
#80899=CARTESIAN_POINT('Ctrl Pts',(17.3960672896008,-1.92731181151864,3.1838596246757));
#80900=CARTESIAN_POINT('Ctrl Pts',(17.3334126674274,-2.00039685399905,3.17886728727522));
#80901=CARTESIAN_POINT('Ctrl Pts',(17.2706577493435,-2.07359888913899,3.17386695826921));
#80902=CARTESIAN_POINT('Ctrl Pts',(17.2045319589979,-2.14375520994463,3.16886662926321));
#80903=CARTESIAN_POINT('Ctrl Pts',(17.1353759985662,-2.21055911360623,3.1638663002572));
#80904=CARTESIAN_POINT('Ctrl Pts',(17.0970230700705,-2.2476076243112,3.16109318772105));
#80905=CARTESIAN_POINT('Ctrl Pts',(17.0577387654674,-2.28362575726213,3.15832007518491));
#80906=CARTESIAN_POINT('Ctrl Pts',(17.01758528669,-2.31856676870264,3.15554696264876));
#80907=CARTESIAN_POINT('Ctrl Pts',(16.9451747419857,-2.38157744045409,3.15054608612742));
#80908=CARTESIAN_POINT('Ctrl Pts',(16.8696832447064,-2.44130263317381,3.14554520960607));
#80909=CARTESIAN_POINT('Ctrl Pts',(16.7914412364284,-2.49742678499768,3.14054433308473));
#80910=CARTESIAN_POINT('Ctrl Pts',(16.7133048991478,-2.55347513744941,3.13555021057726));
#80911=CARTESIAN_POINT('Ctrl Pts',(16.6324257872682,-2.60593186144669,3.1305560880698));
#80912=CARTESIAN_POINT('Ctrl Pts',(16.5491687979154,-2.65452034943514,3.12556196556233));
#80913=CARTESIAN_POINT('Ctrl Pts',(16.4659991906131,-2.70305784156442,3.12057308461678));
#80914=CARTESIAN_POINT('Ctrl Pts',(16.3804570441074,-2.74773494872369,3.11558420367123));
#80915=CARTESIAN_POINT('Ctrl Pts',(16.2929368919671,-2.78831785192979,3.11059532272568));
#80916=CARTESIAN_POINT('Ctrl Pts',(16.2054788798438,-2.82887194094588,3.10560998392601));
#80917=CARTESIAN_POINT('Ctrl Pts',(16.1160460508533,-2.86533742089797,3.10062464512633));
#80918=CARTESIAN_POINT('Ctrl Pts',(16.0250573779798,-2.89752646611713,3.09563930632666));
#80919=CARTESIAN_POINT('Ctrl Pts',(15.9341014942885,-2.92970391151363,3.0906557640713));
#80920=CARTESIAN_POINT('Ctrl Pts',(15.8415912938814,-2.9576078380647,3.08567222181594));
#80921=CARTESIAN_POINT('Ctrl Pts',(15.7479646625862,-2.98109897747832,3.08068867956058));
#80922=CARTESIAN_POINT('Ctrl Pts',(15.6543462528656,-3.00458805407979,3.07570557492177));
#80923=CARTESIAN_POINT('Ctrl Pts',(15.5596120327128,-3.02366500743946,3.07072247028296));
#80924=CARTESIAN_POINT('Ctrl Pts',(15.4642129048914,-3.03824104194059,3.06573936564415));
#80925=CARTESIAN_POINT('Ctrl Pts',(15.3687961533535,-3.0528197691697,3.06075534044322));
#80926=CARTESIAN_POINT('Ctrl Pts',(15.2727146838301,-3.0628958599669,3.05577131524229));
#80927=CARTESIAN_POINT('Ctrl Pts',(15.1764263303416,-3.06843217294471,3.05078729004136));
#80928=CARTESIAN_POINT('Ctrl Pts',(15.0800345443018,-3.07397443300704,3.04579791102115));
#80929=CARTESIAN_POINT('Ctrl Pts',(14.9834358692918,-3.074967154573,3.04080853200095));
#80930=CARTESIAN_POINT('Ctrl Pts',(14.8870897351376,-3.07142532419212,3.03581915298074));
#80931=CARTESIAN_POINT('Ctrl Pts',(14.7906864920082,-3.06788139439849,3.03082681651627));
#80932=CARTESIAN_POINT('Ctrl Pts',(14.6945365247006,-3.05979759740087,3.02583448005179));
#80933=CARTESIAN_POINT('Ctrl Pts',(14.5990936205754,-3.04724077239339,3.02084214358732));
#80934=CARTESIAN_POINT('Ctrl Pts',(14.5034979336912,-3.03466384671539,3.0158418155079));
#80935=CARTESIAN_POINT('Ctrl Pts',(14.4086120013494,-3.0175996735953,3.01084148742848));
#80936=CARTESIAN_POINT('Ctrl Pts',(14.3148788347279,-2.99616609000505,3.00584115934905));
#80937=CARTESIAN_POINT('Ctrl Pts',(14.2628955478462,-2.98427928232712,3.00306803753504));
#80938=CARTESIAN_POINT('Ctrl Pts',(14.2112665472188,-2.97104947544008,3.00029491572103));
#80939=CARTESIAN_POINT('Ctrl Pts',(14.1600649653834,-2.95650323653191,2.99752179390702));
#80940=CARTESIAN_POINT('Ctrl Pts',(14.0677311973554,-2.93027144835505,2.99252091742801));
#80941=CARTESIAN_POINT('Ctrl Pts',(13.976466386845,-2.8996642779387,2.98752004094901));
#80942=CARTESIAN_POINT('Ctrl Pts',(13.886715360663,-2.86478612845989,2.98251916447001));
#80943=CARTESIAN_POINT('Ctrl Pts',(13.7970855492583,-2.82995508426004,2.97752504200993));
#80944=CARTESIAN_POINT('Ctrl Pts',(13.7089658642828,-2.7908646827843,2.97253091954985));
#80945=CARTESIAN_POINT('Ctrl Pts',(13.6227873256133,-2.7476694669317,2.96753679708977));
#80946=CARTESIAN_POINT('Ctrl Pts',(13.5366992353812,-2.70451958649365,2.96254791619655));
#80947=CARTESIAN_POINT('Ctrl Pts',(13.4525486314016,-2.65727365182197,2.95755903530334));
#80948=CARTESIAN_POINT('Ctrl Pts',(13.3707468824896,-2.60613440349547,2.95257015441012));
#80949=CARTESIAN_POINT('Ctrl Pts',(13.2890032136005,-2.5550314645236,2.94758481566998));
#80950=CARTESIAN_POINT('Ctrl Pts',(13.2096054553147,-2.50004093914038,2.94259947692984));
#80951=CARTESIAN_POINT('Ctrl Pts',(13.1329398021085,-2.44141116312865,2.9376141381897));
#80952=CARTESIAN_POINT('Ctrl Pts',(13.0563017766302,-2.38280251532021,2.9326305959983));
#80953=CARTESIAN_POINT('Ctrl Pts',(12.9823942480704,-2.32055748890506,2.92764705380689));
#80954=CARTESIAN_POINT('Ctrl Pts',(12.9115730699147,-2.25496678638391,2.92266351161549));
#80955=CARTESIAN_POINT('Ctrl Pts',(12.8407581107952,-2.189381843594,2.91768040704502));
#80956=CARTESIAN_POINT('Ctrl Pts',(12.7730292849172,-2.12045210706759,2.91269730247454));
#80957=CARTESIAN_POINT('Ctrl Pts',(12.7087072797838,-2.04850675378045,2.90771419790406));
#80958=CARTESIAN_POINT('Ctrl Pts',(12.6443733920732,-1.97654810961079,2.90273017277576));
#80959=CARTESIAN_POINT('Ctrl Pts',(12.5834478673824,-1.90157306932208,2.89774614764746));
#80960=CARTESIAN_POINT('Ctrl Pts',(12.5262119131704,-1.82394483235097,2.89276212251917));
#80961=CARTESIAN_POINT('Ctrl Pts',(12.4689144764028,-1.74623320754331,2.88777274357776));
#80962=CARTESIAN_POINT('Ctrl Pts',(12.4153147830547,-1.66586304998148,2.88278336463635));
#80963=CARTESIAN_POINT('Ctrl Pts',(12.3656512492023,-1.58322737128015,2.87779398569494));
#80964=CARTESIAN_POINT('Ctrl Pts',(12.3159582774265,-1.50054271050704,2.87280164931286));
#80965=CARTESIAN_POINT('Ctrl Pts',(12.2702063187608,-1.41559024069342,2.86780931293078));
#80966=CARTESIAN_POINT('Ctrl Pts',(12.2285872744958,-1.3287865723709,2.86281697654869));
#80967=CARTESIAN_POINT('Ctrl Pts',(12.1869016074819,-1.24184395085775,2.85781664855655));
#80968=CARTESIAN_POINT('Ctrl Pts',(12.1493622354496,-1.15304461762709,2.85281632056441));
#80969=CARTESIAN_POINT('Ctrl Pts',(12.1161124565978,-1.06282401507016,2.84781599257226));
#80970=CARTESIAN_POINT('Ctrl Pts',(12.0976725244638,-1.01278874128219,2.84504287010327));
#80971=CARTESIAN_POINT('Ctrl Pts',(12.080551041576,-0.962316593232633,2.84226974763428));
#80972=CARTESIAN_POINT('Ctrl Pts',(12.0647657044095,-0.911483340489195,
2.83949662516529));
#80973=CARTESIAN_POINT('Ctrl Pts',(12.0303090566219,-0.800523183781246,
2.83344338074116));
#80974=CARTESIAN_POINT('Ctrl Pts',(12.0021241467251,-0.687529803949023,
2.82739013631703));
#80975=CARTESIAN_POINT('Ctrl Pts',(11.9804132908884,-0.573147761189416,
2.8213368918929));
#80976=CARTESIAN_POINT('Ctrl Pts',(11.9589656931388,-0.460152674246049,
2.81535704694966));
#80977=CARTESIAN_POINT('Ctrl Pts',(11.9438361316593,-0.345802413645502,
2.80937720200641));
#80978=CARTESIAN_POINT('Ctrl Pts',(11.9351734469449,-0.230738921052811,
2.80339735706317));
#80979=CARTESIAN_POINT('Ctrl Pts',(11.9294653892418,-0.15492073340149,2.79945708899189));
#80980=CARTESIAN_POINT('Ctrl Pts',(11.9265641950853,-0.0787932931996348,
2.79551682092061));
#80981=CARTESIAN_POINT('Ctrl Pts',(11.9265010538313,-0.00254517192389286,
2.79157655284934));
#80982=CARTESIAN_POINT('Origin',(15.,0.,8.20842344717745));
#80983=CARTESIAN_POINT('',(16.8744034286678,2.4401532777456,4.43742370379915));
#80984=CARTESIAN_POINT('',(16.8723108164276,2.43738680900022,4.35414769597494));
#80985=CARTESIAN_POINT('',(16.8723108164276,2.43738680900022,8.20842344717745));
#80986=CARTESIAN_POINT('',(11.926500046528,0.00053479698373032,3.70842344715139));
#80987=CARTESIAN_POINT('Ctrl Pts',(16.8723108164276,2.43738680900022,4.35414769597494));
#80988=CARTESIAN_POINT('Ctrl Pts',(16.9488483750057,2.37859347416326,4.34916459568889));
#80989=CARTESIAN_POINT('Ctrl Pts',(17.022627942246,2.31618088767149,4.34418149540283));
#80990=CARTESIAN_POINT('Ctrl Pts',(17.0932982724848,2.25044542089165,4.33919839511677));
#80991=CARTESIAN_POINT('Ctrl Pts',(17.1639761185111,2.18470296314693,4.33421476487815));
#80992=CARTESIAN_POINT('Ctrl Pts',(17.231543749874,2.11563722236728,4.32923113463953));
#80993=CARTESIAN_POINT('Ctrl Pts',(17.295685840847,2.04358233749817,4.32424750440091));
#80994=CARTESIAN_POINT('Ctrl Pts',(17.3598940064996,1.97145322674465,4.31925874037626));
#80995=CARTESIAN_POINT('Ctrl Pts',(17.420669291915,1.89632915049203,4.3142699763516));
#80996=CARTESIAN_POINT('Ctrl Pts',(17.4777359811466,1.81857819676022,4.30928121232694));
#80997=CARTESIAN_POINT('Ctrl Pts',(17.5348324844232,1.74078662265126,4.30428984196157));
#80998=CARTESIAN_POINT('Ctrl Pts',(17.5882162894751,1.66036580309245,4.2992984715962));
#80999=CARTESIAN_POINT('Ctrl Pts',(17.6376556431944,1.57771193756179,4.29430710123082));
#81000=CARTESIAN_POINT('Ctrl Pts',(17.687178382336,1.4949186663356,4.28930731231838));
#81001=CARTESIAN_POINT('Ctrl Pts',(17.7327431714415,1.40988521179885,4.28430752340594));
#81002=CARTESIAN_POINT('Ctrl Pts',(17.7741646975999,1.32303154935572,4.2793077344935));
#81003=CARTESIAN_POINT('Ctrl Pts',(17.809038064846,1.24990822561668,4.27509834167129));
#81004=CARTESIAN_POINT('Ctrl Pts',(17.8409753984857,1.17549521079981,4.27088894884907));
#81005=CARTESIAN_POINT('Ctrl Pts',(17.8698934162568,1.1000518302907,4.26667955602686));
#81006=CARTESIAN_POINT('Ctrl Pts',(17.9042487347892,1.01042323302418,4.26167869350647));
#81007=CARTESIAN_POINT('Ctrl Pts',(17.9344612304041,0.919027319678192,4.25667783098609));
#81008=CARTESIAN_POINT('Ctrl Pts',(17.9603478056003,0.826282711835128,4.25167696846571));
#81009=CARTESIAN_POINT('Ctrl Pts',(17.9861994180126,0.733663366204382,4.24668286018277));
#81010=CARTESIAN_POINT('Ctrl Pts',(18.007736605184,0.639699365344247,4.24168875189983));
#81011=CARTESIAN_POINT('Ctrl Pts',(18.0248246780298,0.544828337352284,4.23669464361689));
#81012=CARTESIAN_POINT('Ctrl Pts',(18.0418948154112,0.450056885008856,4.23170577709828));
#81013=CARTESIAN_POINT('Ctrl Pts',(18.054525044472,0.35438072756338,4.22671691057968));
#81014=CARTESIAN_POINT('Ctrl Pts',(18.0626310335647,0.258250657784551,4.22172804406108));
#81015=CARTESIAN_POINT('Ctrl Pts',(18.0707312669298,0.162188845993797,4.21674271993032));
#81016=CARTESIAN_POINT('Ctrl Pts',(18.0743136099195,0.065674198492784,4.21175739579957));
#81017=CARTESIAN_POINT('Ctrl Pts',(18.0733453163882,-0.0308353082480665,
4.20677207166882));
#81018=CARTESIAN_POINT('Ctrl Pts',(18.0723773718256,-0.12731003339422,4.20178854422659));
#81019=CARTESIAN_POINT('Ctrl Pts',(18.0668620537893,-0.223779183249446,
4.19680501678437));
#81020=CARTESIAN_POINT('Ctrl Pts',(18.0568187148435,-0.319783668411212,
4.19182148934214));
#81021=CARTESIAN_POINT('Ctrl Pts',(18.0467762580836,-0.415779720739623,
4.18683839964255));
#81022=CARTESIAN_POINT('Ctrl Pts',(18.0322066170607,-0.511310753255124,
4.18185530994296));
#81023=CARTESIAN_POINT('Ctrl Pts',(18.013181020168,-0.605922758855491,4.17687222024337));
#81024=CARTESIAN_POINT('Ctrl Pts',(17.9941519089521,-0.700552240763099,
4.17188821008969));
#81025=CARTESIAN_POINT('Ctrl Pts',(17.9706652937107,-0.794261928563089,
4.16690419993602));
#81026=CARTESIAN_POINT('Ctrl Pts',(17.9428433014491,-0.88660901930666,4.16192018978235));
#81027=CARTESIAN_POINT('Ctrl Pts',(17.9149914232404,-0.97905530784485,4.15693082588325));
#81028=CARTESIAN_POINT('Ctrl Pts',(17.8827949977367,-1.07013565659585,4.15194146198414));
#81029=CARTESIAN_POINT('Ctrl Pts',(17.8464256657073,-1.15942364112636,4.14695209808503));
#81030=CARTESIAN_POINT('Ctrl Pts',(17.8100347762303,-1.24876454994617,4.14195977680549));
#81031=CARTESIAN_POINT('Ctrl Pts',(17.7694662395117,-1.33631058130578,4.13696745552595));
#81032=CARTESIAN_POINT('Ctrl Pts',(17.7249384690705,-1.42165839419308,4.13197513424641));
#81033=CARTESIAN_POINT('Ctrl Pts',(17.6803394189777,-1.50714283108624,4.12697482130418));
#81034=CARTESIAN_POINT('Ctrl Pts',(17.6317687010872,-1.59042164471374,4.12197450836195));
#81035=CARTESIAN_POINT('Ctrl Pts',(17.579488938003,-1.67111910668276,4.11697419541973));
#81036=CARTESIAN_POINT('Ctrl Pts',(17.5504935795652,-1.71587546548723,4.11420092604153));
#81037=CARTESIAN_POINT('Ctrl Pts',(17.5203580550293,-1.75983835100493,4.11142765666333));
#81038=CARTESIAN_POINT('Ctrl Pts',(17.4891324099213,-1.80294816782937,4.10865438728513));
#81039=CARTESIAN_POINT('Ctrl Pts',(17.4328249414843,-1.88068570189063,4.10365350491937));
#81040=CARTESIAN_POINT('Ctrl Pts',(17.3727740527321,-1.95591853085914,4.0986526225536));
#81041=CARTESIAN_POINT('Ctrl Pts',(17.3092303728174,-2.02826461174513,4.09365174018784));
#81042=CARTESIAN_POINT('Ctrl Pts',(17.2457725119616,-2.10051298546995,4.08865761177492));
#81043=CARTESIAN_POINT('Ctrl Pts',(17.1788315222906,-2.16988203288277,4.08366348336201));
#81044=CARTESIAN_POINT('Ctrl Pts',(17.1087003964975,-2.23601987643477,4.0786693549491));
#81045=CARTESIAN_POINT('Ctrl Pts',(17.0386428757322,-2.30208830604593,4.07368046804567));
#81046=CARTESIAN_POINT('Ctrl Pts',(16.9654021923812,-2.36493197416687,4.06869158114224));
#81047=CARTESIAN_POINT('Ctrl Pts',(16.8893098741311,-2.42423399231814,4.06370269423881));
#81048=CARTESIAN_POINT('Ctrl Pts',(16.8132715811698,-2.48349390623696,4.05871734942822));
#81049=CARTESIAN_POINT('Ctrl Pts',(16.7343860233073,-2.53921690019619,4.05373200461763));
#81050=CARTESIAN_POINT('Ctrl Pts',(16.6530189243427,-2.59112537052238,4.04874665980704));
#81051=CARTESIAN_POINT('Ctrl Pts',(16.5716811467436,-2.64301513516479,4.04376311151025));
#81052=CARTESIAN_POINT('Ctrl Pts',(16.487863974313,-2.69109287173475,4.03877956321347));
#81053=CARTESIAN_POINT('Ctrl Pts',(16.4019625223432,-2.73512400741631,4.03379601491669));
#81054=CARTESIAN_POINT('Ctrl Pts',(16.3160686131762,-2.77915127682831,4.02881290421346));
#81055=CARTESIAN_POINT('Ctrl Pts',(16.2280911788234,-2.81913245191646,4.02382979351022));
#81056=CARTESIAN_POINT('Ctrl Pts',(16.1384494151317,-2.85487918819455,4.01884668280699));
#81057=CARTESIAN_POINT('Ctrl Pts',(16.048791091061,-2.89063252830858,4.01386265152614));
#81058=CARTESIAN_POINT('Ctrl Pts',(15.957468234481,-2.92214971355348,4.00887862024528));
#81059=CARTESIAN_POINT('Ctrl Pts',(15.8649184602626,-2.9492911533277,4.00389458896443));
#81060=CARTESIAN_POINT('Ctrl Pts',(15.7722692698296,-2.97646174821571,3.99890520387772));
#81061=CARTESIAN_POINT('Ctrl Pts',(15.6783909522895,-2.99924709033049,3.99391581879102));
#81062=CARTESIAN_POINT('Ctrl Pts',(15.5837344509653,-3.01755800950972,3.98892643370431));
#81063=CARTESIAN_POINT('Ctrl Pts',(15.4890218422372,-3.03587978244039,3.9839340911721));
#81064=CARTESIAN_POINT('Ctrl Pts',(15.3935305651652,-3.04972178852117,3.97894174863989));
#81065=CARTESIAN_POINT('Ctrl Pts',(15.2977177781436,-3.05904664472074,3.97394940610768));
#81066=CARTESIAN_POINT('Ctrl Pts',(15.2017516175532,-3.06838642780554,3.96894907201803));
#81067=CARTESIAN_POINT('Ctrl Pts',(15.1054633571565,-3.0731946012312,3.96394873792838));
#81068=CARTESIAN_POINT('Ctrl Pts',(15.0093111762828,-3.0734858958512,3.95894840383872));
#81069=CARTESIAN_POINT('Ctrl Pts',(14.9559875519744,-3.07364744065173,3.95617534207361));
#81070=CARTESIAN_POINT('Ctrl Pts',(14.90270572017,-3.07242073058102,3.9534022803085));
#81071=CARTESIAN_POINT('Ctrl Pts',(14.8495429190397,-3.06981512746108,3.95062921854339));
#81072=CARTESIAN_POINT('Ctrl Pts',(14.7536703234448,-3.06511624160693,3.94562834154831));
#81073=CARTESIAN_POINT('Ctrl Pts',(14.6578508137849,-3.05591359805995,3.94062746455323));
#81074=CARTESIAN_POINT('Ctrl Pts',(14.5625413030582,-3.04220843113518,3.93562658755814));
#81075=CARTESIAN_POINT('Ctrl Pts',(14.4673605136946,-3.02852177388226,3.93063246455538));
#81076=CARTESIAN_POINT('Ctrl Pts',(14.3726887848571,-3.01034474086119,3.92563834155262));
#81077=CARTESIAN_POINT('Ctrl Pts',(14.2789809042196,-2.98773052893329,3.92064421854986));
#81078=CARTESIAN_POINT('Ctrl Pts',(14.1853713739254,-2.96514005156742,3.91565533708824));
#81079=CARTESIAN_POINT('Ctrl Pts',(14.0927241049829,-2.9381217556984,3.91066645562662));
#81080=CARTESIAN_POINT('Ctrl Pts',(14.0014856279963,-2.90678022886182,3.90567757416501));
#81081=CARTESIAN_POINT('Ctrl Pts',(13.9103119305315,-2.87546095457913,3.90069223482034));
#81082=CARTESIAN_POINT('Ctrl Pts',(13.8205454502547,-2.8398246935631,3.89570689547568));
#81083=CARTESIAN_POINT('Ctrl Pts',(13.7326184923474,-2.80002613631733,3.89072155613101));
#81084=CARTESIAN_POINT('Ctrl Pts',(13.6447232199693,-2.76024192095689,3.88573801331291));
#81085=CARTESIAN_POINT('Ctrl Pts',(13.5586665520638,-2.71629857036273,3.88075447049481));
#81086=CARTESIAN_POINT('Ctrl Pts',(13.4748608060477,-2.66839889991558,3.8757709276767));
#81087=CARTESIAN_POINT('Ctrl Pts',(13.3910624189226,-2.62050343548613,3.87078782245805));
#81088=CARTESIAN_POINT('Ctrl Pts',(13.3095149414523,-2.56865255978706,3.8658047172394));
#81089=CARTESIAN_POINT('Ctrl Pts',(13.2306051238602,-2.51309451121327,3.86082161202074));
#81090=CARTESIAN_POINT('Ctrl Pts',(13.1516807284728,-2.45752619884866,3.8558375862235));
#81091=CARTESIAN_POINT('Ctrl Pts',(13.0753953193757,-2.39824960601306,3.85085356042627));
#81092=CARTESIAN_POINT('Ctrl Pts',(13.0021048714653,-2.33555503154548,3.84586953462903));
#81093=CARTESIAN_POINT('Ctrl Pts',(12.9287356949499,-2.27279311056099,3.84088015499089));
#81094=CARTESIAN_POINT('Ctrl Pts',(12.8583682361594,-2.20660616374052,3.83589077535274));
#81095=CARTESIAN_POINT('Ctrl Pts',(12.7913235179395,-2.1373231968032,3.83090139571459));
#81096=CARTESIAN_POINT('Ctrl Pts',(12.7242390589276,-2.06799916235066,3.82590905861903));
#81097=CARTESIAN_POINT('Ctrl Pts',(12.6604815519403,-1.99557578271777,3.82091672152347));
#81098=CARTESIAN_POINT('Ctrl Pts',(12.6003320372269,-1.9204155587894,3.81592438442791));
#81099=CARTESIAN_POINT('Ctrl Pts',(12.5400862364191,-1.845135019935,3.81092405570278));
#81100=CARTESIAN_POINT('Ctrl Pts',(12.4834602174762,-1.76710924381181,3.80592372697764));
#81101=CARTESIAN_POINT('Ctrl Pts',(12.4306919269981,-1.68673005427879,3.80092339825251));
#81102=CARTESIAN_POINT('Ctrl Pts',(12.4014273312902,-1.64215281928218,3.79815028210222));
#81103=CARTESIAN_POINT('Ctrl Pts',(12.3733484337038,-1.59685221060393,3.79537716595194));
#81104=CARTESIAN_POINT('Ctrl Pts',(12.3464895869019,-1.55089804229029,3.79260404980166));
#81105=CARTESIAN_POINT('Ctrl Pts',(12.2962687235998,-1.46497261064162,3.78741885744656));
#81106=CARTESIAN_POINT('Ctrl Pts',(12.2501518247339,-1.37648008503504,3.78223366509146));
#81107=CARTESIAN_POINT('Ctrl Pts',(12.2083991234112,-1.28583311352156,3.77704847273635));
#81108=CARTESIAN_POINT('Ctrl Pts',(12.1667175851587,-1.19534064019856,3.77187211799406));
#81109=CARTESIAN_POINT('Ctrl Pts',(12.1293856045808,-1.10270138378311,3.76669576325176));
#81110=CARTESIAN_POINT('Ctrl Pts',(12.0966184712053,-1.00835407881036,3.76151940850946));
#81111=CARTESIAN_POINT('Ctrl Pts',(12.063916973894,-0.914195761555924,3.75635342255801));
#81112=CARTESIAN_POINT('Ctrl Pts',(12.0357622347784,-0.818336582006121,
3.75118743660656));
#81113=CARTESIAN_POINT('Ctrl Pts',(12.0123217486003,-0.721235686938343,
3.7460214506551));
#81114=CARTESIAN_POINT('Ctrl Pts',(11.9889093155104,-0.624251000209755,
3.74086164724859));
#81115=CARTESIAN_POINT('Ctrl Pts',(11.970200001538,-0.526027935410458,3.73570184384208));
#81116=CARTESIAN_POINT('Ctrl Pts',(11.9563118270862,-0.427041632706651,
3.73054204043557));
#81117=CARTESIAN_POINT('Ctrl Pts',(11.9424418566281,-0.328185076790691,
3.725389000267));
#81118=CARTESIAN_POINT('Ctrl Pts',(11.9333804921489,-0.228567664282163,
3.72023596009843));
#81119=CARTESIAN_POINT('Ctrl Pts',(11.9291947176724,-0.128674659621159,
3.71508291992986));
#81120=CARTESIAN_POINT('Ctrl Pts',(11.9273915716872,-0.0856427974625278,
3.71286309567906));
#81121=CARTESIAN_POINT('Ctrl Pts',(11.926492547944,-0.0425599106124228,
3.71064327142826));
#81122=CARTESIAN_POINT('Ctrl Pts',(11.9265000465279,0.000534796477657107,
3.70842344717746));
#81123=CARTESIAN_POINT('Ctrl Pts',(11.926500046528,0.000534796983736532,
3.70842344715139));
#81124=CARTESIAN_POINT('Ctrl Pts',(11.9265179259855,0.103288763884867,3.70313055243193));
#81125=CARTESIAN_POINT('Ctrl Pts',(11.9316930045359,0.205917075552153,3.69783765771246));
#81126=CARTESIAN_POINT('Ctrl Pts',(11.9419621490322,0.307907050987914,3.69254476299299));
#81127=CARTESIAN_POINT('Ctrl Pts',(11.9522653070746,0.410234838471516,3.68723433710346));
#81128=CARTESIAN_POINT('Ctrl Pts',(11.9676962419627,0.511919711507636,3.68192391121393));
#81129=CARTESIAN_POINT('Ctrl Pts',(11.9881402471583,0.612456593737547,3.6766134853244));
#81130=CARTESIAN_POINT('Ctrl Pts',(12.0086191925345,0.713165300264503,3.67129398355968));
#81131=CARTESIAN_POINT('Ctrl Pts',(12.034128220555,0.812721762062335,3.66597448179496));
#81132=CARTESIAN_POINT('Ctrl Pts',(12.0645027368102,0.910636078686353,3.66065498003023));
#81133=CARTESIAN_POINT('Ctrl Pts',(12.0949645851663,1.0088319162704,3.65532018375807));
#81134=CARTESIAN_POINT('Ctrl Pts',(12.1303197790766,1.1053758367413,3.64998538748591));
#81135=CARTESIAN_POINT('Ctrl Pts',(12.1703549949709,1.19979639752506,3.64465059121375));
#81136=CARTESIAN_POINT('Ctrl Pts',(12.1955495272369,1.25921613117943,3.64129335449581));
#81137=CARTESIAN_POINT('Ctrl Pts',(12.2225965524397,1.31779542095264,3.63793611777786));
#81138=CARTESIAN_POINT('Ctrl Pts',(12.2514338177412,1.3754221867278,3.63457888105992));
#81139=CARTESIAN_POINT('Ctrl Pts',(12.2943892720977,1.46126194584123,3.62957800365029));
#81140=CARTESIAN_POINT('Ctrl Pts',(12.3414447733354,1.54523722853729,3.62457712624066));
#81141=CARTESIAN_POINT('Ctrl Pts',(12.3924149664827,1.62693040508086,3.61957624883103));
#81142=CARTESIAN_POINT('Ctrl Pts',(12.4433163211217,1.70851324976051,3.61458212542644));
#81143=CARTESIAN_POINT('Ctrl Pts',(12.4981216295677,1.78781974491484,3.60958800202185));
#81144=CARTESIAN_POINT('Ctrl Pts',(12.5565988421315,1.86445515680238,3.60459387861725));
#81145=CARTESIAN_POINT('Ctrl Pts',(12.6150146802628,1.94101013642041,3.59960499676705));
#81146=CARTESIAN_POINT('Ctrl Pts',(12.677094496469,2.01489925900873,3.59461611491685));
#81147=CARTESIAN_POINT('Ctrl Pts',(12.7425625419643,2.08575606748667,3.58962723306665));
#81148=CARTESIAN_POINT('Ctrl Pts',(12.8079841047226,2.15656256717085,3.58464189335493));
#81149=CARTESIAN_POINT('Ctrl Pts',(12.8767888174963,2.22434071151225,3.57965655364321));
#81150=CARTESIAN_POINT('Ctrl Pts',(12.948660817216,2.2887572626155,3.57467121393149));
#81151=CARTESIAN_POINT('Ctrl Pts',(13.0205069168094,2.35315060027235,3.56968767075985));
#81152=CARTESIAN_POINT('Ctrl Pts',(13.0954177807538,2.41418445918998,3.56470412758821));
#81153=CARTESIAN_POINT('Ctrl Pts',(13.1730415652243,2.47156329629689,3.55972058441658));
#81154=CARTESIAN_POINT('Ctrl Pts',(13.2506585334171,2.52893709486964,3.55473747885842));
#81155=CARTESIAN_POINT('Ctrl Pts',(13.3309875955968,2.58265624918541,3.54975437330026));
#81156=CARTESIAN_POINT('Ctrl Pts',(13.4136456492958,2.63246692742794,3.54477126774211));
#81157=CARTESIAN_POINT('Ctrl Pts',(13.4963189729971,2.68228680754659,3.53978724161989));
#81158=CARTESIAN_POINT('Ctrl Pts',(13.5813217669772,2.72819655121854,3.53480321549767));
#81159=CARTESIAN_POINT('Ctrl Pts',(13.668244847156,2.76998744814366,3.52981918937546));
#81160=CARTESIAN_POINT('Ctrl Pts',(13.7552612996843,2.81182323664675,3.52482980943666));
#81161=CARTESIAN_POINT('Ctrl Pts',(13.8442017604325,2.84953115524765,3.51984042949785));
#81162=CARTESIAN_POINT('Ctrl Pts',(13.9346357166394,2.88295008519736,3.51485104955905));
#81163=CARTESIAN_POINT('Ctrl Pts',(14.0251232773767,2.916388824145,3.50985871217615));
#81164=CARTESIAN_POINT('Ctrl Pts',(14.1171056783353,2.94553337985266,3.50486637479326));
#81165=CARTESIAN_POINT('Ctrl Pts',(14.2101378756744,2.97027272730231,3.49987403741037));
#81166=CARTESIAN_POINT('Ctrl Pts',(14.3033189965691,2.99505167686489,3.49487370842182));
#81167=CARTESIAN_POINT('Ctrl Pts',(14.3975528408454,3.01541124538148,3.48987337943328));
#81168=CARTESIAN_POINT('Ctrl Pts',(14.4923849059777,3.03129166632324,3.48487305044474));
#81169=CARTESIAN_POINT('Ctrl Pts',(14.5449774465139,3.04009872626596,3.48209993773589));
#81170=CARTESIAN_POINT('Ctrl Pts',(14.5977538872124,3.04752907963788,3.47932682502704));
#81171=CARTESIAN_POINT('Ctrl Pts',(14.6506364897203,3.05357943857451,3.47655371231819));
#81172=CARTESIAN_POINT('Ctrl Pts',(14.7478038738911,3.06469646994753,3.47145834833928));
#81173=CARTESIAN_POINT('Ctrl Pts',(14.8456751428802,3.07119073221958,3.46636298436037));
#81174=CARTESIAN_POINT('Ctrl Pts',(14.9437730708905,3.07298564631254,3.46126762038146));
#81175=CARTESIAN_POINT('Ctrl Pts',(15.0399040776467,3.07474457132041,3.45627442145242));
#81176=CARTESIAN_POINT('Ctrl Pts',(15.1362522756829,3.07199079458058,3.45128122252339));
#81177=CARTESIAN_POINT('Ctrl Pts',(15.232360432918,3.06470404431066,3.44628802359435));
#81178=CARTESIAN_POINT('Ctrl Pts',(15.3283766492337,3.05742426483843,3.44129960135975));
#81179=CARTESIAN_POINT('Ctrl Pts',(15.4241528461465,3.04562016087953,3.43631117912515));
#81180=CARTESIAN_POINT('Ctrl Pts',(15.5192316013898,3.02932348786295,3.43132275689055));
#81181=CARTESIAN_POINT('Ctrl Pts',(15.6142453186025,3.01303796248409,3.42633774695513));
#81182=CARTESIAN_POINT('Ctrl Pts',(15.7085621113835,2.99226605011536,3.4213527370197));
#81183=CARTESIAN_POINT('Ctrl Pts',(15.8017305545386,2.96709123013083,3.41636772708428));
#81184=CARTESIAN_POINT('Ctrl Pts',(15.8984541423936,2.94095578308408,3.41119249789595));
#81185=CARTESIAN_POINT('Ctrl Pts',(15.9939394997286,2.91007475332913,3.40601726870763));
#81186=CARTESIAN_POINT('Ctrl Pts',(16.0876947952964,2.87459949945817,3.4008420395193));
#81187=CARTESIAN_POINT('Ctrl Pts',(16.1779764290032,2.84043861439844,3.39585855412683));
#81188=CARTESIAN_POINT('Ctrl Pts',(16.2666535061744,2.80201811261858,3.39087506873436));
#81189=CARTESIAN_POINT('Ctrl Pts',(16.3533052419485,2.75952299720708,3.38589158334189));
#81190=CARTESIAN_POINT('Ctrl Pts',(16.4399652523917,2.71702382379239,3.38090762205943));
#81191=CARTESIAN_POINT('Ctrl Pts',(16.5245991469185,2.67044946398176,3.37592366077698));
#81192=CARTESIAN_POINT('Ctrl Pts',(16.606810133319,2.62003119169666,3.37093969949453));
#81193=CARTESIAN_POINT('Ctrl Pts',(16.6890743805132,2.56958025568474,3.36595250932813));
#81194=CARTESIAN_POINT('Ctrl Pts',(16.768912220232,2.51528067766863,3.36096531916174));
#81195=CARTESIAN_POINT('Ctrl Pts',(16.8459558454969,2.45740702092184,3.35597812899535));
#81196=CARTESIAN_POINT('Ctrl Pts',(16.8547776101565,2.45078028473102,3.35540707827169));
#81197=CARTESIAN_POINT('Ctrl Pts',(16.8635627751665,2.44410673224555,3.35483602754802));
#81198=CARTESIAN_POINT('Ctrl Pts',(16.8723108164276,2.43738680900022,3.35426497682436));
#81199=CARTESIAN_POINT('',(11.9260286661608,0.000457056471357439,3.79157660457388));
#81200=CARTESIAN_POINT('Ctrl Pts',(11.9265000341218,0.000457981234923757,
3.79157655282255));
#81201=CARTESIAN_POINT('Ctrl Pts',(11.9265037802304,0.0255980166936363,
3.79026691442027));
#81202=CARTESIAN_POINT('Ctrl Pts',(11.9268159741402,0.0507354235207862,
3.78895727601798));
#81203=CARTESIAN_POINT('Ctrl Pts',(11.9274364573799,0.0758651867586845,
3.7876476376157));
#81204=CARTESIAN_POINT('Ctrl Pts',(11.9298057860042,0.171823729304893,3.7826467551499));
#81205=CARTESIAN_POINT('Ctrl Pts',(11.936678843721,0.267838568083366,3.7776458726841));
#81206=CARTESIAN_POINT('Ctrl Pts',(11.9480654915482,0.363452893950377,3.77264499021831));
#81207=CARTESIAN_POINT('Ctrl Pts',(11.9594367611156,0.458938087700323,3.76765086170423));
#81208=CARTESIAN_POINT('Ctrl Pts',(11.9753094540373,0.554023411679852,3.76265673319015));
#81209=CARTESIAN_POINT('Ctrl Pts',(11.995641432497,0.648252919678345,3.75766260467606));
#81210=CARTESIAN_POINT('Ctrl Pts',(12.0159520718507,0.742383530588454,3.7526737176705));
#81211=CARTESIAN_POINT('Ctrl Pts',(12.040712600613,0.835659684587091,3.74768483066494));
#81212=CARTESIAN_POINT('Ctrl Pts',(12.0698293049436,0.927632442205818,3.74269594365938));
#81213=CARTESIAN_POINT('Ctrl Pts',(12.0989253365193,1.01953989949872,3.73771059874558));
#81214=CARTESIAN_POINT('Ctrl Pts',(12.1323712630674,1.11014538307368,3.73272525383178));
#81215=CARTESIAN_POINT('Ctrl Pts',(12.1700229371203,1.19901295805135,3.72773990891797));
#81216=CARTESIAN_POINT('Ctrl Pts',(12.207661043059,1.28784850881123,3.72275636051737));
#81217=CARTESIAN_POINT('Ctrl Pts',(12.2495017141688,1.37494699183315,3.71777281211677));
#81218=CARTESIAN_POINT('Ctrl Pts',(12.2953522069319,1.45989128549082,3.71278926371617));
#81219=CARTESIAN_POINT('Ctrl Pts',(12.3411986736766,1.54482812039991,3.70780615290864));
#81220=CARTESIAN_POINT('Ctrl Pts',(12.3910540534722,1.62761075610814,3.70282304210111));
#81221=CARTESIAN_POINT('Ctrl Pts',(12.4446795723252,1.70784652762125,3.69783993129358));
#81222=CARTESIAN_POINT('Ctrl Pts',(12.4983149979361,1.78809712186014,3.69285589990806));
#81223=CARTESIAN_POINT('Ctrl Pts',(12.5557217020849,1.86579955277997,3.68787186852255));
#81224=CARTESIAN_POINT('Ctrl Pts',(12.6166181154014,1.94059090025874,3.68288783713703));
#81225=CARTESIAN_POINT('Ctrl Pts',(12.677579943147,2.01546258799133,3.67789845194576));
#81226=CARTESIAN_POINT('Ctrl Pts',(12.7420386862182,2.08741660883097,3.67290906675449));
#81227=CARTESIAN_POINT('Ctrl Pts',(12.8096732310118,2.15612404444959,3.66791968156322));
#81228=CARTESIAN_POINT('Ctrl Pts',(12.8773478660129,2.22487220622907,3.66292733892634));
#81229=CARTESIAN_POINT('Ctrl Pts',(12.9482017290782,2.2903696533319,3.65793499628946));
#81230=CARTESIAN_POINT('Ctrl Pts',(13.0218792503718,2.35232662483132,3.65294265365258));
#81231=CARTESIAN_POINT('Ctrl Pts',(13.0956747119036,2.4143827747484,3.64794231945912));
#81232=CARTESIAN_POINT('Ctrl Pts',(13.1723025083832,2.47288686685116,3.64294198526566));
#81233=CARTESIAN_POINT('Ctrl Pts',(13.251376709153,2.52759150906694,3.6379416510722));
#81234=CARTESIAN_POINT('Ctrl Pts',(13.2952292903294,2.55792934037148,3.63516859033945));
#81235=CARTESIAN_POINT('Ctrl Pts',(13.3398337948282,2.58709943598804,3.63239552960671));
#81236=CARTESIAN_POINT('Ctrl Pts',(13.3851212676778,2.61506576014706,3.62962246887396));
#81237=CARTESIAN_POINT('Ctrl Pts',(13.4667917043678,2.66549961664126,3.6246215918817));
#81238=CARTESIAN_POINT('Ctrl Pts',(13.5509695081239,2.71219184757326,3.61962071488944));
#81239=CARTESIAN_POINT('Ctrl Pts',(13.6372774368868,2.75488465565842,3.61461983789718));
#81240=CARTESIAN_POINT('Ctrl Pts',(13.7234688014811,2.79751980447922,3.60962571489701));
#81241=CARTESIAN_POINT('Ctrl Pts',(13.8117841835152,2.83616607287433,3.60463159189685));
#81242=CARTESIAN_POINT('Ctrl Pts',(13.901818658671,2.87060968986674,3.59963746889669));
#81243=CARTESIAN_POINT('Ctrl Pts',(13.9917586388803,2.90501715684283,3.59464858743745));
#81244=CARTESIAN_POINT('Ctrl Pts',(14.0834137178149,2.93523058519941,3.58965970597821));
#81245=CARTESIAN_POINT('Ctrl Pts',(14.1763566660133,2.96108323226133,3.58467082451897));
#81246=CARTESIAN_POINT('Ctrl Pts',(14.2692336245182,2.98691752388817,3.57968548517631));
#81247=CARTESIAN_POINT('Ctrl Pts',(14.3633962130629,3.0083970721192,3.57470014583365));
#81248=CARTESIAN_POINT('Ctrl Pts',(14.4584005449834,3.02540448210247,3.56971480649099));
#81249=CARTESIAN_POINT('Ctrl Pts',(14.5533706409624,3.04240576326319,3.56473126367468));
#81250=CARTESIAN_POINT('Ctrl Pts',(14.6491814462386,3.05493803109365,3.55974772085837));
#81251=CARTESIAN_POINT('Ctrl Pts',(14.7453782861762,3.06293487244659,3.55476417804206));
#81252=CARTESIAN_POINT('Ctrl Pts',(14.8415666791784,3.07093101160597,3.54978107282498));
#81253=CARTESIAN_POINT('Ctrl Pts',(14.9381406022654,3.07439247998299,3.54479796760791));
#81254=CARTESIAN_POINT('Ctrl Pts',(15.0346407212946,3.07330477994425,3.53981486239083));
#81255=CARTESIAN_POINT('Ctrl Pts',(15.131158667755,3.07221687896382,3.53483083659494));
#81256=CARTESIAN_POINT('Ctrl Pts',(15.2276023444474,3.06657814546016,3.52984681079905));
#81257=CARTESIAN_POINT('Ctrl Pts',(15.3235139544554,3.05642617631648,3.52486278500316));
#81258=CARTESIAN_POINT('Ctrl Pts',(15.4195285927294,3.04626330192602,3.519873405366));
#81259=CARTESIAN_POINT('Ctrl Pts',(15.515009586372,3.03157755956898,3.51488402572885));
#81260=CARTESIAN_POINT('Ctrl Pts',(15.6095060173364,3.01245824283602,3.50989464609169));
#81261=CARTESIAN_POINT('Ctrl Pts',(15.7040584611141,2.99332759311717,3.50490230899691));
#81262=CARTESIAN_POINT('Ctrl Pts',(15.797624755,2.96975824328842,3.49990997190213));
#81263=CARTESIAN_POINT('Ctrl Pts',(15.8897679576311,2.94188973817392,3.49491763480736));
#81264=CARTESIAN_POINT('Ctrl Pts',(15.9820586611939,2.9139766217332,3.48991730608268));
#81265=CARTESIAN_POINT('Ctrl Pts',(16.0729213118051,2.88175075522685,3.484916977358));
#81266=CARTESIAN_POINT('Ctrl Pts',(16.1619378719125,2.84540025863065,3.47991664863333));
#81267=CARTESIAN_POINT('Ctrl Pts',(16.211305278649,2.82524075405788,3.47714353246629));
#81268=CARTESIAN_POINT('Ctrl Pts',(16.2601052981254,2.80381348718193,3.47437041629926));
#81269=CARTESIAN_POINT('Ctrl Pts',(16.3082700746706,2.78115653312097,3.47159730013223));
#81270=CARTESIAN_POINT('Ctrl Pts',(16.3951353878213,2.74029465124967,3.46659597714205));
#81271=CARTESIAN_POINT('Ctrl Pts',(16.4802360276853,2.69528791493697,3.46159465415187));
#81272=CARTESIAN_POINT('Ctrl Pts',(16.5631498740513,2.64631153140617,3.45659333116168));
#81273=CARTESIAN_POINT('Ctrl Pts',(16.6459414432796,2.5974073757632,3.45159938386913));
#81274=CARTESIAN_POINT('Ctrl Pts',(16.7265522571003,2.54454543504667,3.44660543657658));
#81275=CARTESIAN_POINT('Ctrl Pts',(16.8045821065948,2.48794808437751,3.44161148928402));
#81276=CARTESIAN_POINT('Ctrl Pts',(16.8273817369834,2.47141084017433,3.44015230215002));
#81277=CARTESIAN_POINT('Ctrl Pts',(16.8499611681798,2.45455498600154,3.43869311501603));
#81278=CARTESIAN_POINT('Ctrl Pts',(16.8723108164276,2.43738680900022,3.43723392788203));
#81279=CARTESIAN_POINT('Ctrl Pts',(16.8744034286678,2.4401532777456,4.43742370379915));
#81280=CARTESIAN_POINT('Ctrl Pts',(16.9648833459027,2.37176298119687,4.43153190672698));
#81281=CARTESIAN_POINT('Ctrl Pts',(17.8240291038397,1.64081102949522,4.37296505340756));
#81282=CARTESIAN_POINT('Ctrl Pts',(18.5634164219284,-0.676361122770444,
4.2617231438409));
#81283=CARTESIAN_POINT('Ctrl Pts',(16.3800292810756,-3.35423176516155,4.10369797509917));
#81284=CARTESIAN_POINT('Ctrl Pts',(12.9727817450913,-2.99125903268367,3.94698262306987));
#81285=CARTESIAN_POINT('Ctrl Pts',(11.923704677711,-0.987130664284586,3.84294232728783));
#81286=CARTESIAN_POINT('Ctrl Pts',(11.9216277130479,0.000448422365026861,
3.79157708775303));
#81287=CARTESIAN_POINT('Origin',(15.,0.,8.20842344717745));
#81288=CARTESIAN_POINT('',(16.8723108164276,2.43738680900022,5.43736140735745));
#81289=CARTESIAN_POINT('',(16.8743174193178,2.43995797974749,5.35407234097178));
#81290=CARTESIAN_POINT('',(16.8723108164276,2.43738680900022,8.20842344717745));
#81291=CARTESIAN_POINT('',(11.9269509903871,-0.00352382680246899,5.79157674146509));
#81292=CARTESIAN_POINT('Ctrl Pts',(11.9265020164746,-0.00352069106647204,
5.79157655282255));
#81293=CARTESIAN_POINT('Ctrl Pts',(11.9263925964237,0.0920009834060071,
5.78664484566267));
#81294=CARTESIAN_POINT('Ctrl Pts',(11.9307405367531,0.18759836643084,5.78171313850279));
#81295=CARTESIAN_POINT('Ctrl Pts',(11.9395400315067,0.282819785817695,5.77678143134291));
#81296=CARTESIAN_POINT('Ctrl Pts',(11.948336955793,0.378013389568948,5.77185116481026));
#81297=CARTESIAN_POINT('Ctrl Pts',(11.9615828108053,0.472830801643596,5.76692089827761));
#81298=CARTESIAN_POINT('Ctrl Pts',(11.9792197838843,0.566823725618401,5.76199063174496));
#81299=CARTESIAN_POINT('Ctrl Pts',(11.996856650819,0.660816083917506,5.75706039488403));
#81300=CARTESIAN_POINT('Ctrl Pts',(12.0188844997887,0.753983523412695,5.7521301580231));
#81301=CARTESIAN_POINT('Ctrl Pts',(12.0451942965562,0.845887406748669,5.74719992116217));
#81302=CARTESIAN_POINT('Ctrl Pts',(12.0715114625849,0.937817031967794,5.74226830336306));
#81303=CARTESIAN_POINT('Ctrl Pts',(12.1021128339379,1.02848196754582,5.73733668556395));
#81304=CARTESIAN_POINT('Ctrl Pts',(12.1368397174184,1.11745937118419,5.73240506776485));
#81305=CARTESIAN_POINT('Ctrl Pts',(12.1716074489345,1.2065414358741,5.72746764907379));
#81306=CARTESIAN_POINT('Ctrl Pts',(12.2105102107563,1.29393159048697,5.72253023038273));
#81307=CARTESIAN_POINT('Ctrl Pts',(12.2533415748387,1.37922795269323,5.71759281169167));
#81308=CARTESIAN_POINT('Ctrl Pts',(12.296202926742,1.46458403403517,5.7126519361313));
#81309=CARTESIAN_POINT('Ctrl Pts',(12.3429981327611,1.54784301736527,5.70771106057094));
#81310=CARTESIAN_POINT('Ctrl Pts',(12.3934764629018,1.62863049847199,5.70277018501057));
#81311=CARTESIAN_POINT('Ctrl Pts',(12.444035586198,1.70954728408431,5.69782140132554));
#81312=CARTESIAN_POINT('Ctrl Pts',(12.4982893379946,1.78798431024768,5.69287261764051));
#81313=CARTESIAN_POINT('Ctrl Pts',(12.5559458884148,1.86359913866777,5.68792383395549));
#81314=CARTESIAN_POINT('Ctrl Pts',(12.5713797829185,1.88384022621544,5.6865991101425));
#81315=CARTESIAN_POINT('Ctrl Pts',(12.5870573023478,1.90387928819221,5.68527438632951));
#81316=CARTESIAN_POINT('Ctrl Pts',(12.6029724092414,1.92371021184119,5.68394966251652));
#81317=CARTESIAN_POINT('Ctrl Pts',(12.6631243299309,1.99866215244131,5.67894280442458));
#81318=CARTESIAN_POINT('Ctrl Pts',(12.7268987108395,2.07091920946328,5.67393594633263));
#81319=CARTESIAN_POINT('Ctrl Pts',(12.7940253727926,2.14011172468098,5.66892908824069));
#81320=CARTESIAN_POINT('Ctrl Pts',(12.8610613977209,2.20921081347866,5.6639289906029));
#81321=CARTESIAN_POINT('Ctrl Pts',(12.9314404049951,2.27525327353562,5.65892889296511));
#81322=CARTESIAN_POINT('Ctrl Pts',(13.0048514334962,2.33790171897317,5.65392879532732));
#81323=CARTESIAN_POINT('Ctrl Pts',(13.0781852825972,2.40048430006402,5.64893395445467));
#81324=CARTESIAN_POINT('Ctrl Pts',(13.154544484504,2.45967967806806,5.64393911358203));
#81325=CARTESIAN_POINT('Ctrl Pts',(13.2335813528962,2.51518735150369,5.63894427270938));
#81326=CARTESIAN_POINT('Ctrl Pts',(13.3125613934417,2.57065511468449,5.6339530231487));
#81327=CARTESIAN_POINT('Ctrl Pts',(13.3942149157232,2.62244019424737,5.62896177358803));
#81328=CARTESIAN_POINT('Ctrl Pts',(13.478162050998,2.67028303873904,5.62397052402735));
#81329=CARTESIAN_POINT('Ctrl Pts',(13.5620784131935,2.71810834514986,5.61898110414339));
#81330=CARTESIAN_POINT('Ctrl Pts',(13.6482863379862,2.76199407175551,5.61399168425942));
#81331=CARTESIAN_POINT('Ctrl Pts',(13.7363787410871,2.80172510500643,5.60900226437546));
#81332=CARTESIAN_POINT('Ctrl Pts',(13.8244626942452,2.84145232720278,5.60401332308341));
#81333=CARTESIAN_POINT('Ctrl Pts',(13.9144303674491,2.87702546882009,5.59902438179136));
#81334=CARTESIAN_POINT('Ctrl Pts',(14.0058529089589,2.90827677695479,5.59403544049932));
#81335=CARTESIAN_POINT('Ctrl Pts',(14.0972914245552,2.939533545571,5.58904562749906));
#81336=CARTESIAN_POINT('Ctrl Pts',(14.1901848993957,2.96646683949829,5.58405581449881));
#81337=CARTESIAN_POINT('Ctrl Pts',(14.2840884776609,2.98895850459355,5.57906600149856));
#81338=CARTESIAN_POINT('Ctrl Pts',(14.3780907208969,3.01147380179655,5.57407094567623));
#81339=CARTESIAN_POINT('Ctrl Pts',(14.4731047602957,3.02953805120322,5.56907588985389));
#81340=CARTESIAN_POINT('Ctrl Pts',(14.5686748998234,3.04308411121967,5.56408083403156));
#81341=CARTESIAN_POINT('Ctrl Pts',(14.6643005749494,3.05663804282186,5.55908287559325));
#81342=CARTESIAN_POINT('Ctrl Pts',(14.7604825583859,3.0656685156294,5.55408491715495));
#81343=CARTESIAN_POINT('Ctrl Pts',(14.8567614522654,3.07016041412218,5.54908695871664));
#81344=CARTESIAN_POINT('Ctrl Pts',(14.9531915603744,3.07465936752536,5.54408115055755));
#81345=CARTESIAN_POINT('Ctrl Pts',(15.0497184457063,3.0746055134796,5.53907534239846));
#81346=CARTESIAN_POINT('Ctrl Pts',(15.1458842162635,3.07003583781121,5.53406953423937));
#81347=CARTESIAN_POINT('Ctrl Pts',(15.1980419010702,3.06755737066225,5.53135452075118));
#81348=CARTESIAN_POINT('Ctrl Pts',(15.2500934603555,3.06375139340765,5.52863950726299));
#81349=CARTESIAN_POINT('Ctrl Pts',(15.3019669800779,3.05863011705284,5.5259244937748));
#81350=CARTESIAN_POINT('Ctrl Pts',(15.3976641489927,3.04918229760645,5.52091578980068));
#81351=CARTESIAN_POINT('Ctrl Pts',(15.4930781290478,3.03522313013419,5.51590708582656));
#81352=CARTESIAN_POINT('Ctrl Pts',(15.5877513814294,3.01677817607258,5.51089838185243));
#81353=CARTESIAN_POINT('Ctrl Pts',(15.6823057632538,2.9983563812657,5.50589596674468));
#81354=CARTESIAN_POINT('Ctrl Pts',(15.7761208401512,2.97546007480159,5.50089355163692));
#81355=CARTESIAN_POINT('Ctrl Pts',(15.8687439006586,2.94816659723776,5.49589113652917));
#81356=CARTESIAN_POINT('Ctrl Pts',(15.9612665265484,2.92090271500329,5.49089414572553));
#81357=CARTESIAN_POINT('Ctrl Pts',(16.0525992897885,2.88925126764076,5.48589715492189));
#81358=CARTESIAN_POINT('Ctrl Pts',(16.1423005464758,2.8533404478823,5.48090016411825));
#81359=CARTESIAN_POINT('Ctrl Pts',(16.2319435201223,2.81745296103853,5.47590642008984));
#81360=CARTESIAN_POINT('Ctrl Pts',(16.3199566896999,2.77731176433479,5.47091267606143));
#81361=CARTESIAN_POINT('Ctrl Pts',(16.4059152154471,2.73309433737192,5.46591893203303));
#81362=CARTESIAN_POINT('Ctrl Pts',(16.4918570019696,2.68888552113658,5.46092616046666));
#81363=CARTESIAN_POINT('Ctrl Pts',(16.5757445472854,2.64060224345441,5.45593338890029));
#81364=CARTESIAN_POINT('Ctrl Pts',(16.6571753181588,2.58846908710251,5.45094061733392));
#81365=CARTESIAN_POINT('Ctrl Pts',(16.7309997475721,2.54120562048028,5.44641421400843));
#81366=CARTESIAN_POINT('Ctrl Pts',(16.8028050080403,2.49077861220831,5.44188781068294));
#81367=CARTESIAN_POINT('Ctrl Pts',(16.8723108164276,2.43738680900022,5.43736140735745));
#81368=CARTESIAN_POINT('',(14.2062007174671,-2.96922295374569,6.));
#81369=CARTESIAN_POINT('Ctrl Pts',(14.2062007174671,-2.96922295374569,6.));
#81370=CARTESIAN_POINT('Ctrl Pts',(13.2234854900245,-2.70650147589439,5.94732494375275));
#81371=CARTESIAN_POINT('Ctrl Pts',(12.123801666398,-1.66916420549225,5.87785090488653));
#81372=CARTESIAN_POINT('Ctrl Pts',(11.9273055846846,-0.328588204067301,
5.80837686602031));
#81373=CARTESIAN_POINT('Ctrl Pts',(11.9296688268652,-0.00354280879104964,
5.79157788340132));
#81374=CARTESIAN_POINT('',(15.7942157255603,-2.96911158956221,5.99999996441182));
#81375=CARTESIAN_POINT('Origin',(15.,0.,6.));
#81376=CARTESIAN_POINT('',(11.9263421499922,0.00192556373082606,5.70842344717746));
#81377=CARTESIAN_POINT('Ctrl Pts',(15.7942157255603,-2.96911158956221,5.99999996441182));
#81378=CARTESIAN_POINT('Ctrl Pts',(15.7018690189097,-2.9938136610113,5.9950202108322));
#81379=CARTESIAN_POINT('Ctrl Pts',(15.6082018290729,-3.01424790828694,5.99004045725257));
#81380=CARTESIAN_POINT('Ctrl Pts',(15.513646119697,-3.03027555079075,5.98506070367295));
#81381=CARTESIAN_POINT('Ctrl Pts',(15.4192176285349,-3.04628162920221,5.9800876500098));
#81382=CARTESIAN_POINT('Ctrl Pts',(15.3239034261041,-3.05789281051075,5.97511459634665));
#81383=CARTESIAN_POINT('Ctrl Pts',(15.2281494838423,-3.06502040173022,5.9701415426835));
#81384=CARTESIAN_POINT('Ctrl Pts',(15.1293011648268,-3.07237832761852,5.9650077802152));
#81385=CARTESIAN_POINT('Ctrl Pts',(15.0299846568516,-3.07495779380533,5.9598740177469));
#81386=CARTESIAN_POINT('Ctrl Pts',(14.9307009746042,-3.07271864886442,5.95474025527859));
#81387=CARTESIAN_POINT('Ctrl Pts',(14.8346927168438,-3.07055337457379,5.94977585851992));
#81388=CARTESIAN_POINT('Ctrl Pts',(14.7387156335956,-3.06388244854816,5.94481146176125));
#81389=CARTESIAN_POINT('Ctrl Pts',(14.6432254126159,-3.05272241512341,5.93984706500257));
#81390=CARTESIAN_POINT('Ctrl Pts',(14.5477665125112,-3.04156604219928,5.93488429657033));
#81391=CARTESIAN_POINT('Ctrl Pts',(14.4527945968673,-3.0259235385553,5.92992152813808));
#81392=CARTESIAN_POINT('Ctrl Pts',(14.3587608067155,-3.00586336133162,5.92495875970583));
#81393=CARTESIAN_POINT('Ctrl Pts',(14.2647316542963,-2.98580417347293,5.91999623603659));
#81394=CARTESIAN_POINT('Ctrl Pts',(14.1716409683242,-2.96132783829202,5.91503371236735));
#81395=CARTESIAN_POINT('Ctrl Pts',(14.0799291539908,-2.93255381678222,5.91007118869811));
#81396=CARTESIAN_POINT('Ctrl Pts',(13.988196304435,-2.90377319559986,5.90510752681358));
#81397=CARTESIAN_POINT('Ctrl Pts',(13.8978433768556,-2.87069306354472,5.90014386492905));
#81398=CARTESIAN_POINT('Ctrl Pts',(13.8092940107979,-2.83348222109797,5.89518020304453));
#81399=CARTESIAN_POINT('Ctrl Pts',(13.7206496084393,-2.79623144182301,5.89021121387099));
#81400=CARTESIAN_POINT('Ctrl Pts',(13.6338130385796,-2.75484127792406,5.88524222469745));
#81401=CARTESIAN_POINT('Ctrl Pts',(13.5491860704935,-2.70952785406421,5.88027323552391));
#81402=CARTESIAN_POINT('Ctrl Pts',(13.4645045392964,-2.66418521444219,5.87530104260204));
#81403=CARTESIAN_POINT('Ctrl Pts',(13.382035824584,-2.61491450741817,5.87032884968017));
#81404=CARTESIAN_POINT('Ctrl Pts',(13.302153493731,-2.56197570073375,5.86535665675831));
#81405=CARTESIAN_POINT('Ctrl Pts',(13.2221525535056,-2.5089582904511,5.86037708111894));
#81406=CARTESIAN_POINT('Ctrl Pts',(13.1447460146018,-2.45226217550332,5.85539750547957));
#81407=CARTESIAN_POINT('Ctrl Pts',(13.0702748154839,-2.39218790278783,5.8504179298402));
#81408=CARTESIAN_POINT('Ctrl Pts',(13.0528932997578,-2.3781666176694,5.84925570104154));
#81409=CARTESIAN_POINT('Ctrl Pts',(13.0356715282748,-2.36396146459253,5.84809347224288));
#81410=CARTESIAN_POINT('Ctrl Pts',(13.0186135388797,-2.3495765451862,5.84693124344422));
#81411=CARTESIAN_POINT('Ctrl Pts',(12.9461274939369,-2.28844941640039,5.8419924803238));
#81412=CARTESIAN_POINT('Ctrl Pts',(12.8763338057764,-2.22384729599405,5.83705371720339));
#81413=CARTESIAN_POINT('Ctrl Pts',(12.8095899402503,-2.15603942917273,5.83211495408297));
#81414=CARTESIAN_POINT('Ctrl Pts',(12.7399398316576,-2.08527898923837,5.82696114129524));
#81415=CARTESIAN_POINT('Ctrl Pts',(12.6736116136119,-2.01102751315833,5.82180732850751));
#81416=CARTESIAN_POINT('Ctrl Pts',(12.6109747270326,-1.93363918431624,5.81665351571978));
#81417=CARTESIAN_POINT('Ctrl Pts',(12.5510981539129,-1.85966124282541,5.81172682371635));
#81418=CARTESIAN_POINT('Ctrl Pts',(12.4945948013533,-1.78281744761207,5.80680013171291));
#81419=CARTESIAN_POINT('Ctrl Pts',(12.4417498504224,-1.70345484888395,5.80187343970948));
#81420=CARTESIAN_POINT('Ctrl Pts',(12.3889350558613,-1.62413753902143,5.79694955916));
#81421=CARTESIAN_POINT('Ctrl Pts',(12.3397747666994,-1.54230465394821,5.79202567861052));
#81422=CARTESIAN_POINT('Ctrl Pts',(12.2945124128363,-1.45833438062172,5.78710179806104));
#81423=CARTESIAN_POINT('Ctrl Pts',(12.2492628016601,-1.37438774740224,5.78217930372907));
#81424=CARTESIAN_POINT('Ctrl Pts',(12.2079091590888,-1.28830531801229,5.77725680939711));
#81425=CARTESIAN_POINT('Ctrl Pts',(12.1706496583682,-1.20049110546804,5.77233431506514));
#81426=CARTESIAN_POINT('Ctrl Pts',(12.1333898750263,-1.11267622683443,5.76741178339501));
#81427=CARTESIAN_POINT('Ctrl Pts',(12.1002244689673,-1.02312995478895,5.76248925172488));
#81428=CARTESIAN_POINT('Ctrl Pts',(12.0713035446006,-0.932276419379552,
5.75756672005475));
#81429=CARTESIAN_POINT('Ctrl Pts',(12.0423595738702,-0.841350485052403,
5.75264026574183));
#81430=CARTESIAN_POINT('Ctrl Pts',(12.0176669722261,-0.749115638273084,
5.74771381142891));
#81431=CARTESIAN_POINT('Ctrl Pts',(11.997325838759,-0.656010770807662,5.742787357116));
#81432=CARTESIAN_POINT('Ctrl Pts',(11.9769751316778,-0.562862083263512,
5.73785858415292));
#81433=CARTESIAN_POINT('Ctrl Pts',(11.9609800447889,-0.468843004043297,
5.73292981118984));
#81434=CARTESIAN_POINT('Ctrl Pts',(11.9493891151334,-0.374400159098826,
5.72800103822676));
#81435=CARTESIAN_POINT('Ctrl Pts',(11.937782976746,-0.279833393473294,5.7230657981046));
#81436=CARTESIAN_POINT('Ctrl Pts',(11.9305925596139,-0.18484220117705,5.71813055798245));
#81437=CARTESIAN_POINT('Ctrl Pts',(11.927814348961,-0.0898753333799633,
5.71319531786029));
#81438=CARTESIAN_POINT('Ctrl Pts',(11.9269189341053,-0.059267595217704,
5.71160469429934));
#81439=CARTESIAN_POINT('Ctrl Pts',(11.9264814406799,-0.0286623583123479,
5.7100140707384));
#81440=CARTESIAN_POINT('Ctrl Pts',(11.9265006031257,0.00192546446421238,
5.70842344717746));
#81441=CARTESIAN_POINT('Ctrl Pts',(11.923315925464,0.00192745957886042,
5.70842344717746));
#81442=CARTESIAN_POINT('Ctrl Pts',(11.9223646639316,0.127164633308888,5.70191765635247));
#81443=CARTESIAN_POINT('Ctrl Pts',(11.985990549022,1.26546775157098,5.64273680928023));
#81444=CARTESIAN_POINT('Ctrl Pts',(13.405195535622,3.25791114562133,5.53088090596076));
#81445=CARTESIAN_POINT('Ctrl Pts',(15.8434703833997,3.157100543563,5.41926966138385));
#81446=CARTESIAN_POINT('Ctrl Pts',(16.7793150670081,2.51416252948969,5.3603334730542));
#81447=CARTESIAN_POINT('Ctrl Pts',(16.8743174193178,2.43995797974749,5.35407234097178));
#81448=CARTESIAN_POINT('Origin',(-15.,0.,8.20842344717746));
#81449=CARTESIAN_POINT('',(-13.1276888212995,2.43738653071546,0.437234105223613));
#81450=CARTESIAN_POINT('',(-13.1274106822325,2.43775135620018,0.35431326766678));
#81451=CARTESIAN_POINT('',(-13.1276888212995,2.43738653071547,8.20842344717746));
#81452=CARTESIAN_POINT('',(-14.2062007174672,-2.96922295374571,0.));
#81453=CARTESIAN_POINT('Ctrl Pts',(-13.1274106822327,2.43775135620036,0.354313267666796));
#81454=CARTESIAN_POINT('Ctrl Pts',(-12.9306016871905,2.28966113378113,0.341558957605688));
#81455=CARTESIAN_POINT('Ctrl Pts',(-12.0147638306694,1.41166373576771,0.276129591297334));
#81456=CARTESIAN_POINT('Ctrl Pts',(-11.5559315165978,-1.13347874614163,
0.158025168741734));
#81457=CARTESIAN_POINT('Ctrl Pts',(-13.2234854900246,-2.70650147589444,
0.052675056247244));
#81458=CARTESIAN_POINT('Ctrl Pts',(-14.2062007174672,-2.96922295374571,
-1.11022302462516E-15));
#81459=CARTESIAN_POINT('',(-15.793800408736,-2.96922265266357,2.23784480712919E-5));
#81460=CARTESIAN_POINT('Origin',(-15.,0.,0.));
#81461=CARTESIAN_POINT('Ctrl Pts',(-13.1276888212995,2.43738653071546,0.437234105223613));
#81462=CARTESIAN_POINT('Ctrl Pts',(-13.051399308353,2.37878371737117,0.432252081048935));
#81463=CARTESIAN_POINT('Ctrl Pts',(-12.9777841872235,2.31653453736228,0.427270056874259));
#81464=CARTESIAN_POINT('Ctrl Pts',(-12.9072078238328,2.2509160707084,0.422288032699581));
#81465=CARTESIAN_POINT('Ctrl Pts',(-12.8366777068085,2.1853406016745,0.417309273081256));
#81466=CARTESIAN_POINT('Ctrl Pts',(-12.7691827111166,2.11640053297353,0.41233051346293));
#81467=CARTESIAN_POINT('Ctrl Pts',(-12.7050537698248,2.04441288652875,0.407351753844606));
#81468=CARTESIAN_POINT('Ctrl Pts',(-12.6409455242956,1.97244847201648,0.402374600977066));
#81469=CARTESIAN_POINT('Ctrl Pts',(-12.580201467203,1.89743876208184,0.397397448109526));
#81470=CARTESIAN_POINT('Ctrl Pts',(-12.5231146160657,1.81973653171346,0.392420295241986));
#81471=CARTESIAN_POINT('Ctrl Pts',(-12.4660305235926,1.74203805622663,0.387443382890316));
#81472=CARTESIAN_POINT('Ctrl Pts',(-12.4126035458098,1.66164767378587,0.382466470538644));
#81473=CARTESIAN_POINT('Ctrl Pts',(-12.3630847891828,1.57894915084718,0.377489558186974));
#81474=CARTESIAN_POINT('Ctrl Pts',(-12.3135548378086,1.49623193218328,0.372511520700507));
#81475=CARTESIAN_POINT('Ctrl Pts',(-12.2679350883388,1.41120591403631,0.367533483214042));
#81476=CARTESIAN_POINT('Ctrl Pts',(-12.2264313533922,1.32428063965096,0.362555445727575));
#81477=CARTESIAN_POINT('Ctrl Pts',(-12.1848815229759,1.23725882307816,0.357571879462148));
#81478=CARTESIAN_POINT('Ctrl Pts',(-12.1474570211995,1.14833393753415,0.35258831319672));
#81479=CARTESIAN_POINT('Ctrl Pts',(-12.1143159219649,1.05793650649491,0.347604746931292));
#81480=CARTESIAN_POINT('Ctrl Pts',(-12.0811538596383,0.967481895406963,
0.342618028357679));
#81481=CARTESIAN_POINT('Ctrl Pts',(-12.0522807251901,0.875553303798613,
0.337631309784064));
#81482=CARTESIAN_POINT('Ctrl Pts',(-12.0278044011559,0.782595407737358,
0.332644591210451));
#81483=CARTESIAN_POINT('Ctrl Pts',(-12.0032892032294,0.689489873688219,
0.327649952609304));
#81484=CARTESIAN_POINT('Ctrl Pts',(-11.9831848464325,0.595352201397336,
0.322655314008159));
#81485=CARTESIAN_POINT('Ctrl Pts',(-11.967547889997,0.500636045983782,0.317660675407011));
#81486=CARTESIAN_POINT('Ctrl Pts',(-11.9606949426945,0.459126381080979,
0.315471758703847));
#81487=CARTESIAN_POINT('Ctrl Pts',(-11.9546993565402,0.417505658357757,
0.313282842000683));
#81488=CARTESIAN_POINT('Ctrl Pts',(-11.9495627393769,0.375812145894949,
0.311093925297518));
#81489=CARTESIAN_POINT('Ctrl Pts',(-11.9378061418289,0.28038477982827,0.306083971873502));
#81490=CARTESIAN_POINT('Ctrl Pts',(-11.9305115409651,0.184241362270561,
0.301074018449483));
#81491=CARTESIAN_POINT('Ctrl Pts',(-11.9277553015649,0.0878337232349656,
0.296064065025466));
#81492=CARTESIAN_POINT('Ctrl Pts',(-11.9250027908209,-0.00844349500458069,
0.291060889094605));
#81493=CARTESIAN_POINT('Ctrl Pts',(-11.9267764507165,-0.10498379110377,
0.286057713163746));
#81494=CARTESIAN_POINT('Ctrl Pts',(-11.9331010727877,-0.201328637466599,
0.281054537232885));
#81495=CARTESIAN_POINT('Ctrl Pts',(-11.9394190239762,-0.297571864291274,
0.276056638392046));
#81496=CARTESIAN_POINT('Ctrl Pts',(-11.9502783655214,-0.393619617480418,
0.271058739551204));
#81497=CARTESIAN_POINT('Ctrl Pts',(-11.9656518423827,-0.489012789571698,
0.266060840710365));
#81498=CARTESIAN_POINT('Ctrl Pts',(-11.9810141469647,-0.584336637125618,
0.261066573964123));
#81499=CARTESIAN_POINT('Ctrl Pts',(-12.0008839948583,-0.679006419251,0.256072307217882));
#81500=CARTESIAN_POINT('Ctrl Pts',(-12.0251823410208,-0.772568537946865,
0.25107804047164));
#81501=CARTESIAN_POINT('Ctrl Pts',(-12.0494716577823,-0.866095888437748,
0.246085629622767));
#81502=CARTESIAN_POINT('Ctrl Pts',(-12.0781860928816,-0.958515970974263,
0.241093218773895));
#81503=CARTESIAN_POINT('Ctrl Pts',(-12.1111957749357,-1.04938667766029,
0.236100807925022));
#81504=CARTESIAN_POINT('Ctrl Pts',(-12.1442020994384,-1.14024814151051,
0.231108904874926));
#81505=CARTESIAN_POINT('Ctrl Pts',(-12.1815026527877,-1.22956013227293,
0.226117001824831));
#81506=CARTESIAN_POINT('Ctrl Pts',(-12.2229184401607,-1.31689796871308,
0.221125098774736));
#81507=CARTESIAN_POINT('Ctrl Pts',(-12.2643411924436,-1.40425049279284,
0.216132356234265));
#81508=CARTESIAN_POINT('Ctrl Pts',(-12.3098803659345,-1.48962780842408,
0.211139613693793));
#81509=CARTESIAN_POINT('Ctrl Pts',(-12.3593102542769,-1.57262834669633,
0.206146871153322));
#81510=CARTESIAN_POINT('Ctrl Pts',(-12.4087914080391,-1.65571496765213,
0.201148950469611));
#81511=CARTESIAN_POINT('Ctrl Pts',(-12.4621711086895,-1.73641951396408,
0.196151029785898));
#81512=CARTESIAN_POINT('Ctrl Pts',(-12.5191795264361,-1.81436821729934,
0.191153109102187));
#81513=CARTESIAN_POINT('Ctrl Pts',(-12.5762206812606,-1.89236168266945,
0.186152318363039));
#81514=CARTESIAN_POINT('Ctrl Pts',(-12.6368944289551,-1.9675958133395,0.181151527623891));
#81515=CARTESIAN_POINT('Ctrl Pts',(-12.700891057101,-2.03973045245736,0.176150736884743));
#81516=CARTESIAN_POINT('Ctrl Pts',(-12.7649871612133,-2.11197721721588,
0.171142172947139));
#81517=CARTESIAN_POINT('Ctrl Pts',(-12.8324161544441,-2.18111455760436,
0.166133609009538));
#81518=CARTESIAN_POINT('Ctrl Pts',(-12.9028320208184,-2.24683971771357,
0.161125045071934));
#81519=CARTESIAN_POINT('Ctrl Pts',(-12.9405867240755,-2.28207941643806,
0.158439615566548));
#81520=CARTESIAN_POINT('Ctrl Pts',(-12.9791995150684,-2.31633888882833,
0.15575418606116));
#81521=CARTESIAN_POINT('Ctrl Pts',(-13.018613470118,-2.34957648719979,0.153068756555774));
#81522=CARTESIAN_POINT('Ctrl Pts',(-13.0916972789461,-2.41120771101968,
0.148089266008675));
#81523=CARTESIAN_POINT('Ctrl Pts',(-13.1677905197507,-2.46953626920912,
0.143109775461575));
#81524=CARTESIAN_POINT('Ctrl Pts',(-13.2465609561695,-2.52425311123324,
0.138130284914476));
#81525=CARTESIAN_POINT('Ctrl Pts',(-13.325226390291,-2.57889701480006,0.133157432110807));
#81526=CARTESIAN_POINT('Ctrl Pts',(-13.4065615679657,-2.62993851859708,
0.12818457930714));
#81527=CARTESIAN_POINT('Ctrl Pts',(-13.4902003138964,-2.67710798397105,
0.12321172650347));
#81528=CARTESIAN_POINT('Ctrl Pts',(-13.5765307278305,-2.72579546039684,
0.118078837001162));
#81529=CARTESIAN_POINT('Ctrl Pts',(-13.6653151432676,-2.77035711985146,
0.112945947498849));
#81530=CARTESIAN_POINT('Ctrl Pts',(-13.7561171347479,-2.8105440162951,0.107813057996541));
#81531=CARTESIAN_POINT('Ctrl Pts',(-13.8439376419678,-2.84941137560889,
0.102848706970231));
#81532=CARTESIAN_POINT('Ctrl Pts',(-13.9336448601417,-2.88418658323434,
0.0978843559439239));
#81533=CARTESIAN_POINT('Ctrl Pts',(-14.0248191542394,-2.91469116169477,
0.0929200049176142));
#81534=CARTESIAN_POINT('Ctrl Pts',(-14.1159645905075,-2.94518608506617,
0.0879572251718644));
#81535=CARTESIAN_POINT('Ctrl Pts',(-14.2085757605611,-2.97141292435503,
0.0829944454261152));
#81536=CARTESIAN_POINT('Ctrl Pts',(-14.3022151173914,-2.99324213982146,
0.0780316656803652));
#81537=CARTESIAN_POINT('Ctrl Pts',(-14.3958509308654,-3.01507052926033,
0.0730690737284831));
#81538=CARTESIAN_POINT('Ctrl Pts',(-14.4905144223162,-3.03250152590661,
0.0681064817766009));
#81539=CARTESIAN_POINT('Ctrl Pts',(-14.5857561229236,-3.04545633038871,
0.063143889824719));
#81540=CARTESIAN_POINT('Ctrl Pts',(-14.6810207609007,-3.05841425481867,
0.0581801027156136));
#81541=CARTESIAN_POINT('Ctrl Pts',(-14.7768634458436,-3.06689378697388,
0.0532163156065092));
#81542=CARTESIAN_POINT('Ctrl Pts',(-14.8728289534792,-3.07086791883448,
0.0482525284974038));
#81543=CARTESIAN_POINT('Ctrl Pts',(-14.9688990315199,-3.07484638117369,
0.0432833325154427));
#81544=CARTESIAN_POINT('Ctrl Pts',(-15.0650917564406,-3.07430962911643,
0.03831413653348));
#81545=CARTESIAN_POINT('Ctrl Pts',(-15.1609516192215,-3.06928278695039,
0.0333449405515189));
#81546=CARTESIAN_POINT('Ctrl Pts',(-15.2568742304286,-3.06425265428898,
0.0283724918085184));
#81547=CARTESIAN_POINT('Ctrl Pts',(-15.3524631060846,-3.05472662614582,
0.0234000430655198));
#81548=CARTESIAN_POINT('Ctrl Pts',(-15.4472696718276,-3.04078149340974,
0.0184275943225192));
#81549=CARTESIAN_POINT('Ctrl Pts',(-15.5422182387491,-3.02681547366795,
0.0134476978508148));
#81550=CARTESIAN_POINT('Ctrl Pts',(-15.6363817250837,-3.00841722912106,
0.00846780137910505));
#81551=CARTESIAN_POINT('Ctrl Pts',(-15.7293238804778,-2.98571414026272,
0.00348790490740036));
#81552=CARTESIAN_POINT('Ctrl Pts',(-15.7508834651356,-2.9804477553359,0.00233272942095613));
#81553=CARTESIAN_POINT('Ctrl Pts',(-15.7723774072569,-2.97494993866391,
0.00117755393451479));
#81554=CARTESIAN_POINT('Ctrl Pts',(-15.793800408736,-2.96922265266357,2.23784480706257E-5));
#81555=CARTESIAN_POINT('Origin',(-15.,0.,8.20842344717746));
#81556=CARTESIAN_POINT('',(-13.1276888212995,2.43738653071547,1.43740553117474));
#81557=CARTESIAN_POINT('',(-13.1276888212995,2.43738653071547,1.35414034322078));
#81558=CARTESIAN_POINT('',(-13.1276888212995,2.43738653071547,8.20842344717746));
#81559=CARTESIAN_POINT('',(-18.0729669117909,0.00038412414453365,0.708423426334819));
#81560=CARTESIAN_POINT('Ctrl Pts',(-13.1276888212995,2.43738653071547,1.35414034322078));
#81561=CARTESIAN_POINT('Ctrl Pts',(-13.0511528609175,2.37859440546573,1.34915698327503));
#81562=CARTESIAN_POINT('Ctrl Pts',(-12.9773706598892,2.31618001504235,1.34417362332928));
#81563=CARTESIAN_POINT('Ctrl Pts',(-12.9066944270949,2.25043863023291,1.33919026338353));
#81564=CARTESIAN_POINT('Ctrl Pts',(-12.8360138629279,2.18469321648145,1.33420659803398));
#81565=CARTESIAN_POINT('Ctrl Pts',(-12.7684399658257,2.11562070261525,1.32922293268444));
#81566=CARTESIAN_POINT('Ctrl Pts',(-12.7042891787565,2.04355427508681,1.3242392673349));
#81567=CARTESIAN_POINT('Ctrl Pts',(-12.6398874552402,1.97120594777026,1.31923610755148));
#81568=CARTESIAN_POINT('Ctrl Pts',(-12.5789359777004,1.89584056428445,1.31423294776806));
#81569=CARTESIAN_POINT('Ctrl Pts',(-12.5217140883649,1.81782870210342,1.30922978798464));
#81570=CARTESIAN_POINT('Ctrl Pts',(-12.464630368716,1.74000520969961,1.30423870898058));
#81571=CARTESIAN_POINT('Ctrl Pts',(-12.4112584556626,1.65954839497049,1.29924762997651));
#81572=CARTESIAN_POINT('Ctrl Pts',(-12.3618313474449,1.57685395984401,1.29425655097245));
#81573=CARTESIAN_POINT('Ctrl Pts',(-12.3122247836463,1.49385928506286,1.28924735079935));
#81574=CARTESIAN_POINT('Ctrl Pts',(-12.2665919228553,1.40861110815873,1.28423815062626));
#81575=CARTESIAN_POINT('Ctrl Pts',(-12.2251204633718,1.32153161415148,1.27922895045317));
#81576=CARTESIAN_POINT('Ctrl Pts',(-12.1836490038882,1.23445212014421,1.27421975028007));
#81577=CARTESIAN_POINT('Ctrl Pts',(-12.1463390605124,1.14554173821997,1.26921055010698));
#81578=CARTESIAN_POINT('Ctrl Pts',(-12.1133282369444,1.05523854287914,1.26420134993389));
#81579=CARTESIAN_POINT('Ctrl Pts',(-12.0803779751112,0.965101017993265,
1.25920133965123));
#81580=CARTESIAN_POINT('Ctrl Pts',(-12.0515960334417,0.873261122870222,
1.25420132936858));
#81581=CARTESIAN_POINT('Ctrl Pts',(-12.0271589963609,0.780140126568347,
1.24920131908592));
#81582=CARTESIAN_POINT('Ctrl Pts',(-12.0027549758747,0.687144944953781,
1.24420806425859));
#81583=CARTESIAN_POINT('Ctrl Pts',(-11.9826843033618,0.592872523079586,
1.23921480943126));
#81584=CARTESIAN_POINT('Ctrl Pts',(-11.9670748685875,0.497762390349688,
1.23422155460393));
#81585=CARTESIAN_POINT('Ctrl Pts',(-11.9514818203138,0.402752102506203,
1.22923354160465));
#81586=CARTESIAN_POINT('Ctrl Pts',(-11.9403407701969,0.306906282816328,
1.22424552860537));
#81587=CARTESIAN_POINT('Ctrl Pts',(-11.9337290537548,0.210676847833027,
1.21925751560608));
#81588=CARTESIAN_POINT('Ctrl Pts',(-11.927122028302,0.114515687290051,1.2142730415842));
#81589=CARTESIAN_POINT('Ctrl Pts',(-11.9250379781261,0.0179718890919223,
1.20928856756232));
#81590=CARTESIAN_POINT('Ctrl Pts',(-11.9275025484609,-0.0784962437677143,
1.20430409354044));
#81591=CARTESIAN_POINT('Ctrl Pts',(-11.9299662316253,-0.174929651031547,
1.19932141377771));
#81592=CARTESIAN_POINT('Ctrl Pts',(-11.9369752707827,-0.271287008817974,
1.19433873401497));
#81593=CARTESIAN_POINT('Ctrl Pts',(-11.9485032013853,-0.367109708458424,
1.18935605425224));
#81594=CARTESIAN_POINT('Ctrl Pts',(-11.9600301272186,-0.462924056233761,
1.18437380877773));
#81595=CARTESIAN_POINT('Ctrl Pts',(-11.9760751087741,-0.558203402842771,
1.17939156330321));
#81596=CARTESIAN_POINT('Ctrl Pts',(-11.9965598908141,-0.652495027209744,
1.1744093178287));
#81597=CARTESIAN_POINT('Ctrl Pts',(-12.0170484757832,-0.746804156491061,
1.16942614741752));
#81598=CARTESIAN_POINT('Ctrl Pts',(-12.0419784049871,-0.840124770540819,
1.16444297700634));
#81599=CARTESIAN_POINT('Ctrl Pts',(-12.0712207052525,-0.932016143990043,
1.15945980659517));
#81600=CARTESIAN_POINT('Ctrl Pts',(-12.1004944921847,-1.02400646153868,
1.15447127055183));
#81601=CARTESIAN_POINT('Ctrl Pts',(-12.1340897866456,-1.11456404737922,
1.14948273450849));
#81602=CARTESIAN_POINT('Ctrl Pts',(-12.1718283629447,-1.20326532458815,
1.14449419846516));
#81603=CARTESIAN_POINT('Ctrl Pts',(-12.2095893537256,-1.29201928510813,
1.13950269952654));
#81604=CARTESIAN_POINT('Ctrl Pts',(-12.2514983357602,-1.37891434662163,
1.13451120058792));
#81605=CARTESIAN_POINT('Ctrl Pts',(-12.2973306779117,-1.46355074576965,
1.12951970164929));
#81606=CARTESIAN_POINT('Ctrl Pts',(-12.3432365532322,-1.54832293511182,
1.124520194376));
#81607=CARTESIAN_POINT('Ctrl Pts',(-12.3930781303693,-1.63082885118772,
1.1195206871027));
#81608=CARTESIAN_POINT('Ctrl Pts',(-12.4465870068629,-1.71069703234628,
1.11452117982941));
#81609=CARTESIAN_POINT('Ctrl Pts',(-12.4763587074866,-1.75513473567015,
1.11173951361699));
#81610=CARTESIAN_POINT('Ctrl Pts',(-12.5072649463413,-1.7987564516688,1.10895784740456));
#81611=CARTESIAN_POINT('Ctrl Pts',(-12.5392542688128,-1.84150283639315,
1.10617618119214));
#81612=CARTESIAN_POINT('Ctrl Pts',(-12.5967762887544,-1.91836780897057,
1.10117429159339));
#81613=CARTESIAN_POINT('Ctrl Pts',(-12.6580034329227,-1.99266890753169,
1.09617240199463));
#81614=CARTESIAN_POINT('Ctrl Pts',(-12.7226790194845,-2.06402795564982,
1.09117051239587));
#81615=CARTESIAN_POINT('Ctrl Pts',(-12.7872672215848,-2.13529058914964,
1.08617538094887));
#81616=CARTESIAN_POINT('Ctrl Pts',(-12.8552943138539,-2.20361875046076,
1.08118024950187));
#81617=CARTESIAN_POINT('Ctrl Pts',(-12.9264617303691,-2.26866509083559,
1.07618511805487));
#81618=CARTESIAN_POINT('Ctrl Pts',(-12.9975543911876,-2.33364310521622,
1.07119523359517));
#81619=CARTESIAN_POINT('Ctrl Pts',(-13.071780496557,-2.3953458575995,1.06620534913548));
#81620=CARTESIAN_POINT('Ctrl Pts',(-13.1488034987124,-2.4534615879652,1.06121546467578));
#81621=CARTESIAN_POINT('Ctrl Pts',(-13.2257716378871,-2.51153592287618,
1.05622913447816));
#81622=CARTESIAN_POINT('Ctrl Pts',(-13.3055323642548,-2.56602805183336,
1.05124280428054));
#81623=CARTESIAN_POINT('Ctrl Pts',(-13.3877155532199,-2.61666603002201,
1.04625647408292));
#81624=CARTESIAN_POINT('Ctrl Pts',(-13.469869002451,-2.66728568378177,1.04127194829488));
#81625=CARTESIAN_POINT('Ctrl Pts',(-13.5544427995286,-2.71405372823244,
1.03628742250684));
#81626=CARTESIAN_POINT('Ctrl Pts',(-13.641038102371,-2.75674170186339,1.0313028967188));
#81627=CARTESIAN_POINT('Ctrl Pts',(-13.7276256457696,-2.7994258504031,1.02631881757332));
#81628=CARTESIAN_POINT('Ctrl Pts',(-13.8162339413956,-2.83803046134822,
1.02133473842784));
#81629=CARTESIAN_POINT('Ctrl Pts',(-13.9064407874791,-2.87237366975653,
1.01635065928236));
#81630=CARTESIAN_POINT('Ctrl Pts',(-13.9966641103045,-2.9067231511276,1.01136566976933));
#81631=CARTESIAN_POINT('Ctrl Pts',(-14.088486153683,-2.93680952812858,1.00638068025629));
#81632=CARTESIAN_POINT('Ctrl Pts',(-14.1814670537934,-2.96249996894082,
1.00139569074325));
#81633=CARTESIAN_POINT('Ctrl Pts',(-14.2745474178067,-2.98821789143486,
0.996405368667162));
#81634=CARTESIAN_POINT('Ctrl Pts',(-14.3687886900333,-3.00953037299097,
0.991415046591069));
#81635=CARTESIAN_POINT('Ctrl Pts',(-14.463738460438,-3.02635520241537,0.986424724514978));
#81636=CARTESIAN_POINT('Ctrl Pts',(-14.5587442987757,-3.04318996691812,
0.981431455648782));
#81637=CARTESIAN_POINT('Ctrl Pts',(-14.6544590336937,-3.05553174657388,
0.976438186782588));
#81638=CARTESIAN_POINT('Ctrl Pts',(-14.7504248369792,-3.06335020655542,
0.971444917916392));
#81639=CARTESIAN_POINT('Ctrl Pts',(-14.8465437369471,-3.07118113952467,
0.9664436831616));
#81640=CARTESIAN_POINT('Ctrl Pts',(-14.9429140671563,-3.07447432925586,
0.961442448406806));
#81641=CARTESIAN_POINT('Ctrl Pts',(-15.0390777808304,-3.07325156423052,
0.956441213652014));
#81642=CARTESIAN_POINT('Ctrl Pts',(-15.0922124281551,-3.0725759332061,0.953677813251482));
#81643=CARTESIAN_POINT('Ctrl Pts',(-15.1452840680108,-3.07052248433969,
0.95091441285095));
#81644=CARTESIAN_POINT('Ctrl Pts',(-15.1982164315189,-3.06710164426872,
0.948151012450418));
#81645=CARTESIAN_POINT('Ctrl Pts',(-15.2940290516472,-3.06090959788129,
0.943148994492202));
#81646=CARTESIAN_POINT('Ctrl Pts',(-15.3897176588972,-3.05021288875187,
0.938146976533989));
#81647=CARTESIAN_POINT('Ctrl Pts',(-15.4848252204982,-3.03502005851178,
0.933144958575774));
#81648=CARTESIAN_POINT('Ctrl Pts',(-15.5798046352281,-3.01984769892225,
0.928149680280945));
#81649=CARTESIAN_POINT('Ctrl Pts',(-15.6742041310068,-3.00019132713698,
0.923154401986114));
#81650=CARTESIAN_POINT('Ctrl Pts',(-15.7675696339611,-2.9761114070244,0.918159123691285));
#81651=CARTESIAN_POINT('Ctrl Pts',(-15.8608374034989,-2.95205669336165,
0.913169074368608));
#81652=CARTESIAN_POINT('Ctrl Pts',(-15.9530729096405,-2.92358774575591,
0.90817902504593));
#81653=CARTESIAN_POINT('Ctrl Pts',(-16.0438311560454,-2.89081628051124,
0.903188975723253));
#81654=CARTESIAN_POINT('Ctrl Pts',(-16.1345252279343,-2.85806798773857,
0.898202454829265));
#81655=CARTESIAN_POINT('Ctrl Pts',(-16.2237437054578,-2.82102337386311,
0.893215933935281));
#81656=CARTESIAN_POINT('Ctrl Pts',(-16.3110566129781,-2.7798440257623,0.888229413041294));
#81657=CARTESIAN_POINT('Ctrl Pts',(-16.3983382035833,-2.73867944764435,
0.883244680685288));
#81658=CARTESIAN_POINT('Ctrl Pts',(-16.4837151860966,-2.69338326887045,
0.878259948329282));
#81659=CARTESIAN_POINT('Ctrl Pts',(-16.5667783337623,-2.64416487815208,
0.873275215973276));
#81660=CARTESIAN_POINT('Ctrl Pts',(-16.6498342971844,-2.59495074439866,
0.86829091475349));
#81661=CARTESIAN_POINT('Ctrl Pts',(-16.7305764465929,-2.54181529688789,
0.863306613533704));
#81662=CARTESIAN_POINT('Ctrl Pts',(-16.8086218371115,-2.48501293765718,
0.858322312313918));
#81663=CARTESIAN_POINT('Ctrl Pts',(-16.8866817196699,-2.42820003094824,
0.853337085572564));
#81664=CARTESIAN_POINT('Ctrl Pts',(-16.9620434943531,-2.36771911822442,
0.848351858831209));
#81665=CARTESIAN_POINT('Ctrl Pts',(-17.0343556498668,-2.30386617229709,
0.843366632089855));
#81666=CARTESIAN_POINT('Ctrl Pts',(-17.106745465764,-2.23994465084152,0.83837605141295));
#81667=CARTESIAN_POINT('Ctrl Pts',(-17.1760787949031,-2.17264415716956,
0.833385470736046));
#81668=CARTESIAN_POINT('Ctrl Pts',(-17.2420396810971,-2.1022988175771,0.828394890059141));
#81669=CARTESIAN_POINT('Ctrl Pts',(-17.3080396798945,-2.03191176554673,
0.823401350134505));
#81670=CARTESIAN_POINT('Ctrl Pts',(-17.370662969492,-1.95847660590655,0.81840781020987));
#81671=CARTESIAN_POINT('Ctrl Pts',(-17.4296340943692,-1.88236033146656,
0.813414270285233));
#81672=CARTESIAN_POINT('Ctrl Pts',(-17.4886994892553,-1.80612237913951,
0.808412747791935));
#81673=CARTESIAN_POINT('Ctrl Pts',(-17.5441008104129,-1.72719511273795,
0.803411225298637));
#81674=CARTESIAN_POINT('Ctrl Pts',(-17.5956061479273,-1.64597417198513,
0.79840970280534));
#81675=CARTESIAN_POINT('Ctrl Pts',(-17.6240416865902,-1.60113297081111,
0.795648416439785));
#81676=CARTESIAN_POINT('Ctrl Pts',(-17.6512905328349,-1.55559309417903,
0.792887130074228));
#81677=CARTESIAN_POINT('Ctrl Pts',(-17.6773198464595,-1.50942395957991,
0.790125843708673));
#81678=CARTESIAN_POINT('Ctrl Pts',(-17.7264573005471,-1.42226708082616,
0.7849131598874));
#81679=CARTESIAN_POINT('Ctrl Pts',(-17.7714055398365,-1.33258368240962,
0.779700476066124));
#81680=CARTESIAN_POINT('Ctrl Pts',(-17.8119086602719,-1.24079488082752,
0.774487792244851));
#81681=CARTESIAN_POINT('Ctrl Pts',(-17.8523389474109,-1.14917113519486,
0.769284481946953));
#81682=CARTESIAN_POINT('Ctrl Pts',(-17.8883398717102,-1.05544987303415,
0.764081171649055));
#81683=CARTESIAN_POINT('Ctrl Pts',(-17.919700908017,-0.960077526934394,
0.758877861351157));
#81684=CARTESIAN_POINT('Ctrl Pts',(-17.9509937778641,-0.864912482504336,
0.753685860986975));
#81685=CARTESIAN_POINT('Ctrl Pts',(-17.9776667349434,-0.768103869508663,
0.748493860622791));
#81686=CARTESIAN_POINT('Ctrl Pts',(-17.9995573856055,-0.670117706421588,
0.743301860258608));
#81687=CARTESIAN_POINT('Ctrl Pts',(-18.0214192330996,-0.572260471064923,
0.738116691397999));
#81688=CARTESIAN_POINT('Ctrl Pts',(-18.0385112123576,-0.473229143462907,
0.73293152253739));
#81689=CARTESIAN_POINT('Ctrl Pts',(-18.0507206053183,-0.373505071299328,
0.72774635367678));
#81690=CARTESIAN_POINT('Ctrl Pts',(-18.0629117058791,-0.273930408088415,
0.722568953358229));
#81691=CARTESIAN_POINT('Ctrl Pts',(-18.0702347462959,-0.173665449625611,
0.717391553039679));
#81692=CARTESIAN_POINT('Ctrl Pts',(-18.0726281689781,-0.0732009918108132,
0.712214152721128));
#81693=CARTESIAN_POINT('Ctrl Pts',(-18.0732122948632,-0.048682175818936,
0.71095058420657));
#81694=CARTESIAN_POINT('Ctrl Pts',(-18.0735030397513,-0.0241515163599685,
0.709687015692014));
#81695=CARTESIAN_POINT('Ctrl Pts',(-18.0734999760384,0.000383786650054932,
0.708423447177457));
#81696=CARTESIAN_POINT('Ctrl Pts',(-18.0685384920293,0.000386927872650887,
0.708423253185047));
#81697=CARTESIAN_POINT('Ctrl Pts',(-18.0689057127741,0.493586641182848,
0.682982393779012));
#81698=CARTESIAN_POINT('Ctrl Pts',(-17.7245434653973,2.00734820677417,0.604866478125731));
#81699=CARTESIAN_POINT('Ctrl Pts',(-15.5876863906459,3.45239524460836,0.486829816286313));
#81700=CARTESIAN_POINT('Ctrl Pts',(-13.7434190668955,2.90127091574708,0.394234013852931));
#81701=CARTESIAN_POINT('Ctrl Pts',(-13.1274106822327,2.43775135620036,0.354313267666796));
#81702=CARTESIAN_POINT('',(-18.0734999054211,0.000762480339119835,0.791576552865793));
#81703=CARTESIAN_POINT('Ctrl Pts',(-18.0734999054209,0.000762481169335827,
0.791576552822548));
#81704=CARTESIAN_POINT('Ctrl Pts',(-18.0734897331699,0.0417660022134045,
0.789440845722604));
#81705=CARTESIAN_POINT('Ctrl Pts',(-18.0726590539714,0.0827584360577896,
0.787305138622661));
#81706=CARTESIAN_POINT('Ctrl Pts',(-18.0710089906967,0.1237175373978,0.785169431522718));
#81707=CARTESIAN_POINT('Ctrl Pts',(-18.0671444936551,0.21964496538364,0.780167542264262));
#81708=CARTESIAN_POINT('Ctrl Pts',(-18.0587743123539,0.315558236027131,
0.775165653005807));
#81709=CARTESIAN_POINT('Ctrl Pts',(-18.0458957639553,0.411000298198215,
0.770163763747351));
#81710=CARTESIAN_POINT('Ctrl Pts',(-18.0330346160107,0.50631340676763,0.765168632637455));
#81711=CARTESIAN_POINT('Ctrl Pts',(-18.0156772656074,0.601156141341239,
0.760173501527557));
#81712=CARTESIAN_POINT('Ctrl Pts',(-17.9938730087447,0.695073131051469,
0.755178370417661));
#81713=CARTESIAN_POINT('Ctrl Pts',(-17.9720916555014,0.788891468512587,
0.750188486291512));
#81714=CARTESIAN_POINT('Ctrl Pts',(-17.9458727806176,0.881785569398113,
0.745198602165363));
#81715=CARTESIAN_POINT('Ctrl Pts',(-17.915317139935,0.973307877087693,0.740208718039215));
#81716=CARTESIAN_POINT('Ctrl Pts',(-17.8847832637967,1.06476499415235,0.735222388168555));
#81717=CARTESIAN_POINT('Ctrl Pts',(-17.8499189014104,1.15485184581244,0.730236058297896));
#81718=CARTESIAN_POINT('Ctrl Pts',(-17.8108750323348,1.24313466792495,0.725249728427236));
#81719=CARTESIAN_POINT('Ctrl Pts',(-17.7718452920814,1.33138554309363,0.720265202961968));
#81720=CARTESIAN_POINT('Ctrl Pts',(-17.72863922749,1.41783328525055,0.715280677496699));
#81721=CARTESIAN_POINT('Ctrl Pts',(-17.6814561150035,1.50206369815343,0.710296152031431));
#81722=CARTESIAN_POINT('Ctrl Pts',(-17.634277230356,1.5862865635968,0.705312073204175));
#81723=CARTESIAN_POINT('Ctrl Pts',(-17.5831222208386,1.66829211237906,0.700327994376919));
#81724=CARTESIAN_POINT('Ctrl Pts',(-17.5282360078883,1.7476913166853,0.695343915549662));
#81725=CARTESIAN_POINT('Ctrl Pts',(-17.4733397696355,1.82710502374163,0.690358926349937));
#81726=CARTESIAN_POINT('Ctrl Pts',(-17.4147112237775,1.90391108018195,0.685373937150211));
#81727=CARTESIAN_POINT('Ctrl Pts',(-17.3526376214765,1.97775086196756,0.680388947950486));
#81728=CARTESIAN_POINT('Ctrl Pts',(-17.2904976174322,2.051669632084,0.675398626178445));
#81729=CARTESIAN_POINT('Ctrl Pts',(-17.2249054824184,2.12261545669681,0.670408304406402));
#81730=CARTESIAN_POINT('Ctrl Pts',(-17.1561874805781,2.19026432162835,0.665417982634361));
#81731=CARTESIAN_POINT('Ctrl Pts',(-17.0874289006215,2.25795313334886,0.660424714067412));
#81732=CARTESIAN_POINT('Ctrl Pts',(-17.0155411048374,2.32234081635242,0.655431445500464));
#81733=CARTESIAN_POINT('Ctrl Pts',(-16.9408842074238,2.38314303879831,0.650438176933514));
#81734=CARTESIAN_POINT('Ctrl Pts',(-16.8661082078042,2.44404226070539,0.645436942467604));
#81735=CARTESIAN_POINT('Ctrl Pts',(-16.7885546382178,2.50134434053398,0.640435708001695));
#81736=CARTESIAN_POINT('Ctrl Pts',(-16.7086133177834,2.55480777756239,0.635434473535785));
#81737=CARTESIAN_POINT('Ctrl Pts',(-16.6644421970374,2.58434869482076,0.632671069950852));
#81738=CARTESIAN_POINT('Ctrl Pts',(-16.6195425459766,2.61271845698118,0.629907666365919));
#81739=CARTESIAN_POINT('Ctrl Pts',(-16.5739831242587,2.6398824546841,0.627144262780987));
#81740=CARTESIAN_POINT('Ctrl Pts',(-16.4915163487453,2.68905180794064,0.622142246194769));
#81741=CARTESIAN_POINT('Ctrl Pts',(-16.4066001453163,2.73443861633628,0.617140229608553));
#81742=CARTESIAN_POINT('Ctrl Pts',(-16.3196159936231,2.77579103669102,0.612138213022337));
#81743=CARTESIAN_POINT('Ctrl Pts',(-16.2327490435889,2.81708773916869,0.607142936108014));
#81744=CARTESIAN_POINT('Ctrl Pts',(-16.1438200757757,2.85436067080395,0.602147659193694));
#81745=CARTESIAN_POINT('Ctrl Pts',(-16.0532375423307,2.88740245366405,0.597152382279371));
#81746=CARTESIAN_POINT('Ctrl Pts',(-15.9627498292833,2.92040964889597,0.592162334343801));
#81747=CARTESIAN_POINT('Ctrl Pts',(-15.8706124014376,2.94919435098315,0.58717228640823));
#81748=CARTESIAN_POINT('Ctrl Pts',(-15.7772552616524,2.97359656110805,0.582182238472661));
#81749=CARTESIAN_POINT('Ctrl Pts',(-15.6839641341344,2.99798151657821,0.577195718969713));
#81750=CARTESIAN_POINT('Ctrl Pts',(-15.5894554322189,3.01799003000409,0.572209199466765));
#81751=CARTESIAN_POINT('Ctrl Pts',(-15.4941750289515,3.03351170934955,0.567222679963817));
#81752=CARTESIAN_POINT('Ctrl Pts',(-15.3989288003828,3.04902782145664,0.562237949000759));
#81753=CARTESIAN_POINT('Ctrl Pts',(-15.3029118527341,3.06006022673292,0.557253218037698));
#81754=CARTESIAN_POINT('Ctrl Pts',(-15.2065800368109,3.06654967975267,0.55226848707464));
#81755=CARTESIAN_POINT('Ctrl Pts',(-15.1102565527621,3.07303857149049,0.54728418724798));
#81756=CARTESIAN_POINT('Ctrl Pts',(-15.0136186920404,3.07498526297084,0.542299887421322));
#81757=CARTESIAN_POINT('Ctrl Pts',(-14.9171261439273,3.07238249148436,0.537315587594661));
#81758=CARTESIAN_POINT('Ctrl Pts',(-14.8206156783357,3.06977923669525,0.532330362244866));
#81759=CARTESIAN_POINT('Ctrl Pts',(-14.7242510172003,3.06262485300488,0.52734513689507));
#81760=CARTESIAN_POINT('Ctrl Pts',(-14.6284894927425,3.05096414154563,0.522359911545275));
#81761=CARTESIAN_POINT('Ctrl Pts',(-14.532625123974,3.03929090691658,0.517369332249125));
#81762=CARTESIAN_POINT('Ctrl Pts',(-14.437365620933,3.0231017359599,0.512378752952973));
#81763=CARTESIAN_POINT('Ctrl Pts',(-14.3431606265272,3.0024930120578,0.507388173656824));
#81764=CARTESIAN_POINT('Ctrl Pts',(-14.2488997716114,2.98187206785,0.50239463510881));
#81765=CARTESIAN_POINT('Ctrl Pts',(-14.1556950936047,2.95682646614238,0.497401096560798));
#81766=CARTESIAN_POINT('Ctrl Pts',(-14.0639814756913,2.92750261693324,0.492407558012784));
#81767=CARTESIAN_POINT('Ctrl Pts',(-13.9721212458973,2.89813189110122,0.487406036876205));
#81768=CARTESIAN_POINT('Ctrl Pts',(-13.8817572460333,2.86446941494189,0.482404515739625));
#81769=CARTESIAN_POINT('Ctrl Pts',(-13.7933047000624,2.82670987246808,0.477402994603045));
#81770=CARTESIAN_POINT('Ctrl Pts',(-13.7444707503213,2.80586312827126,0.47464169441511));
#81771=CARTESIAN_POINT('Ctrl Pts',(-13.6962190030361,2.78376839987139,0.471880394227175));
#81772=CARTESIAN_POINT('Ctrl Pts',(-13.6486158438361,2.76046429291688,0.46911909403924));
#81773=CARTESIAN_POINT('Ctrl Pts',(-13.5625000336455,2.71830633355279,0.464123803666508));
#81774=CARTESIAN_POINT('Ctrl Pts',(-13.4782063288343,2.6720401092025,0.45912851329378));
#81775=CARTESIAN_POINT('Ctrl Pts',(-13.396153501264,2.62184642160679,0.454133222921047));
#81776=CARTESIAN_POINT('Ctrl Pts',(-13.3142210451482,2.57172636812416,0.449145260636641));
#81777=CARTESIAN_POINT('Ctrl Pts',(-13.2345233024221,2.51769053448111,0.444157298352234));
#81778=CARTESIAN_POINT('Ctrl Pts',(-13.157456487099,2.45996659592493,0.43916933606783));
#81779=CARTESIAN_POINT('Ctrl Pts',(-13.1474896863913,2.45250134659235,0.438524259119758));
#81780=CARTESIAN_POINT('Ctrl Pts',(-13.1375668557,2.44497447542531,0.437879182171686));
#81781=CARTESIAN_POINT('Ctrl Pts',(-13.1276888212995,2.43738653071546,0.437234105223613));
#81782=CARTESIAN_POINT('Ctrl Pts',(-13.1276888212995,2.43738653071547,1.43740553117474));
#81783=CARTESIAN_POINT('Ctrl Pts',(-13.0512577645854,2.37867498862629,1.43240468041753));
#81784=CARTESIAN_POINT('Ctrl Pts',(-12.977690155484,2.31644121794465,1.42740382966033));
#81785=CARTESIAN_POINT('Ctrl Pts',(-12.9073088484283,2.25100999423224,1.42240297890312));
#81786=CARTESIAN_POINT('Ctrl Pts',(-12.8832290610115,2.22862379506477,1.42069202143197));
#81787=CARTESIAN_POINT('Ctrl Pts',(-12.8595219093937,2.20586361481061,1.41898106396081));
#81788=CARTESIAN_POINT('Ctrl Pts',(-12.8361992417048,2.1827433491827,1.41727010648965));
#81789=CARTESIAN_POINT('Ctrl Pts',(-12.768032105381,2.11516779050628,1.41226934616771));
#81790=CARTESIAN_POINT('Ctrl Pts',(-12.7029146328237,2.04427796376991,1.40726858584576));
#81791=CARTESIAN_POINT('Ctrl Pts',(-12.641185842504,1.97038017153966,1.40226782552381));
#81792=CARTESIAN_POINT('Ctrl Pts',(-12.579540424382,1.89658218721594,1.39727381933353));
#81793=CARTESIAN_POINT('Ctrl Pts',(-12.5212748710505,1.81978464557945,1.39227981314325));
#81794=CARTESIAN_POINT('Ctrl Pts',(-12.4666918889697,1.7403310790158,1.38728580695297));
#81795=CARTESIAN_POINT('Ctrl Pts',(-12.4121661951544,1.66096090395694,1.38229704228563));
#81796=CARTESIAN_POINT('Ctrl Pts',(-12.3613156359765,1.57894060547886,1.37730827761828));
#81797=CARTESIAN_POINT('Ctrl Pts',(-12.31440242706,1.49464642180646,1.37231951295094));
#81798=CARTESIAN_POINT('Ctrl Pts',(-12.2675225226475,1.41041208004298,1.36733428989451));
#81799=CARTESIAN_POINT('Ctrl Pts',(-12.2245746244422,1.32390744446607,1.36234906683807));
#81800=CARTESIAN_POINT('Ctrl Pts',(-12.1857768784946,1.23553651195931,1.35736384378164));
#81801=CARTESIAN_POINT('Ctrl Pts',(-12.1469931113263,1.14719741938873,1.35238041689482));
#81802=CARTESIAN_POINT('Ctrl Pts',(-12.1123567015251,1.0569937672414,1.34739699000801));
#81803=CARTESIAN_POINT('Ctrl Pts',(-12.0820387614793,0.965351987873125,
1.34241356312119));
#81804=CARTESIAN_POINT('Ctrl Pts',(-12.0517234806571,0.873718246517522,
1.33743057333685));
#81805=CARTESIAN_POINT('Ctrl Pts',(-12.0257260540698,0.780647045298507,
1.33244758355251));
#81806=CARTESIAN_POINT('Ctrl Pts',(-12.0041682162928,0.686581512807936,
1.32746459376817));
#81807=CARTESIAN_POINT('Ctrl Pts',(-11.9826063930718,0.59249859021968,1.32248068276776));
#81808=CARTESIAN_POINT('Ctrl Pts',(-11.9654858866696,0.497421398884258,
1.31749677176736));
#81809=CARTESIAN_POINT('Ctrl Pts',(-11.9528774275583,0.401803781112274,
1.31251286076696));
#81810=CARTESIAN_POINT('Ctrl Pts',(-11.9402554199237,0.306083416644196,
1.30752359426408));
#81811=CARTESIAN_POINT('Ctrl Pts',(-11.9321551962721,0.209821902045561,
1.3025343277612));
#81812=CARTESIAN_POINT('Ctrl Pts',(-11.9285956178948,0.113478507149245,
1.29754506125833));
#81813=CARTESIAN_POINT('Ctrl Pts',(-11.9250339289747,0.017077988392859,
1.29255283652295));
#81814=CARTESIAN_POINT('Ctrl Pts',(-11.9260182415748,-0.0794040688892739,
1.28756061178758));
#81815=CARTESIAN_POINT('Ctrl Pts',(-11.9315152897072,-0.175510206823777,
1.2825683870522));
#81816=CARTESIAN_POINT('Ctrl Pts',(-11.9370211401419,-0.27177023740481,
1.27756816837707));
#81817=CARTESIAN_POINT('Ctrl Pts',(-11.9470541089325,-0.367652710765975,
1.27256794970194));
#81818=CARTESIAN_POINT('Ctrl Pts',(-11.961529277627,-0.462707163637923,
1.26756773102681));
#81819=CARTESIAN_POINT('Ctrl Pts',(-11.9695605154953,-0.515446094532162,
1.26479346660052));
#81820=CARTESIAN_POINT('Ctrl Pts',(-11.9789583085164,-0.567930333086632,
1.26201920217422));
#81821=CARTESIAN_POINT('Ctrl Pts',(-11.9897015145351,-0.620084896129376,
1.25924493774793));
#81822=CARTESIAN_POINT('Ctrl Pts',(-12.0090675753953,-0.714100447936634,
1.254243956325));
#81823=CARTESIAN_POINT('Ctrl Pts',(-12.0328759778584,-0.807371879480203,
1.24924297490208));
#81824=CARTESIAN_POINT('Ctrl Pts',(-12.0610553300471,-0.899447873395274,
1.24424199347916));
#81825=CARTESIAN_POINT('Ctrl Pts',(-12.0891966211125,-0.991399502643214,
1.23924776675269));
#81826=CARTESIAN_POINT('Ctrl Pts',(-12.1216970011,-1.08215848743051,1.23425354002622));
#81827=CARTESIAN_POINT('Ctrl Pts',(-12.1584340584121,-1.17128359059939,
1.22925931329976));
#81828=CARTESIAN_POINT('Ctrl Pts',(-12.1951325533239,-1.26031514033326,
1.22427032894664));
#81829=CARTESIAN_POINT('Ctrl Pts',(-12.2360587183488,-1.34771581454367,
1.21928134459352));
#81830=CARTESIAN_POINT('Ctrl Pts',(-12.2810406288576,-1.43306042722451,
1.2142923602404));
#81831=CARTESIAN_POINT('Ctrl Pts',(-12.3259905879064,-1.51834441809222,
1.20930691965259));
#81832=CARTESIAN_POINT('Ctrl Pts',(-12.3749903613579,-1.60157486384683,
1.20432147906477));
#81833=CARTESIAN_POINT('Ctrl Pts',(-12.4278207005252,-1.68234832937574,
1.19933603847696));
#81834=CARTESIAN_POINT('Ctrl Pts',(-12.480631990839,-1.76309267069424,1.19435239547229));
#81835=CARTESIAN_POINT('Ctrl Pts',(-12.5372708626804,-1.84138142530105,
1.18936875246763));
#81836=CARTESIAN_POINT('Ctrl Pts',(-12.5974735826146,-1.91683829880488,
1.18438510946296));
#81837=CARTESIAN_POINT('Ctrl Pts',(-12.657671002151,-1.9922885288972,1.17940190523067));
#81838=CARTESIAN_POINT('Ctrl Pts',(-12.7214313721858,-2.06490703085392,
1.17441870099837));
#81839=CARTESIAN_POINT('Ctrl Pts',(-12.7884500009607,-2.13434974916232,
1.16943549676608));
#81840=CARTESIAN_POINT('Ctrl Pts',(-12.8554809931549,-2.2038052780797,1.16445137324545));
#81841=CARTESIAN_POINT('Ctrl Pts',(-12.9257711332084,-2.27008354421172,
1.15946724972482));
#81842=CARTESIAN_POINT('Ctrl Pts',(-12.9989788932715,-2.33287736077724,
1.15448312620419));
#81843=CARTESIAN_POINT('Ctrl Pts',(-13.0722652542397,-2.39573859711926,
1.14949365138447));
#81844=CARTESIAN_POINT('Ctrl Pts',(-13.148475155439,-2.455107629182,1.14450417656474));
#81845=CARTESIAN_POINT('Ctrl Pts',(-13.2272341880939,-2.5107177511893,1.13951470174502));
#81846=CARTESIAN_POINT('Ctrl Pts',(-13.306039883813,-2.56636082101982,1.1345222707668));
#81847=CARTESIAN_POINT('Ctrl Pts',(-13.3873973486272,-2.61824031055167,
1.12952983978859));
#81848=CARTESIAN_POINT('Ctrl Pts',(-13.4709052146561,-2.66613416531015,
1.12453740881038));
#81849=CARTESIAN_POINT('Ctrl Pts',(-13.5545467066022,-2.71410465788225,
1.11953698914558));
#81850=CARTESIAN_POINT('Ctrl Pts',(-13.640345080331,-2.75807658150661,1.11453656948078));
#81851=CARTESIAN_POINT('Ctrl Pts',(-13.7278766093667,-2.79787496664945,
1.10953614981599));
#81852=CARTESIAN_POINT('Ctrl Pts',(-13.7764022383554,-2.81993834990194,
1.10676402287938));
#81853=CARTESIAN_POINT('Ctrl Pts',(-13.8254602007446,-2.84071992500492,
1.10399189594279));
#81854=CARTESIAN_POINT('Ctrl Pts',(-13.8749763169397,-2.86019649020019,
1.10121976900618));
#81855=CARTESIAN_POINT('Ctrl Pts',(-13.9643065805911,-2.89533346857428,
1.09621867342054));
#81856=CARTESIAN_POINT('Ctrl Pts',(-14.0554402537431,-2.92634271790657,
1.09121757783489));
#81857=CARTESIAN_POINT('Ctrl Pts',(-14.1479602771984,-2.95303751428391,
1.08621648224925));
#81858=CARTESIAN_POINT('Ctrl Pts',(-14.2403553867585,-2.97969626926316,
1.08122213878392));
#81859=CARTESIAN_POINT('Ctrl Pts',(-14.3341327086799,-3.00205202791187,
1.07622779531858));
#81860=CARTESIAN_POINT('Ctrl Pts',(-14.428855760121,-3.01996630895992,1.07123345185325));
#81861=CARTESIAN_POINT('Ctrl Pts',(-14.5234794295356,-3.0378617946089,1.06624434837931));
#81862=CARTESIAN_POINT('Ctrl Pts',(-14.6190464271741,-3.0513249854539,1.06125524490537));
#81863=CARTESIAN_POINT('Ctrl Pts',(-14.7151066707566,-3.06026764204581,
1.05626614143143));
#81864=CARTESIAN_POINT('Ctrl Pts',(-14.8110987407271,-3.06920395206626,
1.05128057870641));
#81865=CARTESIAN_POINT('Ctrl Pts',(-14.9075829252319,-3.07362606516694,
1.04629501598139));
#81866=CARTESIAN_POINT('Ctrl Pts',(-15.0041015120033,-3.0734972633141,1.04130945325637));
#81867=CARTESIAN_POINT('Ctrl Pts',(-15.1005853333848,-3.07336850785489,
1.0363256862998));
#81868=CARTESIAN_POINT('Ctrl Pts',(-15.1971030942253,-3.06869209506222,
1.03134191934323));
#81869=CARTESIAN_POINT('Ctrl Pts',(-15.2931955178381,-3.05948339402581,
1.02635815238666));
#81870=CARTESIAN_POINT('Ctrl Pts',(-15.3892795132487,-3.05027550067839,
1.02137482255295));
#81871=CARTESIAN_POINT('Ctrl Pts',(-15.4849378090008,-3.03653615152407,
1.01639149271924));
#81872=CARTESIAN_POINT('Ctrl Pts',(-15.579715760275,-3.01833263363878,1.01140816288553));
#81873=CARTESIAN_POINT('Ctrl Pts',(-15.6745112237502,-3.00012575227431,
1.00642391227782));
#81874=CARTESIAN_POINT('Ctrl Pts',(-15.7684255889595,-2.97745314676545,
1.0014396616701));
#81875=CARTESIAN_POINT('Ctrl Pts',(-15.8610149724201,-2.95043309825327,
0.99645541106239));
#81876=CARTESIAN_POINT('Ctrl Pts',(-15.953703790842,-2.92338403197063,0.991465807694484));
#81877=CARTESIAN_POINT('Ctrl Pts',(-16.0450643650687,-2.89197832502405,
0.986476204326578));
#81878=CARTESIAN_POINT('Ctrl Pts',(-16.1346687587719,-2.85638391289878,
0.981486600958672));
#81879=CARTESIAN_POINT('Ctrl Pts',(-16.2243262579988,-2.82076840515736,
0.976494040419932));
#81880=CARTESIAN_POINT('Ctrl Pts',(-16.312225104865,-2.78095942996662,0.971501479881193));
#81881=CARTESIAN_POINT('Ctrl Pts',(-16.3979600378624,-2.73717189495649,
0.966508919342453));
#81882=CARTESIAN_POINT('Ctrl Pts',(-16.4838321619879,-2.6933142921092,0.961508369819661));
#81883=CARTESIAN_POINT('Ctrl Pts',(-16.5675330778827,-2.64546563514151,
0.956507820296869));
#81884=CARTESIAN_POINT('Ctrl Pts',(-16.6486847501473,-2.5938852797747,0.951507270774077));
#81885=CARTESIAN_POINT('Ctrl Pts',(-16.6936522821998,-2.5653037210894,0.948736380604204));
#81886=CARTESIAN_POINT('Ctrl Pts',(-16.7378376294089,-2.53557710926649,
0.945965490434332));
#81887=CARTESIAN_POINT('Ctrl Pts',(-16.7811809181293,-2.50475483568596,
0.943194600264459));
#81888=CARTESIAN_POINT('Ctrl Pts',(-16.8588974660735,-2.44948905468059,
0.938226264333042));
#81889=CARTESIAN_POINT('Ctrl Pts',(-16.9341838418177,-2.39049999289044,
0.933257928401624));
#81890=CARTESIAN_POINT('Ctrl Pts',(-17.0066586192695,-2.32802994733994,
0.928289592470207));
#81891=CARTESIAN_POINT('Ctrl Pts',(-17.0790351989641,-2.26564454390325,
0.923327988252394));
#81892=CARTESIAN_POINT('Ctrl Pts',(-17.1486074151297,-2.19978781560031,
0.918366384034581));
#81893=CARTESIAN_POINT('Ctrl Pts',(-17.2150233744915,-2.13074486986504,
0.913404779816767));
#81894=CARTESIAN_POINT('Ctrl Pts',(-17.2829729916507,-2.06010760473582,
0.90832860369381));
#81895=CARTESIAN_POINT('Ctrl Pts',(-17.3476183845453,-1.98613540779927,
0.903252427570853));
#81896=CARTESIAN_POINT('Ctrl Pts',(-17.4086190435062,-1.90917693084204,
0.898176251447896));
#81897=CARTESIAN_POINT('Ctrl Pts',(-17.4681388199416,-1.83408673638613,
0.893223307116927));
#81898=CARTESIAN_POINT('Ctrl Pts',(-17.5241885178778,-1.75615397477629,
0.888270362785958));
#81899=CARTESIAN_POINT('Ctrl Pts',(-17.5764905960058,-1.67573818321774,
0.883317418454989));
#81900=CARTESIAN_POINT('Ctrl Pts',(-17.6287754491663,-1.59534887549015,
0.87836610530787));
#81901=CARTESIAN_POINT('Ctrl Pts',(-17.6773148918573,-1.51247853509114,
0.873414792160749));
#81902=CARTESIAN_POINT('Ctrl Pts',(-17.7218742095594,-1.42751638776421,
0.868463479013631));
#81903=CARTESIAN_POINT('Ctrl Pts',(-17.7664314111598,-1.34255827525095,
0.863512401002118));
#81904=CARTESIAN_POINT('Ctrl Pts',(-17.8070086575104,-1.25550894786147,
0.858561322990605));
#81905=CARTESIAN_POINT('Ctrl Pts',(-17.8434173326361,-1.16678195155079,
0.853610244979092));
#81906=CARTESIAN_POINT('Ctrl Pts',(-17.8814320258966,-1.07414113072894,
0.848440770636316));
#81907=CARTESIAN_POINT('Ctrl Pts',(-17.914901702574,-0.979671707568172,
0.843271296293546));
#81908=CARTESIAN_POINT('Ctrl Pts',(-17.9436684417483,-0.88386557521798,
0.838101821950771));
#81909=CARTESIAN_POINT('Ctrl Pts',(-17.9712565102632,-0.791984944347023,
0.833144158466879));
#81910=CARTESIAN_POINT('Ctrl Pts',(-17.9945194094835,-0.698875450581568,
0.828186494982984));
#81911=CARTESIAN_POINT('Ctrl Pts',(-18.0133698527397,-0.604982958933142,
0.823228831499092));
#81912=CARTESIAN_POINT('Ctrl Pts',(-18.0322328518359,-0.511027927688841,
0.818267865831338));
#81913=CARTESIAN_POINT('Ctrl Pts',(-18.0466774803284,-0.416289299842081,
0.813306900163584));
#81914=CARTESIAN_POINT('Ctrl Pts',(-18.0566682323481,-0.321218877642427,
0.808345934495829));
#81915=CARTESIAN_POINT('Ctrl Pts',(-18.066673516729,-0.226010167783542,
0.803377752700137));
#81916=CARTESIAN_POINT('Ctrl Pts',(-18.0722119787107,-0.130469143381661,
0.798409570904445));
#81917=CARTESIAN_POINT('Ctrl Pts',(-18.0733001629596,-0.035047943623454,
0.793441389108753));
#81918=CARTESIAN_POINT('Ctrl Pts',(-18.0734363150779,-0.0231089741993823,
0.792819777027766));
#81919=CARTESIAN_POINT('Ctrl Pts',(-18.0735028661208,-0.0111718734142489,
0.79219816494678));
#81920=CARTESIAN_POINT('Ctrl Pts',(-18.0734999054211,0.000762480339109222,
0.791576552865792));
#81921=CARTESIAN_POINT('Origin',(-15.,0.,8.20842344717746));
#81922=CARTESIAN_POINT('',(-13.1276888212995,2.43738653071547,2.43734746082558));
#81923=CARTESIAN_POINT('',(-13.1254325828889,2.44028101900739,2.35408149450477));
#81924=CARTESIAN_POINT('',(-13.1276888212995,2.43738653071547,8.20842344717746));
#81925=CARTESIAN_POINT('',(-18.073498904786,-0.00259466362292773,1.70842344717746));
#81926=CARTESIAN_POINT('Ctrl Pts',(-13.1254325828889,2.44028101900739,2.35408149450477));
#81927=CARTESIAN_POINT('Ctrl Pts',(-12.4084487444517,1.88105036108211,2.30683845046461));
#81928=CARTESIAN_POINT('Ctrl Pts',(-11.4280462758325,-0.0162669500815165,
2.20692035017721));
#81929=CARTESIAN_POINT('Ctrl Pts',(-12.9443038197492,-2.98822585588414,
2.05432719364256));
#81930=CARTESIAN_POINT('Ctrl Pts',(-16.3800295351377,-3.35423238380087,
1.89630202490083));
#81931=CARTESIAN_POINT('Ctrl Pts',(-17.9731131493935,-1.40035444911347,
1.78100077607913));
#81932=CARTESIAN_POINT('Ctrl Pts',(-18.076577770913,-0.194497574487465,
1.71837458350467));
#81933=CARTESIAN_POINT('Ctrl Pts',(-18.0748543381996,-0.00259580788680448,
1.70842344717746));
#81934=CARTESIAN_POINT('Ctrl Pts',(-18.073498904786,-0.00259466362292773,
1.70842344717746));
#81935=CARTESIAN_POINT('Ctrl Pts',(-18.0735789633664,0.0922384226565076,
1.70350363328471));
#81936=CARTESIAN_POINT('Ctrl Pts',(-18.0692656912357,0.187216825807511,
1.69858381939197));
#81937=CARTESIAN_POINT('Ctrl Pts',(-18.0605453982257,0.281893801634021,
1.69366400549922));
#81938=CARTESIAN_POINT('Ctrl Pts',(-18.0518336958937,0.376477507725467,
1.68874903829421));
#81939=CARTESIAN_POINT('Ctrl Pts',(-18.0387236414728,0.47075992793125,1.68383407108921));
#81940=CARTESIAN_POINT('Ctrl Pts',(-18.0212535976478,0.564295090090703,
1.6789191038842));
#81941=CARTESIAN_POINT('Ctrl Pts',(-18.0037927532641,0.657780998152678,
1.67400672482112));
#81942=CARTESIAN_POINT('Ctrl Pts',(-17.9819765600055,0.750519985203623,
1.66909434575803));
#81943=CARTESIAN_POINT('Ctrl Pts',(-17.9558950091817,0.842073004373502,
1.66418196669494));
#81944=CARTESIAN_POINT('Ctrl Pts',(-17.9298195878756,0.933604507343941,
1.65927074210746));
#81945=CARTESIAN_POINT('Ctrl Pts',(-17.899480924029,1.02395016074908,1.65435951751998));
#81946=CARTESIAN_POINT('Ctrl Pts',(-17.8650194238835,1.11268411994169,1.64944829293251));
#81947=CARTESIAN_POINT('Ctrl Pts',(-17.8305559748702,1.20142309721957,1.64453679060532));
#81948=CARTESIAN_POINT('Ctrl Pts',(-17.7919693921325,1.28854977782556,1.63962528827814));
#81949=CARTESIAN_POINT('Ctrl Pts',(-17.7494485017389,1.37365759426636,1.63471378595096));
#81950=CARTESIAN_POINT('Ctrl Pts',(-17.7068863483411,1.45884800079765,1.62979751741735));
#81951=CARTESIAN_POINT('Ctrl Pts',(-17.6603824677528,1.54201522605512,1.62488124888374));
#81952=CARTESIAN_POINT('Ctrl Pts',(-17.6101718132093,1.62277705046865,1.61996498035013));
#81953=CARTESIAN_POINT('Ctrl Pts',(-17.5599354305212,1.70358025757101,1.61504619270044));
#81954=CARTESIAN_POINT('Ctrl Pts',(-17.5059887511946,1.78197523848825,1.61012740505074));
#81955=CARTESIAN_POINT('Ctrl Pts',(-17.4486089501875,1.85761041638489,1.60520861740105));
#81956=CARTESIAN_POINT('Ctrl Pts',(-17.391136305883,1.93336797566299,1.60028187091468));
#81957=CARTESIAN_POINT('Ctrl Pts',(-17.3302197396758,2.00635646943507,1.59535512442832));
#81958=CARTESIAN_POINT('Ctrl Pts',(-17.2661752905315,2.07625908850132,1.59042837794195));
#81959=CARTESIAN_POINT('Ctrl Pts',(-17.2220785395579,2.12438938592067,1.58703614776709));
#81960=CARTESIAN_POINT('Ctrl Pts',(-17.1764997129828,2.1710575011714,1.58364391759222));
#81961=CARTESIAN_POINT('Ctrl Pts',(-17.129551019269,2.21617118163968,1.58025168741735));
#81962=CARTESIAN_POINT('Ctrl Pts',(-17.0603370994175,2.28267984071285,1.57525070594442));
#81963=CARTESIAN_POINT('Ctrl Pts',(-16.9878837377594,2.34605894210612,1.57024972447148));
#81964=CARTESIAN_POINT('Ctrl Pts',(-16.9125054133723,2.40597699361855,1.56524874299855));
#81965=CARTESIAN_POINT('Ctrl Pts',(-16.8372289005508,2.46581411535857,1.56025451622278));
#81966=CARTESIAN_POINT('Ctrl Pts',(-16.7590356173462,2.52219920752529,1.555260289447));
#81967=CARTESIAN_POINT('Ctrl Pts',(-16.6782763784391,2.57483798472318,1.55026606267123));
#81968=CARTESIAN_POINT('Ctrl Pts',(-16.5976019114416,2.62742150768985,1.54527707826953));
#81969=CARTESIAN_POINT('Ctrl Pts',(-16.5143672088258,2.67626629507595,1.54028809386783));
#81970=CARTESIAN_POINT('Ctrl Pts',(-16.4289547970201,2.7211193355076,1.53529910946614));
#81971=CARTESIAN_POINT('Ctrl Pts',(-16.3436030552084,2.76594051600651,1.53031366883106));
#81972=CARTESIAN_POINT('Ctrl Pts',(-16.2560770666207,2.80677538294738,1.52532822819598));
#81973=CARTESIAN_POINT('Ctrl Pts',(-16.1667860369241,2.84341565622033,1.5203427875609));
#81974=CARTESIAN_POINT('Ctrl Pts',(-16.0775272026012,2.88004271823016,1.5153591445098));
#81975=CARTESIAN_POINT('Ctrl Pts',(-15.9865049971013,2.91247802533915,1.51037550145869));
#81976=CARTESIAN_POINT('Ctrl Pts',(-15.8941499124283,2.94056086216633,1.50539185840759));
#81977=CARTESIAN_POINT('Ctrl Pts',(-15.8018029589437,2.96864122650556,1.50040865412972));
#81978=CARTESIAN_POINT('Ctrl Pts',(-15.7081237793487,2.99236975505983,1.49542544985186));
#81979=CARTESIAN_POINT('Ctrl Pts',(-15.6135583580429,3.0116355010651,1.490442245574));
#81980=CARTESIAN_POINT('Ctrl Pts',(-15.5189754915764,3.03090480116058,1.48545812200874));
#81981=CARTESIAN_POINT('Ctrl Pts',(-15.4235064885192,3.04570959611494,1.48047399844347));
#81982=CARTESIAN_POINT('Ctrl Pts',(-15.3276068059865,3.05599018824854,1.47548987487821));
#81983=CARTESIAN_POINT('Ctrl Pts',(-15.2316041589666,3.0662818183321,1.4705004000155));
#81984=CARTESIAN_POINT('Ctrl Pts',(-15.1351703461965,3.07203950146474,1.46551092515279));
#81985=CARTESIAN_POINT('Ctrl Pts',(-15.0387649919052,3.07325552556285,1.46052145029008));
#81986=CARTESIAN_POINT('Ctrl Pts',(-14.9423025194942,3.07447227012934,1.45552901926975));
#81987=CARTESIAN_POINT('Ctrl Pts',(-14.8458689772977,3.07114201283781,1.45053658824942));
#81988=CARTESIAN_POINT('Ctrl Pts',(-14.749920914246,3.06330910958533,1.44554415722909));
#81989=CARTESIAN_POINT('Ctrl Pts',(-14.6538193190112,3.05546367244005,1.44054373752395));
#81990=CARTESIAN_POINT('Ctrl Pts',(-14.5582051887255,3.04310125939591,1.43554331781881));
#81991=CARTESIAN_POINT('Ctrl Pts',(-14.4635268272169,3.02631769397796,1.43054289811367));
#81992=CARTESIAN_POINT('Ctrl Pts',(-14.4110391544942,3.01701324178062,1.42777077163432));
#81993=CARTESIAN_POINT('Ctrl Pts',(-14.3588388540241,3.00635091370299,1.42499864515497));
#81994=CARTESIAN_POINT('Ctrl Pts',(-14.3070001997571,2.9943536075192,1.42222651867561));
#81995=CARTESIAN_POINT('Ctrl Pts',(-14.2134709796855,2.97270762333628,1.41722494540526));
#81996=CARTESIAN_POINT('Ctrl Pts',(-14.1207938463946,2.94663759779816,1.41222337213489));
#81997=CARTESIAN_POINT('Ctrl Pts',(-14.0294183957941,2.91622591710196,1.40722179886454));
#81998=CARTESIAN_POINT('Ctrl Pts',(-13.9381896884165,2.88586307565098,1.40222825780607));
#81999=CARTESIAN_POINT('Ctrl Pts',(-13.8482589179546,2.85117258671998,1.39723471674761));
#82000=CARTESIAN_POINT('Ctrl Pts',(-13.7600640209766,2.81228750627017,1.39224117568915));
#82001=CARTESIAN_POINT('Ctrl Pts',(-13.6719511175242,2.77343857671967,1.38725227705389));
#82002=CARTESIAN_POINT('Ctrl Pts',(-13.5855712807978,2.7304029780461,1.38226337841863));
#82003=CARTESIAN_POINT('Ctrl Pts',(-13.5013453567284,2.68336291064037,1.37727447978338));
#82004=CARTESIAN_POINT('Ctrl Pts',(-13.4171795407834,2.63635641354282,1.37228914149303));
#82005=CARTESIAN_POINT('Ctrl Pts',(-13.3351649633428,2.58535134241823,1.36730380320269));
#82006=CARTESIAN_POINT('Ctrl Pts',(-13.2556995740404,2.53057666827089,1.36231846491235));
#82007=CARTESIAN_POINT('Ctrl Pts',(-13.2122469812482,2.50062524373329,1.35959242434849));
#82008=CARTESIAN_POINT('Ctrl Pts',(-13.169556182852,2.46954750644487,1.35686638378463));
#82009=CARTESIAN_POINT('Ctrl Pts',(-13.1276888212995,2.43738653071547,1.35414034322078));
#82010=CARTESIAN_POINT('',(-18.0734993815183,0.00194982225149054,1.79157655278713));
#82011=CARTESIAN_POINT('Ctrl Pts',(-18.0734993815183,0.00194982225148788,
1.79157655278713));
#82012=CARTESIAN_POINT('Ctrl Pts',(-18.0734301645551,0.111056328367583,
1.78594824754486));
#82013=CARTESIAN_POINT('Ctrl Pts',(-18.0675471115686,0.21994398135138,1.78031994230258));
#82014=CARTESIAN_POINT('Ctrl Pts',(-18.0559442096784,0.328035420851308,
1.77469163706031));
#82015=CARTESIAN_POINT('Ctrl Pts',(-18.0442899661858,0.436605153433593,
1.76903842716809));
#82016=CARTESIAN_POINT('Ctrl Pts',(-18.0268652646068,0.544371409516094,
1.76338521727588));
#82017=CARTESIAN_POINT('Ctrl Pts',(-18.0038150252988,0.650766888977212,
1.75773200738366));
#82018=CARTESIAN_POINT('Ctrl Pts',(-17.9806384718765,0.757745410140075,
1.75204781819484));
#82019=CARTESIAN_POINT('Ctrl Pts',(-17.9517746673911,0.863337893675431,
1.74636362900601));
#82020=CARTESIAN_POINT('Ctrl Pts',(-17.9174192949469,0.966988576701586,
1.74067943981719));
#82021=CARTESIAN_POINT('Ctrl Pts',(-17.9025933139296,1.01171878771819,1.73822644120251));
#82022=CARTESIAN_POINT('Ctrl Pts',(-17.886745218295,1.05608765124302,1.73577344258782));
#82023=CARTESIAN_POINT('Ctrl Pts',(-17.8698934155499,1.10005183213486,1.73332044397313));
#82024=CARTESIAN_POINT('Ctrl Pts',(-17.8355379352173,1.18968085134503,1.72831955789956));
#82025=CARTESIAN_POINT('Ctrl Pts',(-17.7969197229677,1.27785526329013,1.72331867182598));
#82026=CARTESIAN_POINT('Ctrl Pts',(-17.7541824063681,1.36414131322687,1.71831778575241));
#82027=CARTESIAN_POINT('Ctrl Pts',(-17.711502810146,1.45031082652141,1.7133236538004));
#82028=CARTESIAN_POINT('Ctrl Pts',(-17.6647153593443,1.53459665687628,1.7083295218484));
#82029=CARTESIAN_POINT('Ctrl Pts',(-17.6140123914159,1.61658326959187,1.70333538989639));
#82030=CARTESIAN_POINT('Ctrl Pts',(-17.5633626396951,1.69848383179036,1.69834649962498));
#82031=CARTESIAN_POINT('Ctrl Pts',(-17.5088057701728,1.77808960258467,1.69335760935357));
#82032=CARTESIAN_POINT('Ctrl Pts',(-17.4505803751013,1.85500891511829,1.68836871908216));
#82033=CARTESIAN_POINT('Ctrl Pts',(-17.3923963229419,1.93187361113333,1.68338337116974));
#82034=CARTESIAN_POINT('Ctrl Pts',(-17.330549187613,2.00605529222922,1.67839802325732));
#82035=CARTESIAN_POINT('Ctrl Pts',(-17.2653207318563,2.077191428786,1.6734126753449));
#82036=CARTESIAN_POINT('Ctrl Pts',(-17.2001157839113,2.1483019284503,1.66842912411184));
#82037=CARTESIAN_POINT('Ctrl Pts',(-17.1315322330067,2.21636874143207,1.66344557287878));
#82038=CARTESIAN_POINT('Ctrl Pts',(-17.0598913363535,2.28106333371431,1.65846202164572));
#82039=CARTESIAN_POINT('Ctrl Pts',(-16.9882567327318,2.34575224313761,1.65347890817443));
#82040=CARTESIAN_POINT('Ctrl Pts',(-16.9135656430403,2.40706922698091,1.64849579470313));
#82041=CARTESIAN_POINT('Ctrl Pts',(-16.8361745122614,2.46472420577267,1.64351268123183));
#82042=CARTESIAN_POINT('Ctrl Pts',(-16.7587690869431,2.52238983373514,1.63852864735388));
#82043=CARTESIAN_POINT('Ctrl Pts',(-16.6786629818744,2.57639185127706,1.63354461347593));
#82044=CARTESIAN_POINT('Ctrl Pts',(-16.5962430110992,2.62648253364017,1.62856057959798));
#82045=CARTESIAN_POINT('Ctrl Pts',(-16.5137345100379,2.67662702022576,1.6235711921881));
#82046=CARTESIAN_POINT('Ctrl Pts',(-16.4289075569818,2.72285155613003,1.61858180477821));
#82047=CARTESIAN_POINT('Ctrl Pts',(-16.3421748464228,2.7649536943012,1.61359241736833));
#82048=CARTESIAN_POINT('Ctrl Pts',(-16.2553907279245,2.80708078711923,1.60860007266444));
#82049=CARTESIAN_POINT('Ctrl Pts',(-16.1666990057432,2.84508044425425,1.60360772796055));
#82050=CARTESIAN_POINT('Ctrl Pts',(-16.0765317345408,2.87879865126525,1.59861538325666));
#82051=CARTESIAN_POINT('Ctrl Pts',(-15.98622013161,2.91257083137568,1.59361504725249));
#82052=CARTESIAN_POINT('Ctrl Pts',(-15.8944286809185,2.94204774322958,1.58861471124831));
#82053=CARTESIAN_POINT('Ctrl Pts',(-15.8016038631026,2.9671254602155,1.58361437524414));
#82054=CARTESIAN_POINT('Ctrl Pts',(-15.7501260595822,2.9810327946775,1.58084134190656));
#82055=CARTESIAN_POINT('Ctrl Pts',(-15.6983306289836,2.99358808105795,1.57806830856899));
#82056=CARTESIAN_POINT('Ctrl Pts',(-15.646294608805,3.00478044599428,1.57529527523141));
#82057=CARTESIAN_POINT('Ctrl Pts',(-15.5524441428783,3.02496662972798,1.57029392290144));
#82058=CARTESIAN_POINT('Ctrl Pts',(-15.457483318007,3.04078686615163,1.56529257057148));
#82059=CARTESIAN_POINT('Ctrl Pts',(-15.3618540344134,3.05212449087169,1.56029121824152));
#82060=CARTESIAN_POINT('Ctrl Pts',(-15.2639515952095,3.0637316165675,1.55517098128041));
#82061=CARTESIAN_POINT('Ctrl Pts',(-15.1653489425364,3.07064013593149,1.55005074431929));
#82062=CARTESIAN_POINT('Ctrl Pts',(-15.0665345243961,3.07277975244946,1.54493050735818));
#82063=CARTESIAN_POINT('Ctrl Pts',(-14.970264993654,3.07486426483166,1.53994213806135));
#82064=CARTESIAN_POINT('Ctrl Pts',(-14.873794943287,3.072422506583,1.53495376876452));
#82065=CARTESIAN_POINT('Ctrl Pts',(-14.7775827112181,3.06544169731719,1.5299653994677));
#82066=CARTESIAN_POINT('Ctrl Pts',(-14.6814337557568,3.05846547917165,1.52498031090847));
#82067=CARTESIAN_POINT('Ctrl Pts',(-14.5855427178046,3.04695617374525,1.51999522234924));
#82068=CARTESIAN_POINT('Ctrl Pts',(-14.4903670173818,3.03095306348146,1.51501013379001));
#82069=CARTESIAN_POINT('Ctrl Pts',(-14.3952279716976,3.01495611644863,1.51002696512332));
#82070=CARTESIAN_POINT('Ctrl Pts',(-14.3008041478561,2.994468878059,1.50504379645664));
#82071=CARTESIAN_POINT('Ctrl Pts',(-14.2075458682047,2.96958224317842,1.50006062778995));
#82072=CARTESIAN_POINT('Ctrl Pts',(-14.1098318279932,2.9435065569172,1.49483936973869));
#82073=CARTESIAN_POINT('Ctrl Pts',(-14.0133979870556,2.91260071370465,1.48961811168742));
#82074=CARTESIAN_POINT('Ctrl Pts',(-13.9187468951899,2.87702867092744,1.48439685363615));
#82075=CARTESIAN_POINT('Ctrl Pts',(-13.8283716120819,2.843063574769,1.47941146292103));
#82076=CARTESIAN_POINT('Ctrl Pts',(-13.7396219250735,2.80484491284714,1.47442607220591));
#82077=CARTESIAN_POINT('Ctrl Pts',(-13.6529153365808,2.76256496024635,1.46944068149079));
#82078=CARTESIAN_POINT('Ctrl Pts',(-13.5661780948845,2.72027006049997,1.46445352830064));
#82079=CARTESIAN_POINT('Ctrl Pts',(-13.4814857768715,2.67391121750432,1.45946637511049));
#82080=CARTESIAN_POINT('Ctrl Pts',(-13.399230810013,2.62372640539905,1.45447922192034));
#82081=CARTESIAN_POINT('Ctrl Pts',(-13.3168923970172,2.57349068173336,1.44948700935584));
#82082=CARTESIAN_POINT('Ctrl Pts',(-13.2369966334426,2.51942148722912,1.44449479679134));
#82083=CARTESIAN_POINT('Ctrl Pts',(-13.1599060793514,2.46179946648623,1.43950258422684));
#82084=CARTESIAN_POINT('Ctrl Pts',(-13.1491117351832,2.45373113787068,1.4388035665428));
#82085=CARTESIAN_POINT('Ctrl Pts',(-13.1383723355347,2.44559321557167,1.43810454885877));
#82086=CARTESIAN_POINT('Ctrl Pts',(-13.1276888212995,2.43738653071547,1.43740553117474));
#82087=CARTESIAN_POINT('Ctrl Pts',(-13.1276888212995,2.43738653071547,2.43734746082558));
#82088=CARTESIAN_POINT('Ctrl Pts',(-13.0511401214871,2.37858461950126,2.43236378975877));
#82089=CARTESIAN_POINT('Ctrl Pts',(-12.9773761852912,2.3161823609361,2.42738011869197));
#82090=CARTESIAN_POINT('Ctrl Pts',(-12.9067421325381,2.25048300378137,2.42239644762517));
#82091=CARTESIAN_POINT('Ctrl Pts',(-12.8360348813808,2.18471556207091,2.41740761195638));
#82092=CARTESIAN_POINT('Ctrl Pts',(-12.7684643130332,2.11564449755975,2.41241877628759));
#82093=CARTESIAN_POINT('Ctrl Pts',(-12.7043392668803,2.0436105422542,2.4074299406188));
#82094=CARTESIAN_POINT('Ctrl Pts',(-12.6401800993334,1.97153825716767,2.402438450355));
#82095=CARTESIAN_POINT('Ctrl Pts',(-12.5794703816786,1.89650028227443,2.39744696009119));
#82096=CARTESIAN_POINT('Ctrl Pts',(-12.5224777998822,1.81886942849767,2.39245546982739));
#82097=CARTESIAN_POINT('Ctrl Pts',(-12.4653897842713,1.74110858221558,2.38745562133625));
#82098=CARTESIAN_POINT('Ctrl Pts',(-12.4120315817031,1.66074654935091,2.3824557728451));
#82099=CARTESIAN_POINT('Ctrl Pts',(-12.3626268417748,1.5781841065837,2.37745592435396));
#82100=CARTESIAN_POINT('Ctrl Pts',(-12.3229872118532,1.51194057040738,2.37344432254933));
#82101=CARTESIAN_POINT('Ctrl Pts',(-12.2858918067237,1.44428108992528,2.36943272074471));
#82102=CARTESIAN_POINT('Ctrl Pts',(-12.2514338178258,1.37542218689698,2.36542111894008));
#82103=CARTESIAN_POINT('Ctrl Pts',(-12.2084783871509,1.2895824751208,2.36042024428879));
#82104=CARTESIAN_POINT('Ctrl Pts',(-12.1694731270101,1.20157879356472,2.3554193696375));
#82105=CARTESIAN_POINT('Ctrl Pts',(-12.1346411926523,1.11180985566544,2.3504184949862));
#82106=CARTESIAN_POINT('Ctrl Pts',(-12.0998563011424,1.02216215669733,2.34542437434929));
#82107=CARTESIAN_POINT('Ctrl Pts',(-12.0692336906521,0.930754345222873,
2.34043025371238));
#82108=CARTESIAN_POINT('Ctrl Pts',(-12.0429501984913,0.83800878360397,2.33543613307547));
#82109=CARTESIAN_POINT('Ctrl Pts',(-12.0166942920677,0.74536056272929,2.33044725399849));
#82110=CARTESIAN_POINT('Ctrl Pts',(-11.9947685694811,0.651377802730684,
2.32545837492152));
#82111=CARTESIAN_POINT('Ctrl Pts',(-11.977301039206,0.556500891656688,2.32046949584454));
#82112=CARTESIAN_POINT('Ctrl Pts',(-11.9598459109866,0.461691343782987,
2.31548415890291));
#82113=CARTESIAN_POINT('Ctrl Pts',(-11.94684276163,0.365989337112503,2.31049882196128));
#82114=CARTESIAN_POINT('Ctrl Pts',(-11.9383689637715,0.269847453207505,
2.30551348501965));
#82115=CARTESIAN_POINT('Ctrl Pts',(-11.9298982195667,0.173740215398392,
2.30052994461512));
#82116=CARTESIAN_POINT('Ctrl Pts',(-11.9259536222082,0.0771938518569984,
2.29554640421059));
#82117=CARTESIAN_POINT('Ctrl Pts',(-11.9265608041214,-0.0193328538229716,
2.29056286380607));
#82118=CARTESIAN_POINT('Ctrl Pts',(-11.9271679327176,-0.115851083445451,
2.28557976100868));
#82119=CARTESIAN_POINT('Ctrl Pts',(-11.9323260429192,-0.212349219977606,
2.28059665821128));
#82120=CARTESIAN_POINT('Ctrl Pts',(-11.9420086429596,-0.3083684650972,2.27561355541389));
#82121=CARTESIAN_POINT('Ctrl Pts',(-11.9516930317545,-0.404405448722155,
2.27062953204276));
#82122=CARTESIAN_POINT('Ctrl Pts',(-11.9659035263656,-0.499962928787207,
2.26564550867162));
#82123=CARTESIAN_POINT('Ctrl Pts',(-11.9845618847413,-0.594588280279178,
2.26066148530049));
#82124=CARTESIAN_POINT('Ctrl Pts',(-12.0032402859632,-0.689315278514189,
2.25567210808142));
#82125=CARTESIAN_POINT('Ctrl Pts',(-12.0263760043518,-0.783107718157338,
2.25068273086235));
#82126=CARTESIAN_POINT('Ctrl Pts',(-12.0538399197974,-0.875524432452098,
2.24569335364328));
#82127=CARTESIAN_POINT('Ctrl Pts',(-12.0813201145038,-0.96799592683787,
2.24070101896635));
#82128=CARTESIAN_POINT('Ctrl Pts',(-12.1131334701694,-1.05908965821645,
2.23570868428941));
#82129=CARTESIAN_POINT('Ctrl Pts',(-12.1491020608473,-1.14838285886504,
2.23071634961248));
#82130=CARTESIAN_POINT('Ctrl Pts',(-12.1851282294996,-1.23781899871455,
2.22571602328194));
#82131=CARTESIAN_POINT('Ctrl Pts',(-12.2253227317514,-1.32544845441526,
2.2207156969514));
#82132=CARTESIAN_POINT('Ctrl Pts',(-12.2694609442956,-1.41087161544655,
2.21571537062085));
#82133=CARTESIAN_POINT('Ctrl Pts',(-12.2939396364568,-1.45824660282806,
2.21294223048002));
#82134=CARTESIAN_POINT('Ctrl Pts',(-12.3196305078895,-1.50494347668573,
2.21016909033918));
#82135=CARTESIAN_POINT('Ctrl Pts',(-12.3464895870466,-1.55089804253787,
2.20739595019835));
#82136=CARTESIAN_POINT('Ctrl Pts',(-12.394925277042,-1.6337691302794,2.20239507301304));
#82137=CARTESIAN_POINT('Ctrl Pts',(-12.4473313701558,-1.71451358993703,
2.19739419582773));
#82138=CARTESIAN_POINT('Ctrl Pts',(-12.5034957991935,-1.79272670124466,
2.19239331864242));
#82139=CARTESIAN_POINT('Ctrl Pts',(-12.559584374276,-1.87083418032301,2.18739919548845));
#82140=CARTESIAN_POINT('Ctrl Pts',(-12.619420943369,-1.94641675244406,2.18240507233449));
#82141=CARTESIAN_POINT('Ctrl Pts',(-12.6827483288791,-2.01909557542172,
2.17741094918052));
#82142=CARTESIAN_POINT('Ctrl Pts',(-12.7460092491569,-2.09169811836956,
2.17242206760653));
#82143=CARTESIAN_POINT('Ctrl Pts',(-12.8127534156523,-2.16140264180255,
2.16743318603254));
#82144=CARTESIAN_POINT('Ctrl Pts',(-12.8826818788696,-2.22786135653291,
2.16244430445855));
#82145=CARTESIAN_POINT('Ctrl Pts',(-12.9525606919073,-2.29427288465337,
2.15745896505973));
#82146=CARTESIAN_POINT('Ctrl Pts',(-13.0256189899682,-2.35744288417238,
2.1524736256609));
#82147=CARTESIAN_POINT('Ctrl Pts',(-13.1015199496688,-2.41705931836488,
2.14748828626208));
#82148=CARTESIAN_POINT('Ctrl Pts',(-13.1773935570037,-2.47665426863257,
2.14250474342586));
#82149=CARTESIAN_POINT('Ctrl Pts',(-13.2561074459012,-2.53269792735683,
2.13752120058965));
#82150=CARTESIAN_POINT('Ctrl Pts',(-13.337291334359,-2.58491820822289,2.13253765775343));
#82151=CARTESIAN_POINT('Ctrl Pts',(-13.4184680935616,-2.63713390330583,
2.12755455255268));
#82152=CARTESIAN_POINT('Ctrl Pts',(-13.5021140520083,-2.68552665096215,
2.12257144735193));
#82153=CARTESIAN_POINT('Ctrl Pts',(-13.5878304418918,-2.72986801680091,
2.11758834215118));
#82154=CARTESIAN_POINT('Ctrl Pts',(-13.6735626663974,-2.77421757394089,
2.11260431640783));
#82155=CARTESIAN_POINT('Ctrl Pts',(-13.7613656923181,-2.81451406135458,
2.10762029066449));
#82156=CARTESIAN_POINT('Ctrl Pts',(-13.8508176534763,-2.85057576367272,
2.10263626492115));
#82157=CARTESIAN_POINT('Ctrl Pts',(-13.9403657029619,-2.88667620308076,
2.09764688539135));
#82158=CARTESIAN_POINT('Ctrl Pts',(-14.0315658162599,-2.91853261176117,
2.09265750586156));
#82159=CARTESIAN_POINT('Ctrl Pts',(-14.1239779320351,-2.94601214974386,
2.08766812633176));
#82160=CARTESIAN_POINT('Ctrl Pts',(-14.2164448245683,-2.97350797606701,
2.08267578937552));
#82161=CARTESIAN_POINT('Ctrl Pts',(-14.3101247243823,-2.99662166081349,
2.07768345241928));
#82162=CARTESIAN_POINT('Ctrl Pts',(-14.4045663206393,-3.01527129517112,
2.07269111546304));
#82163=CARTESIAN_POINT('Ctrl Pts',(-14.4991590961543,-3.03395078330078,
2.06769078692442));
#82164=CARTESIAN_POINT('Ctrl Pts',(-14.5945155691579,-3.04815188821779,
2.0626904583858));
#82165=CARTESIAN_POINT('Ctrl Pts',(-14.6901783166036,-3.05784446538693,
2.05769012984717));
#82166=CARTESIAN_POINT('Ctrl Pts',(-14.7432316121923,-3.06321984060142,
2.05491701371699));
#82167=CARTESIAN_POINT('Ctrl Pts',(-14.7963790757514,-3.06720947326471,
2.0521438975868));
#82168=CARTESIAN_POINT('Ctrl Pts',(-14.8495429191303,-3.06981512746552,
2.04937078145661));
#82169=CARTESIAN_POINT('Ctrl Pts',(-14.945415621551,-3.07451401855257,2.04436989888999));
#82170=CARTESIAN_POINT('Ctrl Pts',(-15.0416759073252,-3.07472553622459,
2.03936901632337));
#82171=CARTESIAN_POINT('Ctrl Pts',(-15.1378689317255,-3.07040622844354,
2.03436813375675));
#82172=CARTESIAN_POINT('Ctrl Pts',(-15.2339320418076,-3.06609275414083,
2.02937400517518));
#82173=CARTESIAN_POINT('Ctrl Pts',(-15.3299276365342,-3.05726063553923,
2.02437987659362));
#82174=CARTESIAN_POINT('Ctrl Pts',(-15.4253979050383,-3.0439183419384,2.01938574801205));
#82175=CARTESIAN_POINT('Ctrl Pts',(-15.5207679736017,-3.0305900516189,2.01439686097213));
#82176=CARTESIAN_POINT('Ctrl Pts',(-15.6156133798509,-3.01276105702709,
2.00940797393221));
#82177=CARTESIAN_POINT('Ctrl Pts',(-15.7094795050446,-2.99049177927672,
2.00441908689228));
#82178=CARTESIAN_POINT('Ctrl Pts',(-15.8032789847001,-2.96823831285338,
1.99943374199349));
#82179=CARTESIAN_POINT('Ctrl Pts',(-15.8961001399201,-2.94155093162123,
1.99444839709469));
#82180=CARTESIAN_POINT('Ctrl Pts',(-15.9874976097487,-2.9105413106054,1.98946305219589));
#82181=CARTESIAN_POINT('Ctrl Pts',(-16.0788621431295,-2.87954286437116,
1.98447950384082));
#82182=CARTESIAN_POINT('Ctrl Pts',(-16.1688035955202,-2.84422541399118,
1.97949595548576));
#82183=CARTESIAN_POINT('Ctrl Pts',(-16.2568917918904,-2.80475048328343,
1.9745124071307));
#82184=CARTESIAN_POINT('Ctrl Pts',(-16.3449722529158,-2.76527901901284,
1.96952929639913));
#82185=CARTESIAN_POINT('Ctrl Pts',(-16.4311993812673,-2.72165097987983,
1.96454618566756));
#82186=CARTESIAN_POINT('Ctrl Pts',(-16.5151640047239,-2.67407559518967,
1.95956307493599));
#82187=CARTESIAN_POINT('Ctrl Pts',(-16.5991441392613,-2.62649142173107,
1.95457904365682));
#82188=CARTESIAN_POINT('Ctrl Pts',(-16.6808605571871,-2.57495867076684,
1.94959501237765));
#82189=CARTESIAN_POINT('Ctrl Pts',(-16.7599306010706,-2.51973143993866,
1.94461098109848));
#82190=CARTESIAN_POINT('Ctrl Pts',(-16.8390855806278,-2.46444488497419,
1.9396215960591));
#82191=CARTESIAN_POINT('Ctrl Pts',(-16.9155881509083,-2.40545617910367,
1.93463221101972));
#82192=CARTESIAN_POINT('Ctrl Pts',(-16.9890866539137,-2.34306135925256,
1.92964282598034));
#82193=CARTESIAN_POINT('Ctrl Pts',(-17.0626287225914,-2.28062955535191,
1.92465048352135));
#82194=CARTESIAN_POINT('Ctrl Pts',(-17.1331628579191,-2.21478791655874,
1.91965814106237));
#82195=CARTESIAN_POINT('Ctrl Pts',(-17.2003739173934,-2.14586972429713,
1.91466579860338));
#82196=CARTESIAN_POINT('Ctrl Pts',(-17.2676925653125,-2.07684121088909,
1.90966546462684));
#82197=CARTESIAN_POINT('Ctrl Pts',(-17.3316772251645,-2.00472663850662,
1.9046651306503));
#82198=CARTESIAN_POINT('Ctrl Pts',(-17.3920527740801,-1.92989268510343,
1.89966479667376));
#82199=CARTESIAN_POINT('Ctrl Pts',(-17.4255355574571,-1.88839162886379,
1.89689173535412));
#82200=CARTESIAN_POINT('Ctrl Pts',(-17.4579091067308,-1.8460547513915,1.89411867403449));
#82201=CARTESIAN_POINT('Ctrl Pts',(-17.4891324092414,-1.80294816876802,
1.89134561271486));
#82202=CARTESIAN_POINT('Ctrl Pts',(-17.5458129998629,-1.72469550597112,
1.88631159194231));
#82203=CARTESIAN_POINT('Ctrl Pts',(-17.5988982171272,-1.64363182743569,
1.88127757116976));
#82204=CARTESIAN_POINT('Ctrl Pts',(-17.6480998096016,-1.56011847254879,
1.87624355039721));
#82205=CARTESIAN_POINT('Ctrl Pts',(-17.6972334799748,-1.47672040666498,
1.87121647901901));
#82206=CARTESIAN_POINT('Ctrl Pts',(-17.7424939640519,-1.39087975307624,
1.86618940764081));
#82207=CARTESIAN_POINT('Ctrl Pts',(-17.783634744614,-1.30298881751823,1.8611623362626));
#82208=CARTESIAN_POINT('Ctrl Pts',(-17.8247294327806,-1.21519635125798,
1.85614089700318));
#82209=CARTESIAN_POINT('Ctrl Pts',(-17.8617134114388,-1.12535855738384,
1.85111945774376));
#82210=CARTESIAN_POINT('Ctrl Pts',(-17.8943852860642,-1.03389364337698,
1.84609801848433));
#82211=CARTESIAN_POINT('Ctrl Pts',(-17.9270269589727,-0.942513279077256,
1.84108122101814));
#82212=CARTESIAN_POINT('Ctrl Pts',(-17.9553643136507,-0.849509191330882,
1.83606442355194));
#82213=CARTESIAN_POINT('Ctrl Pts',(-17.97924386297,-0.755319968593296,1.83104762608575));
#82214=CARTESIAN_POINT('Ctrl Pts',(-18.0031103269534,-0.661182358957654,
1.8260335776865));
#82215=CARTESIAN_POINT('Ctrl Pts',(-18.0225237378336,-0.565861322705995,
1.82101952928725));
#82216=CARTESIAN_POINT('Ctrl Pts',(-18.0373805448444,-0.469810255103615,
1.81600548088801));
#82217=CARTESIAN_POINT('Ctrl Pts',(-18.0522352245164,-0.373772941005991,
1.81099215044787));
#82218=CARTESIAN_POINT('Ctrl Pts',(-18.0625345258306,-0.277006228114954,
1.80597882000772));
#82219=CARTESIAN_POINT('Ctrl Pts',(-18.068226216715,-0.179972589753701,
1.80096548956758));
#82220=CARTESIAN_POINT('Ctrl Pts',(-18.0717793388245,-0.119397907674138,
1.7978358439859));
#82221=CARTESIAN_POINT('Ctrl Pts',(-18.0735378699228,-0.0587193639364806,
1.79470619840423));
#82222=CARTESIAN_POINT('Ctrl Pts',(-18.0734993815187,0.00194982156482441,
1.79157655282255));
#82223=CARTESIAN_POINT('Origin',(-15.,0.,8.20842344717746));
#82224=CARTESIAN_POINT('',(-13.1276888212995,2.43738653071547,3.43723390425693));
#82225=CARTESIAN_POINT('',(-13.1276888212995,2.43738653071547,3.3542649531753));
#82226=CARTESIAN_POINT('',(-13.1276888212995,2.43738653071547,8.20842344717746));
#82227=CARTESIAN_POINT('',(-18.073499222413,0.00218628150294359,2.70842344717746));
#82228=CARTESIAN_POINT('Ctrl Pts',(-13.1276888212995,2.43738653071547,3.3542649531753));
#82229=CARTESIAN_POINT('Ctrl Pts',(-13.0512005964765,2.37863107417608,3.34927198847025));
#82230=CARTESIAN_POINT('Ctrl Pts',(-12.9775534946703,2.31632766092925,3.3442790237652));
#82231=CARTESIAN_POINT('Ctrl Pts',(-12.9070773460554,2.25079475177229,3.33928605906015));
#82232=CARTESIAN_POINT('Ctrl Pts',(-12.8364918224869,2.18516013928675,3.33428534555933));
#82233=CARTESIAN_POINT('Ctrl Pts',(-12.7690873807666,2.11628633992039,3.3292846320585));
#82234=CARTESIAN_POINT('Ctrl Pts',(-12.7051552920996,2.04452684419193,3.32428391855767));
#82235=CARTESIAN_POINT('Ctrl Pts',(-12.680628582491,2.01699725224389,3.3223654602306));
#82236=CARTESIAN_POINT('Ctrl Pts',(-12.6566124837819,1.98904327447208,3.32044700190352));
#82237=CARTESIAN_POINT('Ctrl Pts',(-12.6331217549234,1.9606860082591,3.31852854357645));
#82238=CARTESIAN_POINT('Ctrl Pts',(-12.5718880904872,1.88676666186203,3.31352766709695));
#82239=CARTESIAN_POINT('Ctrl Pts',(-12.5140137541319,1.80984705634736,3.30852679061746));
#82240=CARTESIAN_POINT('Ctrl Pts',(-12.4598061902056,1.73026519894555,3.30352591413796));
#82241=CARTESIAN_POINT('Ctrl Pts',(-12.4056718372278,1.65079082217648,3.29853179167736));
#82242=CARTESIAN_POINT('Ctrl Pts',(-12.3551946591348,1.56866169907131,3.29353766921675));
#82243=CARTESIAN_POINT('Ctrl Pts',(-12.3086423207339,1.48424933628268,3.28854354675615));
#82244=CARTESIAN_POINT('Ctrl Pts',(-12.2621388412056,1.39992556824611,3.28355466586238));
#82245=CARTESIAN_POINT('Ctrl Pts',(-12.2195522230033,1.31332370657085,3.27856578496861));
#82246=CARTESIAN_POINT('Ctrl Pts',(-12.1811066352899,1.22484384653443,3.27357690407484));
#82247=CARTESIAN_POINT('Ctrl Pts',(-12.1426883443105,1.13642680804277,3.2685915653341));
#82248=CARTESIAN_POINT('Ctrl Pts',(-12.1084054131327,1.04613482315557,3.26360622659336));
#82249=CARTESIAN_POINT('Ctrl Pts',(-12.0784354376814,0.95439130245612,3.25862088785262));
#82250=CARTESIAN_POINT('Ctrl Pts',(-12.048476262403,0.862680843041611,3.2536373456606));
#82251=CARTESIAN_POINT('Ctrl Pts',(-12.0228270907301,0.769520303724429,
3.24865380346858));
#82252=CARTESIAN_POINT('Ctrl Pts',(-12.0016165162505,0.675350823186146,
3.24367026127656));
#82253=CARTESIAN_POINT('Ctrl Pts',(-11.9804078043398,0.581189611973402,
3.23868715670544));
#82254=CARTESIAN_POINT('Ctrl Pts',(-11.9636370108476,0.4860200636921,3.23370405213432));
#82255=CARTESIAN_POINT('Ctrl Pts',(-11.9513819554675,0.390295104441535,
3.2287209475632));
#82256=CARTESIAN_POINT('Ctrl Pts',(-11.9391246361399,0.294552461363366,
3.22373692243424));
#82257=CARTESIAN_POINT('Ctrl Pts',(-11.9313847673773,0.198254638653824,
3.21875289730527));
#82258=CARTESIAN_POINT('Ctrl Pts',(-11.9281883615582,0.101860237252839,
3.2137688721763));
#82259=CARTESIAN_POINT('Ctrl Pts',(-11.9249885221769,0.00536228950122442,
3.20877949323419));
#82260=CARTESIAN_POINT('Ctrl Pts',(-11.926341903648,-0.0912320049161493,
3.20379011429208));
#82261=CARTESIAN_POINT('Ctrl Pts',(-11.9322223670329,-0.187463715600849,
3.19880073534997));
#82262=CARTESIAN_POINT('Ctrl Pts',(-11.9381063160463,-0.283752467368255,
3.19380839896716));
#82263=CARTESIAN_POINT('Ctrl Pts',(-11.9485226428087,-0.379677771578006,
3.18881606258436));
#82264=CARTESIAN_POINT('Ctrl Pts',(-11.96339350805,-0.474787597823518,3.18382372620156));
#82265=CARTESIAN_POINT('Ctrl Pts',(-11.9782881782089,-0.570049673554757,
3.17882339820867));
#82266=CARTESIAN_POINT('Ctrl Pts',(-11.9976515367199,-0.664493235451254,
3.17382307021578));
#82267=CARTESIAN_POINT('Ctrl Pts',(-12.0213550232632,-0.757678264542756,
3.16882274222289));
#82268=CARTESIAN_POINT('Ctrl Pts',(-12.0345006951214,-0.809357573926145,
3.16604961976017));
#82269=CARTESIAN_POINT('Ctrl Pts',(-12.0489803672796,-0.860650087863547,
3.16327649729744));
#82270=CARTESIAN_POINT('Ctrl Pts',(-12.0647657044095,-0.91148334048911,
3.16050337483472));
#82271=CARTESIAN_POINT('Ctrl Pts',(-12.0932319989279,-1.00315286446984,
3.15550249838146));
#82272=CARTESIAN_POINT('Ctrl Pts',(-12.126046426735,-1.09364749385214,3.15050162192819));
#82273=CARTESIAN_POINT('Ctrl Pts',(-12.1630938131952,-1.18252506834685,
3.14550074547493));
#82274=CARTESIAN_POINT('Ctrl Pts',(-12.2000911647162,-1.27128260781442,
3.1405066230352));
#82275=CARTESIAN_POINT('Ctrl Pts',(-12.2413099453687,-1.35842703143618,
3.13551250059547));
#82276=CARTESIAN_POINT('Ctrl Pts',(-12.2865851908717,-1.44353119938691,
3.13051837815574));
#82277=CARTESIAN_POINT('Ctrl Pts',(-12.3318129179195,-1.52854604659407,
3.1255294972775));
#82278=CARTESIAN_POINT('Ctrl Pts',(-12.3810884411476,-1.61152450983249,
3.12054061639926));
#82279=CARTESIAN_POINT('Ctrl Pts',(-12.4341990900186,-1.69206026498422,
3.11555173552103));
#82280=CARTESIAN_POINT('Ctrl Pts',(-12.4872720299071,-1.77253883911039,
3.11056639678782));
#82281=CARTESIAN_POINT('Ctrl Pts',(-12.5441744414,-1.85057778781918,3.10558105805462));
#82282=CARTESIAN_POINT('Ctrl Pts',(-12.6046486835395,-1.92579706114918,
3.10059571932141));
#82283=CARTESIAN_POINT('Ctrl Pts',(-12.6651011328523,-2.00098922805294,
3.09561217713198));
#82284=CARTESIAN_POINT('Ctrl Pts',(-12.7291225806967,-2.07336339700366,
3.09062863494254));
#82285=CARTESIAN_POINT('Ctrl Pts',(-12.7964137686971,-2.14257087892379,
3.0856450927531));
#82286=CARTESIAN_POINT('Ctrl Pts',(-12.8636990477083,-2.21177228358065,
3.08066198817962));
#82287=CARTESIAN_POINT('Ctrl Pts',(-12.9342531900463,-2.2778072397267,3.07567888360613));
#82288=CARTESIAN_POINT('Ctrl Pts',(-13.0077393281836,-2.34036314821731,
3.07069577903264));
#82289=CARTESIAN_POINT('Ctrl Pts',(-13.0812390419149,-2.40293061308626,
3.06571175389636));
#82290=CARTESIAN_POINT('Ctrl Pts',(-13.1576714931271,-2.46201746954657,
3.06072772876008));
#82291=CARTESIAN_POINT('Ctrl Pts',(-13.2366667606056,-2.51735141306231,
3.0557437036238));
#82292=CARTESIAN_POINT('Ctrl Pts',(-13.3157468844965,-2.57274479608733,
3.05075432466689));
#82293=CARTESIAN_POINT('Ctrl Pts',(-13.397394960687,-2.62437696604428,3.04576494570998));
#82294=CARTESIAN_POINT('Ctrl Pts',(-13.481212303729,-2.67201912112464,3.04077556675307));
#82295=CARTESIAN_POINT('Ctrl Pts',(-13.5650793293426,-2.71968951600236,
3.03578323035122));
#82296=CARTESIAN_POINT('Ctrl Pts',(-13.651117791172,-2.76336498825401,3.03079089394936));
#82297=CARTESIAN_POINT('Ctrl Pts',(-13.7389065413854,-2.80286381021972,
3.02579855754751));
#82298=CARTESIAN_POINT('Ctrl Pts',(-13.8268358217984,-2.84242586098552,
3.02079822952907));
#82299=CARTESIAN_POINT('Ctrl Pts',(-13.9165205772469,-2.87779775093621,
3.01579790151064));
#82300=CARTESIAN_POINT('Ctrl Pts',(-14.0075220138788,-2.90884679848645,
3.01079757349221));
#82301=CARTESIAN_POINT('Ctrl Pts',(-14.0579903286513,-2.92606623109265,
3.0080244510258));
#82302=CARTESIAN_POINT('Ctrl Pts',(-14.1088633714619,-2.9419569941894,3.00525132855939));
#82303=CARTESIAN_POINT('Ctrl Pts',(-14.1600649653456,-2.95650323652116,
3.00247820609297));
#82304=CARTESIAN_POINT('Ctrl Pts',(-14.252398734525,-2.9827350250264,2.99747732955187));
#82305=CARTESIAN_POINT('Ctrl Pts',(-14.3461236146214,-3.00468295413524,
2.99247645301077));
#82306=CARTESIAN_POINT('Ctrl Pts',(-14.4408063302793,-3.02220196044941,
2.98747557646967));
#82307=CARTESIAN_POINT('Ctrl Pts',(-14.5353611706074,-3.03969730617577,
2.98248145394627));
#82308=CARTESIAN_POINT('Ctrl Pts',(-14.6308708477552,-3.0527755381568,2.97748733142286));
#82309=CARTESIAN_POINT('Ctrl Pts',(-14.7268874695359,-3.06134150262651,
2.97249320889945));
#82310=CARTESIAN_POINT('Ctrl Pts',(-14.8228033173709,-3.06989847671494,
2.96750432794175));
#82311=CARTESIAN_POINT('Ctrl Pts',(-14.9192246174675,-3.07395255926622,
2.96251544698405));
#82312=CARTESIAN_POINT('Ctrl Pts',(-15.0156948530631,-3.07345992679054,
2.95752656602635));
#82313=CARTESIAN_POINT('Ctrl Pts',(-15.1120965939003,-3.07296764408847,
2.95254122722022));
#82314=CARTESIAN_POINT('Ctrl Pts',(-15.208546763739,-3.06793506622035,2.94755588841409));
#82315=CARTESIAN_POINT('Ctrl Pts',(-15.3045862878005,-3.05837039013981,
2.94257054960795));
#82316=CARTESIAN_POINT('Ctrl Pts',(-15.4005912024592,-3.04880916084568,
2.93758700734965));
#82317=CARTESIAN_POINT('Ctrl Pts',(-15.4961853293009,-3.03471912188065,
2.93260346509135));
#82318=CARTESIAN_POINT('Ctrl Pts',(-15.5909131278633,-3.01616046080423,
2.92761992283305));
#82319=CARTESIAN_POINT('Ctrl Pts',(-15.6856326080882,-2.99760342942058,
2.92263681819482));
#82320=CARTESIAN_POINT('Ctrl Pts',(-15.7794854808445,-2.97457864067198,
2.9176537135566));
#82321=CARTESIAN_POINT('Ctrl Pts',(-15.8720258906693,-2.94719749864211,
2.91267060891838));
#82322=CARTESIAN_POINT('Ctrl Pts',(-15.9645833960353,-2.91981129833078,
2.90768658372155));
#82323=CARTESIAN_POINT('Ctrl Pts',(-16.0558275363149,-2.88806727092228,
2.90270255852472));
#82324=CARTESIAN_POINT('Ctrl Pts',(-16.1453281514182,-2.85212651815606,
2.8977185333279));
#82325=CARTESIAN_POINT('Ctrl Pts',(-16.2349249076165,-2.81614715802023,
2.89272915431714));
#82326=CARTESIAN_POINT('Ctrl Pts',(-16.3227739919592,-2.77596223648105,
2.88773977530638));
#82327=CARTESIAN_POINT('Ctrl Pts',(-16.4084659700617,-2.73178071249838,
2.88275039629561));
#82328=CARTESIAN_POINT('Ctrl Pts',(-16.4942087418581,-2.68757300003394,
2.87775805984361));
#82329=CARTESIAN_POINT('Ctrl Pts',(-16.5777914816568,-2.63936418712446,
2.87276572339161));
#82330=CARTESIAN_POINT('Ctrl Pts',(-16.6588319147118,-2.58740776236247,
2.8677733869396));
#82331=CARTESIAN_POINT('Ctrl Pts',(-16.7400020753135,-2.53536816702421,
2.86277305887729));
#82332=CARTESIAN_POINT('Ctrl Pts',(-16.8186214458339,-2.47956923514097,
2.85777273081498));
#82333=CARTESIAN_POINT('Ctrl Pts',(-16.8943391938762,-2.42030602787013,
2.85277240275267));
#82334=CARTESIAN_POINT('Ctrl Pts',(-16.9363313462235,-2.38743936592297,
2.8499992809522));
#82335=CARTESIAN_POINT('Ctrl Pts',(-16.9774316737466,-2.35350789689179,
2.84722615915172));
#82336=CARTESIAN_POINT('Ctrl Pts',(-17.0175852866678,-2.31856676872189,
2.84445303735124));
#82337=CARTESIAN_POINT('Ctrl Pts',(-17.0889589316375,-2.25645839302651,
2.83952377205118));
#82338=CARTESIAN_POINT('Ctrl Pts',(-17.1576039115037,-2.19092748187001,
2.83459450675111));
#82339=CARTESIAN_POINT('Ctrl Pts',(-17.2231671496839,-2.12224646885475,
2.82966524145105));
#82340=CARTESIAN_POINT('Ctrl Pts',(-17.2903594199941,-2.05185895719735,
2.82461350002298));
#82341=CARTESIAN_POINT('Ctrl Pts',(-17.3543143585099,-1.97816296494052,
2.81956175859491));
#82342=CARTESIAN_POINT('Ctrl Pts',(-17.4146868794231,-1.90149665378145,
2.81451001716685));
#82343=CARTESIAN_POINT('Ctrl Pts',(-17.4734480008263,-1.82687663875776,
2.80959311148091));
#82344=CARTESIAN_POINT('Ctrl Pts',(-17.52881521957,-1.74944324297213,2.80467620579497));
#82345=CARTESIAN_POINT('Ctrl Pts',(-17.5805078919353,-1.66954522839601,
2.79975930010903));
#82346=CARTESIAN_POINT('Ctrl Pts',(-17.6321694728631,-1.58969526984033,
2.79484535177968));
#82347=CARTESIAN_POINT('Ctrl Pts',(-17.6801606504181,-1.50738401458739,
2.78993140345033));
#82348=CARTESIAN_POINT('Ctrl Pts',(-17.724242835189,-1.42299094337295,2.78501745512099));
#82349=CARTESIAN_POINT('Ctrl Pts',(-17.7683113470811,-1.33862404818035,
2.78010503094069));
#82350=CARTESIAN_POINT('Ctrl Pts',(-17.8084730657097,-1.25217702067679,
2.77519260676039));
#82351=CARTESIAN_POINT('Ctrl Pts',(-17.8445349215123,-1.1640546938597,2.77028018258008));
#82352=CARTESIAN_POINT('Ctrl Pts',(-17.8823755169536,-1.07158576112708,
2.76512545462987));
#82353=CARTESIAN_POINT('Ctrl Pts',(-17.9157011777319,-0.977272502073842,
2.75997072667965));
#82354=CARTESIAN_POINT('Ctrl Pts',(-17.9443460255526,-0.881605768931114,
2.75481599872943));
#82355=CARTESIAN_POINT('Ctrl Pts',(-17.9716643411015,-0.790369326695886,
2.74989998431753));
#82356=CARTESIAN_POINT('Ctrl Pts',(-17.9947256424304,-0.69790244673538,
2.74498396990564));
#82357=CARTESIAN_POINT('Ctrl Pts',(-18.0134378458492,-0.604644192234935,
2.74006795549375));
#82358=CARTESIAN_POINT('Ctrl Pts',(-18.032158764123,-0.511342504466295,
2.73514965154112));
#82359=CARTESIAN_POINT('Ctrl Pts',(-18.0465264852592,-0.417249155543324,
2.73023134758849));
#82360=CARTESIAN_POINT('Ctrl Pts',(-18.056500603696,-0.322810020919425,
2.72531304363586));
#82361=CARTESIAN_POINT('Ctrl Pts',(-18.0664867611952,-0.228256895406328,
2.72038880314175));
#82362=CARTESIAN_POINT('Ctrl Pts',(-18.0720687134541,-0.133357602149294,
2.71546456264763));
#82363=CARTESIAN_POINT('Ctrl Pts',(-18.0732581163465,-0.0385590496523394,
2.71054032215352));
#82364=CARTESIAN_POINT('Ctrl Pts',(-18.0734285532713,-0.0249747765184603,
2.7098346971615));
#82365=CARTESIAN_POINT('Ctrl Pts',(-18.0735088814944,-0.0113925642842438,
2.70912907216948));
#82366=CARTESIAN_POINT('Ctrl Pts',(-18.073499222413,0.00218628150294359,
2.70842344717746));
#82367=CARTESIAN_POINT('Ctrl Pts',(-18.0762767414075,0.00218825724393669,
2.70842344717746));
#82368=CARTESIAN_POINT('Ctrl Pts',(-18.0774175670185,0.143408855469269,
2.70109158765481));
#82369=CARTESIAN_POINT('Ctrl Pts',(-18.0046436801636,1.2980338168667,2.64108467188491));
#82370=CARTESIAN_POINT('Ctrl Pts',(-16.5438880884248,3.28204007054153,2.52840269986777));
#82371=CARTESIAN_POINT('Ctrl Pts',(-14.1255737879022,3.14463322099092,2.41762057516619));
#82372=CARTESIAN_POINT('Ctrl Pts',(-13.2078714909188,2.50458144295651,2.35951350671185));
#82373=CARTESIAN_POINT('Ctrl Pts',(-13.1254325828889,2.44028101900739,2.35408149450477));
#82374=CARTESIAN_POINT('',(-18.0734989461686,-0.00254517198238653,2.79157655284933));
#82375=CARTESIAN_POINT('Ctrl Pts',(-18.073498946169,-0.00254517146422184,
2.79157655282255));
#82376=CARTESIAN_POINT('Ctrl Pts',(-18.0735783970018,0.0933980898477828,
2.78661850057295));
#82377=CARTESIAN_POINT('Ctrl Pts',(-18.0691610737691,0.189417023051302,
2.78166044832335));
#82378=CARTESIAN_POINT('Ctrl Pts',(-18.0602524559986,0.285056407671365,
2.77670239607375));
#82379=CARTESIAN_POINT('Ctrl Pts',(-18.0513467904042,0.380664098900641,
2.77174598684483));
#82380=CARTESIAN_POINT('Ctrl Pts',(-18.0379528279,0.47589204991766,2.76678957761592));
#82381=CARTESIAN_POINT('Ctrl Pts',(-18.0201280577465,0.570288317267858,
2.76183316838701));
#82382=CARTESIAN_POINT('Ctrl Pts',(-18.0023042035091,0.664679734117188,
2.75687701384049));
#82383=CARTESIAN_POINT('Ctrl Pts',(-17.980050077036,0.75823911624815,2.75192085929396));
#82384=CARTESIAN_POINT('Ctrl Pts',(-17.9534744186567,0.850524019849157,
2.74696470474744));
#82385=CARTESIAN_POINT('Ctrl Pts',(-17.9268926845698,0.942830021557655,
2.74200741712848));
#82386=CARTESIAN_POINT('Ctrl Pts',(-17.895987579697,1.03386053982986,2.73705012950952));
#82387=CARTESIAN_POINT('Ctrl Pts',(-17.8609175744308,1.12318871179908,2.73209284189055));
#82388=CARTESIAN_POINT('Ctrl Pts',(-17.8258083482045,1.21261678499865,2.72713001022964));
#82389=CARTESIAN_POINT('Ctrl Pts',(-17.7865250883768,1.3003382988599,2.72216717856873));
#82390=CARTESIAN_POINT('Ctrl Pts',(-17.743274126476,1.38594708304738,2.71720434690782));
#82391=CARTESIAN_POINT('Ctrl Pts',(-17.6999952881571,1.47161104441819,2.7122383165673));
#82392=CARTESIAN_POINT('Ctrl Pts',(-17.652743876713,1.55515918054058,2.70727228622678));
#82393=CARTESIAN_POINT('Ctrl Pts',(-17.6017707263958,1.63621249759002,2.70230625588626));
#82394=CARTESIAN_POINT('Ctrl Pts',(-17.5507164815259,1.71739476453662,2.6973323249548));
#82395=CARTESIAN_POINT('Ctrl Pts',(-17.4959289345585,1.79607392841621,2.69235839402335));
#82396=CARTESIAN_POINT('Ctrl Pts',(-17.4377003472425,1.87190257947729,2.6873844630919));
#82397=CARTESIAN_POINT('Ctrl Pts',(-17.4146263084971,1.90195093395825,2.68541346086911));
#82398=CARTESIAN_POINT('Ctrl Pts',(-17.391012352214,1.93155207610088,2.68344245864633));
#82399=CARTESIAN_POINT('Ctrl Pts',(-17.3668782450813,1.96068600825349,2.68147145642355));
#82400=CARTESIAN_POINT('Ctrl Pts',(-17.305644579888,2.03460535556479,2.67647057988226));
#82401=CARTESIAN_POINT('Ctrl Pts',(-17.2408379417085,2.10578234896841,2.67146970334098));
#82402=CARTESIAN_POINT('Ctrl Pts',(-17.1727332236773,2.17385201629014,2.6664688267997));
#82403=CARTESIAN_POINT('Ctrl Pts',(-17.1047204856153,2.24182975098103,2.6614747042761));
#82404=CARTESIAN_POINT('Ctrl Pts',(-17.0334188281061,2.30670819283883,2.6564805817525));
#82405=CARTESIAN_POINT('Ctrl Pts',(-16.9591434609307,2.36815522073461,2.6514864592289));
#82406=CARTESIAN_POINT('Ctrl Pts',(-16.8849460492348,2.42953775709419,2.646497578271));
#82407=CARTESIAN_POINT('Ctrl Pts',(-16.8077814686798,2.48749576090924,2.64150869731309));
#82408=CARTESIAN_POINT('Ctrl Pts',(-16.7280011121749,2.5417345271138,2.63651981635519));
#82409=CARTESIAN_POINT('Ctrl Pts',(-16.6482774004602,2.59593478329323,2.63153447754886));
#82410=CARTESIAN_POINT('Ctrl Pts',(-16.5659419666771,2.64642080558076,2.62654913874253));
#82411=CARTESIAN_POINT('Ctrl Pts',(-16.4813777783395,2.6929393100926,2.6215637999362));
#82412=CARTESIAN_POINT('Ctrl Pts',(-16.3968440640809,2.73944105090565,2.6165802576777));
#82413=CARTESIAN_POINT('Ctrl Pts',(-16.3100835750895,2.78197790357921,2.6115967154192));
#82414=CARTESIAN_POINT('Ctrl Pts',(-16.2215058158792,2.82034143177264,2.6066131731607));
#82415=CARTESIAN_POINT('Ctrl Pts',(-16.1329358349526,2.85870159114742,2.60163006852227));
#82416=CARTESIAN_POINT('Ctrl Pts',(-16.0425493037159,2.89288898053685,2.59664696388384));
#82417=CARTESIAN_POINT('Ctrl Pts',(-15.9507767564214,2.92274285722311,2.59166385924542));
#82418=CARTESIAN_POINT('Ctrl Pts',(-15.8589872554378,2.95260224899378,2.5866798340484));
#82419=CARTESIAN_POINT('Ctrl Pts',(-15.7658116470334,2.97812640246882,2.58169580885138));
#82420=CARTESIAN_POINT('Ctrl Pts',(-15.6716956816881,2.99920442137602,2.57671178365436));
#82421=CARTESIAN_POINT('Ctrl Pts',(-15.5774786174622,3.02030508218155,2.57172240464339));
#82422=CARTESIAN_POINT('Ctrl Pts',(-15.4823196084789,3.03694997776553,2.56673302563242));
#82423=CARTESIAN_POINT('Ctrl Pts',(-15.3866744334398,3.0490793909841,2.56174364662145));
#82424=CARTESIAN_POINT('Ctrl Pts',(-15.2909725649758,3.06121599388034,2.55675131016924));
#82425=CARTESIAN_POINT('Ctrl Pts',(-15.1947843937238,3.0688317503288,2.55175897371703));
#82426=CARTESIAN_POINT('Ctrl Pts',(-15.0985685395066,3.07191902448934,2.54676663726483));
#82427=CARTESIAN_POINT('Ctrl Pts',(-15.0021986652989,3.07501124068298,2.54176630920231));
#82428=CARTESIAN_POINT('Ctrl Pts',(-14.9058014579086,3.07356050693218,2.53676598113979));
#82429=CARTESIAN_POINT('Ctrl Pts',(-14.8098331738837,3.06761125767997,2.53176565307727));
#82430=CARTESIAN_POINT('Ctrl Pts',(-14.75661031789,3.0643118756035,2.52899253127878));
#82431=CARTESIAN_POINT('Ctrl Pts',(-14.7035192655416,3.05962981734055,2.52621940948029));
#82432=CARTESIAN_POINT('Ctrl Pts',(-14.6506364896964,3.05357943857178,2.52344628768181));
#82433=CARTESIAN_POINT('Ctrl Pts',(-14.5552763385047,3.04266917478673,2.51844569325858));
#82434=CARTESIAN_POINT('Ctrl Pts',(-14.4602614050597,3.02726860095593,2.51344509883535));
#82435=CARTESIAN_POINT('Ctrl Pts',(-14.366047481739,3.00740859455288,2.50844450441211));
#82436=CARTESIAN_POINT('Ctrl Pts',(-14.2719552305796,2.98757423626868,2.50345036798479));
#82437=CARTESIAN_POINT('Ctrl Pts',(-14.1786623596624,2.96329197809384,2.49845623155747));
#82438=CARTESIAN_POINT('Ctrl Pts',(-14.0866192495522,2.93464441708216,2.49346209513014));
#82439=CARTESIAN_POINT('Ctrl Pts',(-13.9946812594751,2.90602957370198,2.48847366237564));
#82440=CARTESIAN_POINT('Ctrl Pts',(-13.903990607949,2.8730594729685,2.48348522962115));
#82441=CARTESIAN_POINT('Ctrl Pts',(-13.8149859797168,2.83586741963234,2.47849679686665));
#82442=CARTESIAN_POINT('Ctrl Pts',(-13.726041367859,2.79870044512907,2.47351172784338));
#82443=CARTESIAN_POINT('Ctrl Pts',(-13.638780923381,2.75731734429835,2.46852665882011));
#82444=CARTESIAN_POINT('Ctrl Pts',(-13.5536259359272,2.71190049905551,2.46354158979685));
#82445=CARTESIAN_POINT('Ctrl Pts',(-13.4684942244174,2.66649606788231,2.45855788337359));
#82446=CARTESIAN_POINT('Ctrl Pts',(-13.3854672157398,2.61706028423352,2.45357417695034));
#82447=CARTESIAN_POINT('Ctrl Pts',(-13.3049432397788,2.56382230851289,2.44859047052709));
#82448=CARTESIAN_POINT('Ctrl Pts',(-13.244390459308,2.52378817683913,2.44484280062658));
#82449=CARTESIAN_POINT('Ctrl Pts',(-13.1852526641704,2.48160496925117,2.44109513072608));
#82450=CARTESIAN_POINT('Ctrl Pts',(-13.1276888212995,2.43738653071547,2.43734746082558));
#82451=CARTESIAN_POINT('Ctrl Pts',(-13.1276888212995,2.43738653071547,3.43723390425693));
#82452=CARTESIAN_POINT('Ctrl Pts',(-13.0487694023508,2.37676351977643,3.4320813303875));
#82453=CARTESIAN_POINT('Ctrl Pts',(-12.9727177480323,2.31224249060819,3.42692875651806));
#82454=CARTESIAN_POINT('Ctrl Pts',(-12.8999347369254,2.24413193480849,3.42177618264863));
#82455=CARTESIAN_POINT('Ctrl Pts',(-12.8295244108795,2.17824174466537,3.41679157977764));
#82456=CARTESIAN_POINT('Ctrl Pts',(-12.7621732628445,2.10899276086274,3.41180697690666));
#82457=CARTESIAN_POINT('Ctrl Pts',(-12.698210607387,2.03670514362153,3.40682237403567));
#82458=CARTESIAN_POINT('Ctrl Pts',(-12.6342653270429,1.96443716292499,3.4018391252054));
#82459=CARTESIAN_POINT('Ctrl Pts',(-12.5737070006539,1.88913251742462,3.39685587637513));
#82460=CARTESIAN_POINT('Ctrl Pts',(-12.5168267268034,1.81114680390137,3.39187262754486));
#82461=CARTESIAN_POINT('Ctrl Pts',(-12.4599464013209,1.73316101958798,3.38688937419114));
#82462=CARTESIAN_POINT('Ctrl Pts',(-12.4067443928656,1.65249451735772,3.38190612083741));
#82463=CARTESIAN_POINT('Ctrl Pts',(-12.357469641323,1.56953354646232,3.37692286748369));
#82464=CARTESIAN_POINT('Ctrl Pts',(-12.3081814153039,1.48654988939138,3.37193825142941));
#82465=CARTESIAN_POINT('Ctrl Pts',(-12.2628228034069,1.40127089438487,3.36695363537514));
#82466=CARTESIAN_POINT('Ctrl Pts',(-12.2215972575323,1.31410823399282,3.36196901932087));
#82467=CARTESIAN_POINT('Ctrl Pts',(-12.1803254865548,1.22684784043912,3.35697881414983));
#82468=CARTESIAN_POINT('Ctrl Pts',(-12.1431962169842,1.13769996377204,3.35198860897879));
#82469=CARTESIAN_POINT('Ctrl Pts',(-12.110365000904,1.04709685416357,3.34699840380776));
#82470=CARTESIAN_POINT('Ctrl Pts',(-12.0775117119113,0.956432830743878,
3.34200484364794));
#82471=CARTESIAN_POINT('Ctrl Pts',(-12.0489623581175,0.864312045096493,
3.33701128348813));
#82472=CARTESIAN_POINT('Ctrl Pts',(-12.0248222175848,0.771180532056574,
3.33201772332832));
#82473=CARTESIAN_POINT('Ctrl Pts',(-12.000645641924,0.677908454027049,3.32701662630253));
#82474=CARTESIAN_POINT('Ctrl Pts',(-11.9808916476761,0.58362303269245,3.32201552927674));
#82475=CARTESIAN_POINT('Ctrl Pts',(-11.9656141365388,0.488778765523918,
3.31701443225095));
#82476=CARTESIAN_POINT('Ctrl Pts',(-11.9621089196193,0.467018039773852,
3.3158669986308));
#82477=CARTESIAN_POINT('Ctrl Pts',(-11.9588391329913,0.445227906867683,
3.31471956501064));
#82478=CARTESIAN_POINT('Ctrl Pts',(-11.9558050410964,0.423413866312542,
3.31357213139049));
#82479=CARTESIAN_POINT('Ctrl Pts',(-11.9425815121966,0.328341401241128,
3.30857125397406));
#82480=CARTESIAN_POINT('Ctrl Pts',(-11.9337929567606,0.232483018086391,
3.30357037655762));
#82481=CARTESIAN_POINT('Ctrl Pts',(-11.9295231862109,0.136287879077004,
3.29856949914118));
#82482=CARTESIAN_POINT('Ctrl Pts',(-11.9252591822595,0.0402226577582837,
3.29357537572969));
#82483=CARTESIAN_POINT('Ctrl Pts',(-11.9255018531107,-0.0561779809558096,
3.2885812523182));
#82484=CARTESIAN_POINT('Ctrl Pts',(-11.930283559738,-0.152457293643444,
3.28358712890672));
#82485=CARTESIAN_POINT('Ctrl Pts',(-11.9350602477518,-0.248635556916652,
3.27859824704954));
#82486=CARTESIAN_POINT('Ctrl Pts',(-11.9443664793168,-0.344692311475923,
3.27360936519236));
#82487=CARTESIAN_POINT('Ctrl Pts',(-11.9581825858215,-0.440169363768726,
3.26862048333518));
#82488=CARTESIAN_POINT('Ctrl Pts',(-11.9719888828012,-0.535578626736652,
3.2636351436164));
#82489=CARTESIAN_POINT('Ctrl Pts',(-11.9902986264711,-0.630408572754681,
3.25864980389762));
#82490=CARTESIAN_POINT('Ctrl Pts',(-12.0130402732352,-0.724205661870558,
3.25366446417884));
#82491=CARTESIAN_POINT('Ctrl Pts',(-12.0357737247145,-0.817968949834355,
3.2486809210001));
#82492=CARTESIAN_POINT('Ctrl Pts',(-12.0629358026725,-0.910699694556035,
3.24369737782135));
#82493=CARTESIAN_POINT('Ctrl Pts',(-12.0944039597898,-1.00195503946786,
3.23871383464261));
#82494=CARTESIAN_POINT('Ctrl Pts',(-12.1258693536345,-1.09320237109201,
3.2337307290773));
#82495=CARTESIAN_POINT('Ctrl Pts',(-12.1616399316239,-1.18297414586291,
3.228747623512));
#82496=CARTESIAN_POINT('Ctrl Pts',(-12.2015437591438,-1.27084417534677,
3.22376451794669));
#82497=CARTESIAN_POINT('Ctrl Pts',(-12.241454958378,-1.35873043767837,3.21878049181729));
#82498=CARTESIAN_POINT('Ctrl Pts',(-12.2855007421938,-1.44471385759508,
3.2137964656879));
#82499=CARTESIAN_POINT('Ctrl Pts',(-12.3334621233701,-1.52839065768477,
3.2088124395585));
#82500=CARTESIAN_POINT('Ctrl Pts',(-12.3814750244284,-1.61215734298556,
3.20382305961251));
#82501=CARTESIAN_POINT('Ctrl Pts',(-12.4334117012619,-1.69361208076667,
3.19883367966651));
#82502=CARTESIAN_POINT('Ctrl Pts',(-12.4890086318113,-1.77237823245545,
3.19384429972052));
#82503=CARTESIAN_POINT('Ctrl Pts',(-12.5446385173203,-1.85119107260919,
3.18885196233043));
#82504=CARTESIAN_POINT('Ctrl Pts',(-12.6039327071977,-1.92731180752927,
3.18385962494033));
#82505=CARTESIAN_POINT('Ctrl Pts',(-12.6665873291252,-2.00039684997779,
3.17886728755024));
#82506=CARTESIAN_POINT('Ctrl Pts',(-12.7293422469639,-2.07359888508704,
3.17386695855454));
#82507=CARTESIAN_POINT('Ctrl Pts',(-12.7954680370553,-2.14375520587752,
3.16886662955885));
#82508=CARTESIAN_POINT('Ctrl Pts',(-12.8646239972249,-2.2105591095404,3.16386630056315));
#82509=CARTESIAN_POINT('Ctrl Pts',(-12.9029769270648,-2.24760762168504,
3.16109318792502));
#82510=CARTESIAN_POINT('Ctrl Pts',(-12.942261233082,-2.28362575600063,3.15832007528689));
#82511=CARTESIAN_POINT('Ctrl Pts',(-12.9824147133364,-2.31856676872561,
3.15554696264875));
#82512=CARTESIAN_POINT('Ctrl Pts',(-13.0548252580608,-2.38157744049307,
3.15054608612606));
#82513=CARTESIAN_POINT('Ctrl Pts',(-13.1303167553614,-2.44130263322672,
3.14554520960336));
#82514=CARTESIAN_POINT('Ctrl Pts',(-13.2085587636618,-2.49742678506238,
3.14054433308066));
#82515=CARTESIAN_POINT('Ctrl Pts',(-13.2866951009647,-2.55347513752583,
3.13555021057184));
#82516=CARTESIAN_POINT('Ctrl Pts',(-13.3675742128677,-2.60593186153271,
3.13055608806303));
#82517=CARTESIAN_POINT('Ctrl Pts',(-13.4508312022446,-2.65452034952854,
3.12556196555422));
#82518=CARTESIAN_POINT('Ctrl Pts',(-13.534000809571,-2.70305784166514,3.12057308460733));
#82519=CARTESIAN_POINT('Ctrl Pts',(-13.6195429561016,-2.74773494882954,
3.11558420366044));
#82520=CARTESIAN_POINT('Ctrl Pts',(-13.7070631082673,-2.78831785203852,
3.11059532271355));
#82521=CARTESIAN_POINT('Ctrl Pts',(-13.7945211204159,-2.8288719410574,3.10560998391255));
#82522=CARTESIAN_POINT('Ctrl Pts',(-13.8839539494324,-2.86533742101005,
3.10062464511156));
#82523=CARTESIAN_POINT('Ctrl Pts',(-13.9749426223322,-2.89752646622749,
3.09563930631056));
#82524=CARTESIAN_POINT('Ctrl Pts',(-14.0658985060495,-2.92970391162219,
3.09065576405388));
#82525=CARTESIAN_POINT('Ctrl Pts',(-14.1584087064832,-2.95760783816921,
3.08567222179721));
#82526=CARTESIAN_POINT('Ctrl Pts',(-14.252035337805,-2.98109897757648,3.08068867954053));
#82527=CARTESIAN_POINT('Ctrl Pts',(-14.3456537475521,-3.00458805417153,
3.07570557490043));
#82528=CARTESIAN_POINT('Ctrl Pts',(-14.4403879677316,-3.0236650075225,3.07072247026032));
#82529=CARTESIAN_POINT('Ctrl Pts',(-14.5357870955796,-3.03824104201257,
3.06573936562021));
#82530=CARTESIAN_POINT('Ctrl Pts',(-14.631203847144,-3.05281976923058,3.06075534041799));
#82531=CARTESIAN_POINT('Ctrl Pts',(-14.7272853166938,-3.06289586001435,
3.05577131521577));
#82532=CARTESIAN_POINT('Ctrl Pts',(-14.8235736702086,-3.06843217297634,
3.05078729001355));
#82533=CARTESIAN_POINT('Ctrl Pts',(-14.9199654562741,-3.07397443302281,
3.04579791099209));
#82534=CARTESIAN_POINT('Ctrl Pts',(-15.0165641313095,-3.07496715457057,
3.04080853197063));
#82535=CARTESIAN_POINT('Ctrl Pts',(-15.1129102654888,-3.0714253241691,3.03581915294917));
#82536=CARTESIAN_POINT('Ctrl Pts',(-15.2093135086429,-3.06788139435487,
3.03082681648345));
#82537=CARTESIAN_POINT('Ctrl Pts',(-15.3054634759748,-3.05979759733429,
3.02583448001773));
#82538=CARTESIAN_POINT('Ctrl Pts',(-15.4009063801237,-3.04724077230142,
3.02084214355202));
#82539=CARTESIAN_POINT('Ctrl Pts',(-15.4965020670309,-3.03466384659808,
3.01584181547139));
#82540=CARTESIAN_POINT('Ctrl Pts',(-15.591387999395,-3.01759967345029,3.01084148739077));
#82541=CARTESIAN_POINT('Ctrl Pts',(-15.6851211660381,-2.99616608982991,
3.00584115931014));
#82542=CARTESIAN_POINT('Ctrl Pts',(-15.7371044526759,-2.98427928219375,
3.0030680375091));
#82543=CARTESIAN_POINT('Ctrl Pts',(-15.7887334530627,-2.97104947536094,
3.00029491570806));
#82544=CARTESIAN_POINT('Ctrl Pts',(-15.8399350346618,-2.95650323651907,
2.99752179390702));
#82545=CARTESIAN_POINT('Ctrl Pts',(-15.9322688027063,-2.93027144833599,
2.99252091742743));
#82546=CARTESIAN_POINT('Ctrl Pts',(-16.0235336132318,-2.89966427791211,
2.98752004094784));
#82547=CARTESIAN_POINT('Ctrl Pts',(-16.1132846394274,-2.86478612842476,
2.98251916446826));
#82548=CARTESIAN_POINT('Ctrl Pts',(-16.2029144508463,-2.82995508421613,
2.97752504200756));
#82549=CARTESIAN_POINT('Ctrl Pts',(-16.2910341358345,-2.79086468273055,
2.97253091954686));
#82550=CARTESIAN_POINT('Ctrl Pts',(-16.3772126745151,-2.74766946686733,
2.96753679708616));
#82551=CARTESIAN_POINT('Ctrl Pts',(-16.463300764759,-2.70451958641832,2.96254791619228));
#82552=CARTESIAN_POINT('Ctrl Pts',(-16.5474513687489,-2.65727365173485,
2.9575590352984));
#82553=CARTESIAN_POINT('Ctrl Pts',(-16.6292531176695,-2.60613440339599,
2.95257015440452));
#82554=CARTESIAN_POINT('Ctrl Pts',(-16.710996786568,-2.55503146441131,2.94758481566367));
#82555=CARTESIAN_POINT('Ctrl Pts',(-16.7903945448615,-2.50004093901466,
2.94259947692282));
#82556=CARTESIAN_POINT('Ctrl Pts',(-16.867060198074,-2.44141116298914,2.93761413818197));
#82557=CARTESIAN_POINT('Ctrl Pts',(-16.9436982235588,-2.3828025151666,2.93263059598983));
#82558=CARTESIAN_POINT('Ctrl Pts',(-17.0176057521235,-2.32055748873695,
2.9276470537977));
#82559=CARTESIAN_POINT('Ctrl Pts',(-17.0884269302826,-2.25496678620115,
2.92266351160556));
#82560=CARTESIAN_POINT('Ctrl Pts',(-17.159241889406,-2.18938184339621,2.91768040703432));
#82561=CARTESIAN_POINT('Ctrl Pts',(-17.2269707152862,-2.12045210685458,
2.91269730246307));
#82562=CARTESIAN_POINT('Ctrl Pts',(-17.2912927204202,-2.04850675355227,
2.90771419789183));
#82563=CARTESIAN_POINT('Ctrl Pts',(-17.3556266081319,-1.97654810936699,
2.90273017276274));
#82564=CARTESIAN_POINT('Ctrl Pts',(-17.4165521328222,-1.90157306906267,
2.89774614763365));
#82565=CARTESIAN_POINT('Ctrl Pts',(-17.4737880870322,-1.82394483207617,
2.89276212250455));
#82566=CARTESIAN_POINT('Ctrl Pts',(-17.5310855237983,-1.74623320725247,
2.88777274356231));
#82567=CARTESIAN_POINT('Ctrl Pts',(-17.5846852171434,-1.66586304967478,
2.88278336462006));
#82568=CARTESIAN_POINT('Ctrl Pts',(-17.6343487509913,-1.58322737095795,
2.87779398567782));
#82569=CARTESIAN_POINT('Ctrl Pts',(-17.6840417227628,-1.50054271016905,
2.87280164929488));
#82570=CARTESIAN_POINT('Ctrl Pts',(-17.7297936814228,-1.41559024033998,
2.86780931291195));
#82571=CARTESIAN_POINT('Ctrl Pts',(-17.7714127256809,-1.32878657200253,
2.86281697652901));
#82572=CARTESIAN_POINT('Ctrl Pts',(-17.8130983926879,-1.24184395047389,
2.85781664853598));
#82573=CARTESIAN_POINT('Ctrl Pts',(-17.850637764712,-1.15304461722821,2.85281632054295));
#82574=CARTESIAN_POINT('Ctrl Pts',(-17.8838875435545,-1.0628240146569,2.84781599254992));
#82575=CARTESIAN_POINT('Ctrl Pts',(-17.9023274756305,-1.01278874100421,
2.84504287008838));
#82576=CARTESIAN_POINT('Ctrl Pts',(-17.9194489584675,-0.962316593092614,
2.84226974762683));
#82577=CARTESIAN_POINT('Ctrl Pts',(-17.9352342955905,-0.911483340489207,
2.83949662516529));
#82578=CARTESIAN_POINT('Ctrl Pts',(-17.9696909433996,-0.800523183712012,
2.83344338073697));
#82579=CARTESIAN_POINT('Ctrl Pts',(-17.9978758533101,-0.687529803808016,
2.82739013630864));
#82580=CARTESIAN_POINT('Ctrl Pts',(-18.0195867091523,-0.57314776097502,
2.82133689188032));
#82581=CARTESIAN_POINT('Ctrl Pts',(-18.0410343069052,-0.460152673970379,
2.81535704693352));
#82582=CARTESIAN_POINT('Ctrl Pts',(-18.0561638683813,-0.345802413307247,
2.80937720198673));
#82583=CARTESIAN_POINT('Ctrl Pts',(-18.0648265530853,-0.230738920651397,
2.80339735703993));
#82584=CARTESIAN_POINT('Ctrl Pts',(-18.0705346107669,-0.154920733152448,
2.7994570889764));
#82585=CARTESIAN_POINT('Ctrl Pts',(-18.0734358049133,-0.0787932931042968,
2.79551682091286));
#82586=CARTESIAN_POINT('Ctrl Pts',(-18.0734989461686,-0.0025451719823722,
2.79157655284932));
#82587=CARTESIAN_POINT('Origin',(-15.,0.,8.20842344717746));
#82588=CARTESIAN_POINT('',(-13.1255958151414,2.44015351965519,4.43742368090164));
#82589=CARTESIAN_POINT('',(-13.1276888212995,2.43738653071546,4.35414767240703));
#82590=CARTESIAN_POINT('',(-13.1276888212995,2.43738653071547,8.20842344717746));
#82591=CARTESIAN_POINT('',(-18.073499953472,0.000534796702364866,3.70842344715139));
#82592=CARTESIAN_POINT('Ctrl Pts',(-13.1276888212995,2.43738653071546,4.35414767240703));
#82593=CARTESIAN_POINT('Ctrl Pts',(-13.0511512711489,2.37859318426367,4.34916457209983));
#82594=CARTESIAN_POINT('Ctrl Pts',(-12.9773717129505,2.31618058657907,4.34418147179263));
#82595=CARTESIAN_POINT('Ctrl Pts',(-12.9067013923136,2.25044510909689,4.33919837148543));
#82596=CARTESIAN_POINT('Ctrl Pts',(-12.8360235558487,2.18470264061002,4.33421474122274));
#82597=CARTESIAN_POINT('Ctrl Pts',(-12.7684559346109,2.11563688957496,4.32923111096004));
#82598=CARTESIAN_POINT('Ctrl Pts',(-12.7043138542653,2.04358199499847,4.32424748069735));
#82599=CARTESIAN_POINT('Ctrl Pts',(-12.6401056992207,1.9714528744934,4.31925871664622));
#82600=CARTESIAN_POINT('Ctrl Pts',(-12.5793304249195,1.8963287890356,4.3142699525951));
#82601=CARTESIAN_POINT('Ctrl Pts',(-12.5222637472399,1.81857782669818,4.30928118854398));
#82602=CARTESIAN_POINT('Ctrl Pts',(-12.4651672554918,1.74078624393895,4.30428981814955));
#82603=CARTESIAN_POINT('Ctrl Pts',(-12.4117834624104,1.66036541632739,4.29929844775512));
#82604=CARTESIAN_POINT('Ctrl Pts',(-12.3623441210296,1.5777115433858,4.29430707736069));
#82605=CARTESIAN_POINT('Ctrl Pts',(-12.3128213942626,1.49491826476197,4.28930728842071));
#82606=CARTESIAN_POINT('Ctrl Pts',(-12.2672566178983,1.40988480347299,4.28430749948072));
#82607=CARTESIAN_POINT('Ctrl Pts',(-12.2258351047685,1.32303113495693,4.27930771054073));
#82608=CARTESIAN_POINT('Ctrl Pts',(-12.1909618148304,1.24990794520622,4.27509832570277));
#82609=CARTESIAN_POINT('Ctrl Pts',(-12.1590245475239,1.17549506976768,4.27088894086482));
#82610=CARTESIAN_POINT('Ctrl Pts',(-12.1301065846113,1.10005183255543,4.26667955602686));
#82611=CARTESIAN_POINT('Ctrl Pts',(-12.0957512667359,1.01042323721447,4.2616786936008));
#82612=CARTESIAN_POINT('Ctrl Pts',(-12.0655387715763,0.919027325800495,
4.25667783117473));
#82613=CARTESIAN_POINT('Ctrl Pts',(-12.0396521966435,0.826282719873983,
4.25167696874867));
#82614=CARTESIAN_POINT('Ctrl Pts',(-12.0138005845027,0.733663376187409,
4.24668286056155));
#82615=CARTESIAN_POINT('Ctrl Pts',(-11.9922633974088,0.639699377256914,
4.24168875237442));
#82616=CARTESIAN_POINT('Ctrl Pts',(-11.9751753244573,0.5448283511603,4.2366946441873));
#82617=CARTESIAN_POINT('Ctrl Pts',(-11.9581051869753,0.450056900738318,
4.2317057777659));
#82618=CARTESIAN_POINT('Ctrl Pts',(-11.9454749576285,0.354380745180614,
4.22671691134449));
#82619=CARTESIAN_POINT('Ctrl Pts',(-11.9373689680756,0.258250677238143,
4.22172804492308));
#82620=CARTESIAN_POINT('Ctrl Pts',(-11.9292687342535,0.162188867314636,
4.21674272089113));
#82621=CARTESIAN_POINT('Ctrl Pts',(-11.92568639063,0.0656742216298454,4.21175739685917));
#82622=CARTESIAN_POINT('Ctrl Pts',(-11.9266546833621,-0.0308352833618727,
4.20677207282722));
#82623=CARTESIAN_POINT('Ctrl Pts',(-11.9276226271257,-0.12731000674011,
4.20178854548476));
#82624=CARTESIAN_POINT('Ctrl Pts',(-11.9331379441961,-0.223779154894447,
4.1968050181423));
#82625=CARTESIAN_POINT('Ctrl Pts',(-11.9431812820208,-0.319783638436798,
4.19182149079983));
#82626=CARTESIAN_POINT('Ctrl Pts',(-11.9532237376579,-0.415779689129582,
4.18683840120085));
#82627=CARTESIAN_POINT('Ctrl Pts',(-11.9677933774015,-0.511310720091047,
4.18185531160186));
#82628=CARTESIAN_POINT('Ctrl Pts',(-11.9868189728695,-0.605922724232127,
4.17687222200288));
#82629=CARTESIAN_POINT('Ctrl Pts',(-12.0058480826578,-0.700552204666182,
4.17188821195057));
#82630=CARTESIAN_POINT('Ctrl Pts',(-12.0293346963251,-0.794261891087647,
4.16690420189826));
#82631=CARTESIAN_POINT('Ctrl Pts',(-12.0571566868773,-0.8866089805598,4.16192019184595));
#82632=CARTESIAN_POINT('Ctrl Pts',(-12.0850085633729,-0.979055267818368,
4.15693082804869));
#82633=CARTESIAN_POINT('Ctrl Pts',(-12.1172049870273,-1.07013561539728,
4.15194146425142));
#82634=CARTESIAN_POINT('Ctrl Pts',(-12.1535743170824,-1.15942359887452,
4.14695210045415));
#82635=CARTESIAN_POINT('Ctrl Pts',(-12.1899652045813,-1.24876450663385,
4.14195977927687));
#82636=CARTESIAN_POINT('Ctrl Pts',(-12.2305337391959,-1.33631053705219,
4.1369674580996));
#82637=CARTESIAN_POINT('Ctrl Pts',(-12.2750615074182,-1.42165834912823,
4.13197513692233));
#82638=CARTESIAN_POINT('Ctrl Pts',(-12.3196605552928,-1.50714278521692,
4.12697482408206));
#82639=CARTESIAN_POINT('Ctrl Pts',(-12.3682312708503,-1.59042159816994,
4.12197451124179));
#82640=CARTESIAN_POINT('Ctrl Pts',(-12.4205110314977,-1.67111905960488,
4.11697419840152));
#82641=CARTESIAN_POINT('Ctrl Pts',(-12.4495063995669,-1.71587543506627,
4.11420092802939));
#82642=CARTESIAN_POINT('Ctrl Pts',(-12.4796419345662,-1.75983833668275,
4.11142765765726));
#82643=CARTESIAN_POINT('Ctrl Pts',(-12.5108675909139,-1.8029481689825,4.10865438728513));
#82644=CARTESIAN_POINT('Ctrl Pts',(-12.5671750600055,-1.88068570387152,
4.10365350486901));
#82645=CARTESIAN_POINT('Ctrl Pts',(-12.6272259494741,-1.95591853358483,
4.09865262245288));
#82646=CARTESIAN_POINT('Ctrl Pts',(-12.6907696301558,-2.02826461513016,
4.09365174003675));
#82647=CARTESIAN_POINT('Ctrl Pts',(-12.7542274917857,-2.10051298952278,
4.0886576115729));
#82648=CARTESIAN_POINT('Ctrl Pts',(-12.8211684822821,-2.16988203751743,
4.08366348310905));
#82649=CARTESIAN_POINT('Ctrl Pts',(-12.8912996089411,-2.23601988156365,
4.07866935464519));
#82650=CARTESIAN_POINT('Ctrl Pts',(-12.9613571305786,-2.30208831167549,
4.07368046769035));
#82651=CARTESIAN_POINT('Ctrl Pts',(-13.0345978148429,-2.36493198020902,
4.06869158073551));
#82652=CARTESIAN_POINT('Ctrl Pts',(-13.110690134037,-2.42423399868385,4.06370269378066));
#82653=CARTESIAN_POINT('Ctrl Pts',(-13.1867284279504,-2.48349391293289,
4.05871734891811));
#82654=CARTESIAN_POINT('Ctrl Pts',(-13.2656139867963,-2.53921690713262,
4.05373200405557));
#82655=CARTESIAN_POINT('Ctrl Pts',(-13.3469810867659,-2.59112537760918,
4.04874665919302));
#82656=CARTESIAN_POINT('Ctrl Pts',(-13.4283188653751,-2.64301514240534,
4.04376311084397));
#82657=CARTESIAN_POINT('Ctrl Pts',(-13.5121360388378,-2.69109287903848,
4.03877956249492));
#82658=CARTESIAN_POINT('Ctrl Pts',(-13.5980374918523,-2.7351240146926,4.03379601414586));
#82659=CARTESIAN_POINT('Ctrl Pts',(-13.683931402068,-2.77915128407923,4.02881290339013));
#82660=CARTESIAN_POINT('Ctrl Pts',(-13.7719088374825,-2.81913245905102,
4.0238297926344));
#82661=CARTESIAN_POINT('Ctrl Pts',(-13.8615506022402,-2.85487919512199,
4.01884668187867));
#82662=CARTESIAN_POINT('Ctrl Pts',(-13.9512089273806,-2.89063253503024,
4.01386265054512));
#82663=CARTESIAN_POINT('Ctrl Pts',(-14.0425317850346,-2.92214971997824,
4.00887861921156));
#82664=CARTESIAN_POINT('Ctrl Pts',(-14.1350815603233,-2.94929115936477,
4.00389458787801));
#82665=CARTESIAN_POINT('Ctrl Pts',(-14.2277307518254,-2.97646175386402,
3.99890520273866));
#82666=CARTESIAN_POINT('Ctrl Pts',(-14.3216090704307,-2.99924709549927,
3.99391581759931));
#82667=CARTESIAN_POINT('Ctrl Pts',(-14.4162655728082,-3.0175580141086,3.98892643245996));
#82668=CARTESIAN_POINT('Ctrl Pts',(-14.5109781825905,-3.03587978646911,
3.98393408987506));
#82669=CARTESIAN_POINT('Ctrl Pts',(-14.6064694607048,-3.0497217918892,3.97894174729016));
#82670=CARTESIAN_POINT('Ctrl Pts',(-14.7022822487487,-3.059046647338,3.97394940470526));
#82671=CARTESIAN_POINT('Ctrl Pts',(-14.7982484103532,-3.06838642966986,
3.96894907056335));
#82672=CARTESIAN_POINT('Ctrl Pts',(-14.894536671744,-3.07319460225313,3.96394873642144));
#82673=CARTESIAN_POINT('Ctrl Pts',(-14.9906888535839,-3.07348589594168,
3.95894840227953));
#82674=CARTESIAN_POINT('Ctrl Pts',(-15.0440124678769,-3.07364744019369,
3.95617534103415));
#82675=CARTESIAN_POINT('Ctrl Pts',(-15.0972942896739,-3.07242073009662,
3.95340227978877));
#82676=CARTESIAN_POINT('Ctrl Pts',(-15.1504570808492,-3.06981512746653,
3.95062921854339));
#82677=CARTESIAN_POINT('Ctrl Pts',(-15.2463296764332,-3.06511624161639,
3.94562834154971));
#82678=CARTESIAN_POINT('Ctrl Pts',(-15.3421491860804,-3.05591359807456,
3.94062746455604));
#82679=CARTESIAN_POINT('Ctrl Pts',(-15.4374586967929,-3.04220843115659,
3.93562658756236));
#82680=CARTESIAN_POINT('Ctrl Pts',(-15.5326394861444,-3.02852177391017,
3.93063246456089));
#82681=CARTESIAN_POINT('Ctrl Pts',(-15.6273112149682,-3.01034474089706,
3.92563834155943));
#82682=CARTESIAN_POINT('Ctrl Pts',(-15.7210190955906,-2.98773052897909,
3.92064421855796));
#82683=CARTESIAN_POINT('Ctrl Pts',(-15.8146286258718,-2.96514005162267,
3.91565533709753));
#82684=CARTESIAN_POINT('Ctrl Pts',(-15.9072758947998,-2.93812175576487,
3.9106664556371));
#82685=CARTESIAN_POINT('Ctrl Pts',(-15.9985143717709,-2.90678022894182,
3.90567757417667));
#82686=CARTESIAN_POINT('Ctrl Pts',(-16.0896880692237,-2.87546095467138,
3.900692234833));
#82687=CARTESIAN_POINT('Ctrl Pts',(-16.1794545494874,-2.83982469366955,
3.89570689548932));
#82688=CARTESIAN_POINT('Ctrl Pts',(-16.2673815073807,-2.80002613644041,
3.89072155614564));
#82689=CARTESIAN_POINT('Ctrl Pts',(-16.3552767797466,-2.76024192109577,
3.88573801332842));
#82690=CARTESIAN_POINT('Ctrl Pts',(-16.4413334476389,-2.71629857051968,
3.8807544705112));
#82691=CARTESIAN_POINT('Ctrl Pts',(-16.5251391936413,-2.66839890009331,
3.87577092769398));
#82692=CARTESIAN_POINT('Ctrl Pts',(-16.6089375807544,-2.62050343568367,
3.8707878224761));
#82693=CARTESIAN_POINT('Ctrl Pts',(-16.6904850582122,-2.56865256000697,
3.86580471725823));
#82694=CARTESIAN_POINT('Ctrl Pts',(-16.7693948757914,-2.51309451145853,
3.86082161204035));
#82695=CARTESIAN_POINT('Ctrl Pts',(-16.8483192711681,-2.45752619911783,
3.85583758624376));
#82696=CARTESIAN_POINT('Ctrl Pts',(-16.9246046802542,-2.39824960630894,
3.85085356044718));
#82697=CARTESIAN_POINT('Ctrl Pts',(-16.9978951281539,-2.33555503187123,
3.84586953465059));
#82698=CARTESIAN_POINT('Ctrl Pts',(-17.0712643046609,-2.27279311091465,
3.84088015501293));
#82699=CARTESIAN_POINT('Ctrl Pts',(-17.1416317634431,-2.20660616412503,
3.83589077537528));
#82700=CARTESIAN_POINT('Ctrl Pts',(-17.2086764816553,-2.13732319722186,
3.83090139573762));
#82701=CARTESIAN_POINT('Ctrl Pts',(-17.2757609406612,-2.06799916280183,
3.82590905864243));
#82702=CARTESIAN_POINT('Ctrl Pts',(-17.3395184476431,-1.99557578320459,
3.82091672154724));
#82703=CARTESIAN_POINT('Ctrl Pts',(-17.3996679623523,-1.92041555931523,
3.81592438445205));
#82704=CARTESIAN_POINT('Ctrl Pts',(-17.4599137631578,-1.84513502049751,
3.81092405572713));
#82705=CARTESIAN_POINT('Ctrl Pts',(-17.5165397820994,-1.76710924441421,
3.80592372700221));
#82706=CARTESIAN_POINT('Ctrl Pts',(-17.569308072578,-1.68673005492445,3.80092339827729));
#82707=CARTESIAN_POINT('Ctrl Pts',(-17.5985726683746,-1.64215281981712,
3.79815028211875));
#82708=CARTESIAN_POINT('Ctrl Pts',(-17.6266515660431,-1.59685221102482,
3.7953771659602));
#82709=CARTESIAN_POINT('Ctrl Pts',(-17.6535104129204,-1.55089804259443,
3.79260404980166));
#82710=CARTESIAN_POINT('Ctrl Pts',(-17.7037312761393,-1.46497261111064,
3.78741885745423));
#82711=CARTESIAN_POINT('Ctrl Pts',(-17.7498481749421,-1.37648008567004,
3.78223366510681));
#82712=CARTESIAN_POINT('Ctrl Pts',(-17.7916008762206,-1.28583311432093,
3.77704847275938));
#82713=CARTESIAN_POINT('Ctrl Pts',(-17.8332824144256,-1.19534064116923,
3.77187211802516));
#82714=CARTESIAN_POINT('Ctrl Pts',(-17.8706143949755,-1.1027013849238,3.76669576329094));
#82715=CARTESIAN_POINT('Ctrl Pts',(-17.9033815283408,-1.00835408011737,
3.76151940855672));
#82716=CARTESIAN_POINT('Ctrl Pts',(-17.9360830256386,-0.914195763038406,
3.75635342261384));
#82717=CARTESIAN_POINT('Ctrl Pts',(-17.9642377647595,-0.818336583660731,
3.75118743667097));
#82718=CARTESIAN_POINT('Ctrl Pts',(-17.98767825096,-0.721235688759529,3.74602145072809));
#82719=CARTESIAN_POINT('Ctrl Pts',(-18.0110906840712,-0.624251002202372,
3.74086164733042));
#82720=CARTESIAN_POINT('Ctrl Pts',(-18.0297999980823,-0.52602793756912,
3.73570184393275));
#82721=CARTESIAN_POINT('Ctrl Pts',(-18.0436881725886,-0.42704163502405,
3.73054204053508));
#82722=CARTESIAN_POINT('Ctrl Pts',(-18.0575581431002,-0.32818507927451,
3.72538900037574));
#82723=CARTESIAN_POINT('Ctrl Pts',(-18.0666195076493,-0.228567666925236,
3.72023596021641));
#82724=CARTESIAN_POINT('Ctrl Pts',(-18.0708052822106,-0.128674662414667,
3.71508292005708));
#82725=CARTESIAN_POINT('Ctrl Pts',(-18.07260842827,-0.0856427994216626,
3.71286309576387));
#82726=CARTESIAN_POINT('Ctrl Pts',(-18.0735074520523,-0.0425599117334144,
3.71064327147067));
#82727=CARTESIAN_POINT('Ctrl Pts',(-18.0734999534721,0.000534796196229549,
3.70842344717746));
#82728=CARTESIAN_POINT('Ctrl Pts',(-18.073499953472,0.000534796702359477,
3.70842344715139));
#82729=CARTESIAN_POINT('Ctrl Pts',(-18.0734820740241,0.10328876314218,3.70313055245769));
#82730=CARTESIAN_POINT('Ctrl Pts',(-18.0683069955294,0.205917074353121,
3.69783765776399));
#82731=CARTESIAN_POINT('Ctrl Pts',(-18.0580378511336,0.307907049341914,
3.69254476307029));
#82732=CARTESIAN_POINT('Ctrl Pts',(-18.0477346931935,0.410234836361457,
3.68723433720743));
#82733=CARTESIAN_POINT('Ctrl Pts',(-18.0323037584543,0.511919708943151,
3.68192391134456));
#82734=CARTESIAN_POINT('Ctrl Pts',(-18.0118597534527,0.612456590732762,
3.67661348548169));
#82735=CARTESIAN_POINT('Ctrl Pts',(-17.9913808082723,0.713165296811276,
3.67129398374407));
#82736=CARTESIAN_POINT('Ctrl Pts',(-17.9658717804935,0.812721758175001,
3.66597448200644));
#82737=CARTESIAN_POINT('Ctrl Pts',(-17.9354972645245,0.910636074383762,
3.66065498026882));
#82738=CARTESIAN_POINT('Ctrl Pts',(-17.9050354164564,1.00883191154829,3.655320184024));
#82739=CARTESIAN_POINT('Ctrl Pts',(-17.8696802228789,1.10537583161873,3.64998538777918));
#82740=CARTESIAN_POINT('Ctrl Pts',(-17.8296450073608,1.19979639202571,3.64465059153437));
#82741=CARTESIAN_POINT('Ctrl Pts',(-17.8044504744005,1.25921612763904,3.64129335470955));
#82742=CARTESIAN_POINT('Ctrl Pts',(-17.7774034483836,1.31779541931844,3.63793611788474));
#82743=CARTESIAN_POINT('Ctrl Pts',(-17.7485661821547,1.37542218693584,3.63457888105992));
#82744=CARTESIAN_POINT('Ctrl Pts',(-17.7056107277124,1.46126194620451,3.62957800364192));
#82745=CARTESIAN_POINT('Ctrl Pts',(-17.6585552263764,1.5452372290436,3.62457712622393));
#82746=CARTESIAN_POINT('Ctrl Pts',(-17.6075850331202,1.62693040571727,3.61957624880593));
#82747=CARTESIAN_POINT('Ctrl Pts',(-17.5566836783714,1.70851325052866,3.61458212539287));
#82748=CARTESIAN_POINT('Ctrl Pts',(-17.5018783698048,1.78781974580175,3.60958800197981));
#82749=CARTESIAN_POINT('Ctrl Pts',(-17.4434011571114,1.86445515779451,3.60459387856674));
#82750=CARTESIAN_POINT('Ctrl Pts',(-17.3849853188495,1.94101013751939,3.59960499670797));
#82751=CARTESIAN_POINT('Ctrl Pts',(-17.3229055025035,2.01489926020094,3.59461611484919));
#82752=CARTESIAN_POINT('Ctrl Pts',(-17.2574374568609,2.08575606875809,3.58962723299042));
#82753=CARTESIAN_POINT('Ctrl Pts',(-17.1920158939542,2.15656256852296,3.58464189327002));
#82754=CARTESIAN_POINT('Ctrl Pts',(-17.1232111810246,2.2243407129309,3.57965655354963));
#82755=CARTESIAN_POINT('Ctrl Pts',(-17.051339181143,2.28875726408626,3.57467121382924));
#82756=CARTESIAN_POINT('Ctrl Pts',(-16.9794930813869,2.35315060179599,3.56968767064887));
#82757=CARTESIAN_POINT('Ctrl Pts',(-16.904582217274,2.41418446075199,3.5647041274685));
#82758=CARTESIAN_POINT('Ctrl Pts',(-16.8269584326305,2.47156329788257,3.55972058428813));
#82759=CARTESIAN_POINT('Ctrl Pts',(-16.7493414642639,2.52893709647962,3.55473747872119));
#82760=CARTESIAN_POINT('Ctrl Pts',(-16.669012401906,2.58265625080491,3.54975437315425));
#82761=CARTESIAN_POINT('Ctrl Pts',(-16.5863543480257,2.63246692904201,3.54477126758731));
#82762=CARTESIAN_POINT('Ctrl Pts',(-16.5036810241425,2.68228680915558,3.53978724145627));
#82763=CARTESIAN_POINT('Ctrl Pts',(-16.4186782299777,2.72819655280745,3.53480321532523));
#82764=CARTESIAN_POINT('Ctrl Pts',(-16.3317551496124,2.76998744969738,3.52981918919419));
#82765=CARTESIAN_POINT('Ctrl Pts',(-16.2447386968974,2.81182323816522,3.52482980924656));
#82766=CARTESIAN_POINT('Ctrl Pts',(-16.1557982359609,2.84953115671571,3.51984042929892));
#82767=CARTESIAN_POINT('Ctrl Pts',(-16.0653642795656,2.88295008659979,3.51485104935129));
#82768=CARTESIAN_POINT('Ctrl Pts',(-15.9748767186394,2.91638882548182,3.50985871195955));
#82769=CARTESIAN_POINT('Ctrl Pts',(-15.8828943174917,2.9455333811086,3.50486637456781));
#82770=CARTESIAN_POINT('Ctrl Pts',(-15.7898621199645,2.970272728462,3.49987403717607));
#82771=CARTESIAN_POINT('Ctrl Pts',(-15.6966809988829,2.99505167792781,3.49487370817874));
#82772=CARTESIAN_POINT('Ctrl Pts',(-15.6024471544208,3.01541124633234,3.48987337918141));
#82773=CARTESIAN_POINT('Ctrl Pts',(-15.5076150891051,3.03129166714667,3.48487305018409));
#82774=CARTESIAN_POINT('Ctrl Pts',(-15.4550225502073,3.04009872672732,3.48209993756212));
#82775=CARTESIAN_POINT('Ctrl Pts',(-15.4022461111601,3.04752907982357,3.47932682494016));
#82776=CARTESIAN_POINT('Ctrl Pts',(-15.349363510309,3.05357943857117,3.47655371231819));
#82777=CARTESIAN_POINT('Ctrl Pts',(-15.252196107347,3.06469647209504,3.47145834735391));
#82778=CARTESIAN_POINT('Ctrl Pts',(-15.1543248192937,3.07119073472823,3.46636298238962));
#82779=CARTESIAN_POINT('Ctrl Pts',(-15.0562268722244,3.07298564735338,3.46126761742533));
#82780=CARTESIAN_POINT('Ctrl Pts',(-14.9600958654314,3.0747445705818,3.45627441849887));
#82781=CARTESIAN_POINT('Ctrl Pts',(-14.863747667448,3.07199079205801,3.45128121957241));
#82782=CARTESIAN_POINT('Ctrl Pts',(-14.7676395103559,3.06470404000979,3.44628802064595));
#82783=CARTESIAN_POINT('Ctrl Pts',(-14.6716232941742,3.05742425876029,3.44129959841347));
#82784=CARTESIAN_POINT('Ctrl Pts',(-14.5758470974853,3.04562015302896,3.43631117618099));
#82785=CARTESIAN_POINT('Ctrl Pts',(-14.4807683425551,3.029323478255,3.43132275394852));
#82786=CARTESIAN_POINT('Ctrl Pts',(-14.3857546256464,3.01303795111846,3.42633774401475));
#82787=CARTESIAN_POINT('Ctrl Pts',(-14.2914378332587,2.99226603700626,3.42135273408098));
#82788=CARTESIAN_POINT('Ctrl Pts',(-14.198269390584,2.96709121530254,3.41636772414722));
#82789=CARTESIAN_POINT('Ctrl Pts',(-14.1015457709371,2.94095575774583,3.41119249323289));
#82790=CARTESIAN_POINT('Ctrl Pts',(-14.006060382732,2.9100747143353,3.40601726231856));
#82791=CARTESIAN_POINT('Ctrl Pts',(-13.9123050577016,2.87459944383534,3.40084203140424));
#82792=CARTESIAN_POINT('Ctrl Pts',(-13.8220234257243,2.84043855415217,3.39585854601124));
#82793=CARTESIAN_POINT('Ctrl Pts',(-13.7333463505172,2.80201804783541,3.39087506061824));
#82794=CARTESIAN_POINT('Ctrl Pts',(-13.6466946169307,2.75952292799963,3.38589157522524));
#82795=CARTESIAN_POINT('Ctrl Pts',(-13.5600346086623,2.71702375015389,3.38090761394151));
#82796=CARTESIAN_POINT('Ctrl Pts',(-13.4754007165344,2.67044938602366,3.37592365265779));
#82797=CARTESIAN_POINT('Ctrl Pts',(-13.3931897327425,2.62003110955497,3.37093969137406));
#82798=CARTESIAN_POINT('Ctrl Pts',(-13.3109254881076,2.56958016932551,3.3659525012033));
#82799=CARTESIAN_POINT('Ctrl Pts',(-13.2310876511612,2.5152805872233,3.36096531103255));
#82800=CARTESIAN_POINT('Ctrl Pts',(-13.154044028865,2.45740692654494,3.35597812086179));
#82801=CARTESIAN_POINT('Ctrl Pts',(-13.1452221846569,2.45078012989336,3.35540706496629));
#82802=CARTESIAN_POINT('Ctrl Pts',(-13.1364369407639,2.44410651610121,3.35483600907079));
#82803=CARTESIAN_POINT('Ctrl Pts',(-13.1276888212995,2.43738653071547,3.3542649531753));
#82804=CARTESIAN_POINT('',(-18.0739720314691,0.000457053523349289,3.79157660465044));
#82805=CARTESIAN_POINT('Ctrl Pts',(-18.0734999658784,0.000457979655525854,
3.79157655282255));
#82806=CARTESIAN_POINT('Ctrl Pts',(-18.0734962197828,0.0255980150809229,
3.79026691442027));
#82807=CARTESIAN_POINT('Ctrl Pts',(-18.0731840258867,0.0507354218780576,
3.78895727601798));
#82808=CARTESIAN_POINT('Ctrl Pts',(-18.0725635426613,0.0758651850894085,
3.7876476376157));
#82809=CARTESIAN_POINT('Ctrl Pts',(-18.0701942141197,0.171823726401515,
3.78264675520893));
#82810=CARTESIAN_POINT('Ctrl Pts',(-18.0633211566005,0.267838563984851,
3.77764587280217));
#82811=CARTESIAN_POINT('Ctrl Pts',(-18.0519345090764,0.363452888705755,
3.77264499039541));
#82812=CARTESIAN_POINT('Ctrl Pts',(-18.0405632398134,0.458938081296764,
3.76765086194103));
#82813=CARTESIAN_POINT('Ctrl Pts',(-18.0246905473028,0.554023404166364,
3.76265673348665));
#82814=CARTESIAN_POINT('Ctrl Pts',(-18.0043585693512,0.648252911112749,
3.75766260503227));
#82815=CARTESIAN_POINT('Ctrl Pts',(-17.9840479305078,0.742383520959695,
3.752673718087));
#82816=CARTESIAN_POINT('Ctrl Pts',(-17.9592874023539,0.835659673953074,
3.74768483114172));
#82817=CARTESIAN_POINT('Ctrl Pts',(-17.9301706987204,0.927632430632183,
3.74269594419645));
#82818=CARTESIAN_POINT('Ctrl Pts',(-17.9010746678452,1.01953988697378,3.73771059934356));
#82819=CARTESIAN_POINT('Ctrl Pts',(-17.8676287420875,1.11014536966332,3.73272525449067));
#82820=CARTESIAN_POINT('Ctrl Pts',(-17.8299770689057,1.19901294382832,3.72773990963779));
#82821=CARTESIAN_POINT('Ctrl Pts',(-17.7923389638407,1.28784849376909,3.72275636129845));
#82822=CARTESIAN_POINT('Ctrl Pts',(-17.7504982936859,1.37494697604483,3.71777281295912));
#82823=CARTESIAN_POINT('Ctrl Pts',(-17.7046478019502,1.45989126903539,3.71278926461978));
#82824=CARTESIAN_POINT('Ctrl Pts',(-17.6588013362356,1.54482810327242,3.70780615387381));
#82825=CARTESIAN_POINT('Ctrl Pts',(-17.6089459575431,1.62761073838789,3.70282304312784));
#82826=CARTESIAN_POINT('Ctrl Pts',(-17.5553204398576,1.70784650939308,3.69783993238187));
#82827=CARTESIAN_POINT('Ctrl Pts',(-17.5016850154166,1.78809710312076,3.69285590105812));
#82828=CARTESIAN_POINT('Ctrl Pts',(-17.4442783125023,1.86579953361445,3.68787186973437));
#82829=CARTESIAN_POINT('Ctrl Pts',(-17.383381900477,1.94059088075737,3.68288783841062));
#82830=CARTESIAN_POINT('Ctrl Pts',(-17.3224200740224,2.01546256815557,3.67789845328106));
#82831=CARTESIAN_POINT('Ctrl Pts',(-17.2579613322987,2.08741658875113,3.6729090681515));
#82832=CARTESIAN_POINT('Ctrl Pts',(-17.190326788901,2.15612402422093,3.66791968302194));
#82833=CARTESIAN_POINT('Ctrl Pts',(-17.122652155297,2.22487218585111,3.66292734044684));
#82834=CARTESIAN_POINT('Ctrl Pts',(-17.0517982936774,2.29036963290002,3.65793499787174));
#82835=CARTESIAN_POINT('Ctrl Pts',(-16.9781207738701,2.35232660444579,3.65294265529663));
#82836=CARTESIAN_POINT('Ctrl Pts',(-16.9043253138179,2.41438275441689,3.64794232116444));
#82837=CARTESIAN_POINT('Ctrl Pts',(-16.8276975188581,2.47288684667339,3.64294198703224));
#82838=CARTESIAN_POINT('Ctrl Pts',(-16.7486233196402,2.5275914891474,3.63794165290004));
#82839=CARTESIAN_POINT('Ctrl Pts',(-16.7047707291522,2.55792932763249,3.63516859155802));
#82840=CARTESIAN_POINT('Ctrl Pts',(-16.6601662150027,2.58709942991981,3.63239553021599));
#82841=CARTESIAN_POINT('Ctrl Pts',(-16.6148787322104,2.6150657602161,3.62962246887397));
#82842=CARTESIAN_POINT('Ctrl Pts',(-16.5332082955066,2.66549961671397,3.62462159188003));
#82843=CARTESIAN_POINT('Ctrl Pts',(-16.4490304917344,2.71219184764961,3.6196207148861));
#82844=CARTESIAN_POINT('Ctrl Pts',(-16.3627225629527,2.75488465573779,3.61461983789216));
#82845=CARTESIAN_POINT('Ctrl Pts',(-16.2765311983419,2.79751980456053,3.60962571489045));
#82846=CARTESIAN_POINT('Ctrl Pts',(-16.1882158162888,2.83616607295716,3.60463159188875));
#82847=CARTESIAN_POINT('Ctrl Pts',(-16.0981813411113,2.87060968995003,3.59963746888704));
#82848=CARTESIAN_POINT('Ctrl Pts',(-16.0082413608828,2.90501715692566,3.59464858742639));
#82849=CARTESIAN_POINT('Ctrl Pts',(-15.9165862819263,2.93523058528095,3.58965970596574));
#82850=CARTESIAN_POINT('Ctrl Pts',(-15.8236433337036,2.96108323234008,3.58467082450508));
#82851=CARTESIAN_POINT('Ctrl Pts',(-15.7307663751782,2.98691752396303,3.57968548516122));
#82852=CARTESIAN_POINT('Ctrl Pts',(-15.6366037866106,3.00839707218904,3.57470014581736));
#82853=CARTESIAN_POINT('Ctrl Pts',(-15.5415994546647,3.02540448216546,3.5697148064735));
#82854=CARTESIAN_POINT('Ctrl Pts',(-15.4466293586627,3.04240576331889,3.56473126365612));
#82855=CARTESIAN_POINT('Ctrl Pts',(-15.3508185533612,3.05493803114046,3.55974772083874));
#82856=CARTESIAN_POINT('Ctrl Pts',(-15.2546217133959,3.06293487248217,3.55476417802136));
#82857=CARTESIAN_POINT('Ctrl Pts',(-15.1584333203684,3.07093101163011,3.54978107280335));
#82858=CARTESIAN_POINT('Ctrl Pts',(-15.0618593972539,3.07439247999359,3.54479796758533));
#82859=CARTESIAN_POINT('Ctrl Pts',(-14.9653592781951,3.0733047799385,3.53981486236732));
#82860=CARTESIAN_POINT('Ctrl Pts',(-14.8688413317076,3.07221687894174,3.53483083657062));
#82861=CARTESIAN_POINT('Ctrl Pts',(-14.7723976549859,3.06657814541914,3.52984681077392));
#82862=CARTESIAN_POINT('Ctrl Pts',(-14.6764860449469,3.05642617625322,3.52486278497722));
#82863=CARTESIAN_POINT('Ctrl Pts',(-14.580471406646,3.04626330184093,3.51987340533946));
#82864=CARTESIAN_POINT('Ctrl Pts',(-14.4849904129745,3.0315775594591,3.51488402570171));
#82865=CARTESIAN_POINT('Ctrl Pts',(-14.3904939819799,3.01245824269769,3.50989464606396));
#82866=CARTESIAN_POINT('Ctrl Pts',(-14.2959415381741,2.99332759295082,3.5049023089687));
#82867=CARTESIAN_POINT('Ctrl Pts',(-14.2023752442585,2.96975824309058,3.49990997187344));
#82868=CARTESIAN_POINT('Ctrl Pts',(-14.1102320415969,2.94188973794042,3.49491763477818));
#82869=CARTESIAN_POINT('Ctrl Pts',(-14.0179413380071,2.9139766214651,3.48991730605321));
#82870=CARTESIAN_POINT('Ctrl Pts',(-13.9270786873677,2.88175075492031,3.48491697732825));
#82871=CARTESIAN_POINT('Ctrl Pts',(-13.8380621272317,2.84540025828118,3.47991664860329));
#82872=CARTESIAN_POINT('Ctrl Pts',(-13.7886947206603,2.82524075375853,3.47714353244627));
#82873=CARTESIAN_POINT('Ctrl Pts',(-13.7398947013448,2.80381348694063,3.47437041628924));
#82874=CARTESIAN_POINT('Ctrl Pts',(-13.6917299249556,2.78115653294512,3.47159730013222));
#82875=CARTESIAN_POINT('Ctrl Pts',(-13.6048646115275,2.74029465092907,3.46659597712793));
#82876=CARTESIAN_POINT('Ctrl Pts',(-13.5197639714094,2.6952879144502,3.46159465412364));
#82877=CARTESIAN_POINT('Ctrl Pts',(-13.4368501248134,2.64631153073559,3.45659333111934));
#82878=CARTESIAN_POINT('Ctrl Pts',(-13.3540585553577,2.59740737491035,3.45159938381283));
#82879=CARTESIAN_POINT('Ctrl Pts',(-13.2734477413335,2.54454543399417,3.44660543650632));
#82880=CARTESIAN_POINT('Ctrl Pts',(-13.1954178916597,2.48794808311147,3.4416114891998));
#82881=CARTESIAN_POINT('Ctrl Pts',(-13.1726181386746,2.47141074996104,3.44015229421884));
#82882=CARTESIAN_POINT('Ctrl Pts',(-13.1500385872511,2.45455480341457,3.43869309923789));
#82883=CARTESIAN_POINT('Ctrl Pts',(-13.1276888212995,2.43738653071547,3.43723390425693));
#82884=CARTESIAN_POINT('Ctrl Pts',(-13.1255958151414,2.44015351965519,4.43742368090164));
#82885=CARTESIAN_POINT('Ctrl Pts',(-13.0351160055007,2.37176328111156,4.43153189146197));
#82886=CARTESIAN_POINT('Ctrl Pts',(-12.1759702308937,1.6408111827257,4.37296504577506));
#82887=CARTESIAN_POINT('Ctrl Pts',(-11.436582832353,-0.676361228608103,
4.26172314384091));
#82888=CARTESIAN_POINT('Ctrl Pts',(-13.6199704166047,-3.35423250130061,
4.10369797509917));
#82889=CARTESIAN_POINT('Ctrl Pts',(-17.0272186911122,-2.99125965920794,
3.94698262309378));
#82890=CARTESIAN_POINT('Ctrl Pts',(-18.0762959775521,-0.987130875700585,
3.84294232733563));
#82891=CARTESIAN_POINT('Ctrl Pts',(-18.0783729425329,0.000448419499977877,
3.79157708782474));
#82892=CARTESIAN_POINT('Origin',(-15.,0.,8.20842344717746));
#82893=CARTESIAN_POINT('',(-13.1276888212995,2.43738653071547,5.43736138633702));
#82894=CARTESIAN_POINT('',(-13.1256826865589,2.43995710119903,5.35407232013781));
#82895=CARTESIAN_POINT('',(-13.1276888212995,2.43738653071547,8.20842344717746));
#82896=CARTESIAN_POINT('',(-18.0730476819807,-0.00351971310571451,5.79157674198311));
#82897=CARTESIAN_POINT('Ctrl Pts',(-18.0734979882452,-0.00351656827781883,
5.79157655282255));
#82898=CARTESIAN_POINT('Ctrl Pts',(-18.0736072822651,0.0920069431531279,
5.78664473933955));
#82899=CARTESIAN_POINT('Ctrl Pts',(-18.0692590445082,0.187606130278477,
5.78171292585655));
#82900=CARTESIAN_POINT('Ctrl Pts',(-18.0604590887115,0.282829305984153,
5.77678111237354));
#82901=CARTESIAN_POINT('Ctrl Pts',(-18.0516617025475,0.378024676028252,
5.77185073900568));
#82902=CARTESIAN_POINT('Ctrl Pts',(-18.038415221166,0.472843806578188,5.76692036563781));
#82903=CARTESIAN_POINT('Ctrl Pts',(-18.0207774649557,0.566838387210871,
5.76198999226995));
#82904=CARTESIAN_POINT('Ctrl Pts',(-18.0031398133705,0.660832410278753,
5.75705964814848));
#82905=CARTESIAN_POINT('Ctrl Pts',(-17.9811110222353,0.754001452603219,
5.75212930402701));
#82906=CARTESIAN_POINT('Ctrl Pts',(-17.9548001333951,0.845906863483294,
5.74719895990554));
#82907=CARTESIAN_POINT('Ctrl Pts',(-17.9284818733408,0.937838022427872,
5.7422672345072));
#82908=CARTESIAN_POINT('Ctrl Pts',(-17.8978792574336,1.02850441626493,5.73733550910886));
#82909=CARTESIAN_POINT('Ctrl Pts',(-17.8631509863536,1.11748318973598,5.73240378371051));
#82910=CARTESIAN_POINT('Ctrl Pts',(-17.8283818661184,1.20656662455667,5.72746625736644));
#82911=CARTESIAN_POINT('Ctrl Pts',(-17.7894775723116,1.29395806073367,5.72252873102237));
#82912=CARTESIAN_POINT('Ctrl Pts',(-17.7466445403766,1.37925560314957,5.71759120467829));
#82913=CARTESIAN_POINT('Ctrl Pts',(-17.7037815187446,1.46461286693794,5.71265022130789));
#82914=CARTESIAN_POINT('Ctrl Pts',(-17.6569845067983,1.54787293116407,5.70770923793749));
#82915=CARTESIAN_POINT('Ctrl Pts',(-17.6065042419745,1.62866137873061,5.70276825456709));
#82916=CARTESIAN_POINT('Ctrl Pts',(-17.5559431874896,1.70957912180153,5.69781936354458));
#82917=CARTESIAN_POINT('Ctrl Pts',(-17.5016873762857,1.78801699128002,5.69287047252208));
#82918=CARTESIAN_POINT('Ctrl Pts',(-17.4440286458054,1.8636325357974,5.68792158149958));
#82919=CARTESIAN_POINT('Ctrl Pts',(-17.4286032501567,1.88386190404153,5.68659760850523));
#82920=CARTESIAN_POINT('Ctrl Pts',(-17.4129345076039,1.90388947532135,5.68527363551087));
#82921=CARTESIAN_POINT('Ctrl Pts',(-17.3970284450544,1.92370914735055,5.68394966251652));
#82922=CARTESIAN_POINT('Ctrl Pts',(-17.3368771896634,1.99866032714632,5.67894285222227));
#82923=CARTESIAN_POINT('Ctrl Pts',(-17.2731035294659,2.07091670579144,5.67393604192802));
#82924=CARTESIAN_POINT('Ctrl Pts',(-17.2059776324753,2.14010862692026,5.66892923163378));
#82925=CARTESIAN_POINT('Ctrl Pts',(-17.1389423799006,2.209207113748,5.66392918235747));
#82926=CARTESIAN_POINT('Ctrl Pts',(-17.0685641899493,2.27524905664967,5.65892913308117));
#82927=CARTESIAN_POINT('Ctrl Pts',(-16.9951540132018,2.33789707078918,5.65392908380487));
#82928=CARTESIAN_POINT('Ctrl Pts',(-16.9218210229,2.40047921425854,5.64893429178374));
#82929=CARTESIAN_POINT('Ctrl Pts',(-16.8454627148059,2.45967424103802,5.64393949976261));
#82930=CARTESIAN_POINT('Ctrl Pts',(-16.7664267653277,2.51518165004718,5.63894470774148));
#82931=CARTESIAN_POINT('Ctrl Pts',(-16.6874476518167,2.57064914282447,5.63395350755215));
#82932=CARTESIAN_POINT('Ctrl Pts',(-16.6057950822321,2.62243403946385,5.62896230736282));
#82933=CARTESIAN_POINT('Ctrl Pts',(-16.5218489159773,2.67027678845072,5.62397110717348));
#82934=CARTESIAN_POINT('Ctrl Pts',(-16.4379335277937,2.71810199634431,5.61898173696069));
#82935=CARTESIAN_POINT('Ctrl Pts',(-16.3517265936208,2.76198771227858,5.61399236674789));
#82936=CARTESIAN_POINT('Ctrl Pts',(-16.2636351889554,2.80171882230064,5.60900299653509));
#82937=CARTESIAN_POINT('Ctrl Pts',(-16.1755522383816,2.84144611934632,5.60401410514986));
#82938=CARTESIAN_POINT('Ctrl Pts',(-16.0855855757646,2.87701942363017,5.59902521376464));
#82939=CARTESIAN_POINT('Ctrl Pts',(-15.9941640445155,2.90827098163024,5.59403632237941));
#82940=CARTESIAN_POINT('Ctrl Pts',(-15.9027265423428,2.93952799913467,5.58904655945765));
#82941=CARTESIAN_POINT('Ctrl Pts',(-15.8098340807032,2.9664616294552,5.5840567965359));
#82942=CARTESIAN_POINT('Ctrl Pts',(-15.7159315074474,2.98895371771529,5.57906703361414));
#82943=CARTESIAN_POINT('Ctrl Pts',(-15.6219302684125,3.01146943897431,5.57407202782385));
#82944=CARTESIAN_POINT('Ctrl Pts',(-15.5269172249754,3.02953419920992,5.56907702203356));
#82945=CARTESIAN_POINT('Ctrl Pts',(-15.4313480654783,3.04308085604181,5.56408201624327));
#82946=CARTESIAN_POINT('Ctrl Pts',(-15.3357233712283,3.05663538476712,5.55908410788051));
#82947=CARTESIAN_POINT('Ctrl Pts',(-15.2395423527312,3.06566654080875,5.55408619951775));
#82948=CARTESIAN_POINT('Ctrl Pts',(-15.1432644002756,3.070159207861,5.54908829115498));
#82949=CARTESIAN_POINT('Ctrl Pts',(-15.0468352254713,3.0746589314786,5.54408253265185));
#82950=CARTESIAN_POINT('Ctrl Pts',(-14.9503092498453,3.07460593233485,5.53907677414872));
#82951=CARTESIAN_POINT('Ctrl Pts',(-14.8541443578981,3.07003719548592,5.53407101564558));
#82952=CARTESIAN_POINT('Ctrl Pts',(-14.8019771458789,3.06755876225491,5.53135550835532));
#82953=CARTESIAN_POINT('Ctrl Pts',(-14.7499160909764,3.06375233419271,5.52864000106506));
#82954=CARTESIAN_POINT('Ctrl Pts',(-14.6980331473027,3.05863012962864,5.5259244937748));
#82955=CARTESIAN_POINT('Ctrl Pts',(-14.6023361309739,3.04918232927076,5.52091579675229));
#82956=CARTESIAN_POINT('Ctrl Pts',(-14.5069222957617,3.03522319463142,5.51590709972977));
#82957=CARTESIAN_POINT('Ctrl Pts',(-14.4122491793749,3.01677828533264,5.51089840270726));
#82958=CARTESIAN_POINT('Ctrl Pts',(-14.3176949370156,2.99835653594174,5.50589599473501));
#82959=CARTESIAN_POINT('Ctrl Pts',(-14.2238799907018,2.9754602871356,5.50089358676275));
#82960=CARTESIAN_POINT('Ctrl Pts',(-14.1312570510269,2.94816687767323,5.4958911787905));
#82961=CARTESIAN_POINT('Ctrl Pts',(-14.0387345507126,2.92090306490263,5.49089419537786));
#82962=CARTESIAN_POINT('Ctrl Pts',(-13.9474019031945,2.88925169788506,5.48589721196523));
#82963=CARTESIAN_POINT('Ctrl Pts',(-13.8577007516974,2.85334096759,5.4809002285526));
#82964=CARTESIAN_POINT('Ctrl Pts',(-13.7680578858049,2.81745357120527,5.47590649205702));
#82965=CARTESIAN_POINT('Ctrl Pts',(-13.6800448133697,2.77731247431519,5.47091275556145));
#82966=CARTESIAN_POINT('Ctrl Pts',(-13.5940863736698,2.73309515481974,5.46591901906588));
#82967=CARTESIAN_POINT('Ctrl Pts',(-13.5081446764819,2.68888644773051,5.46092625522282));
#82968=CARTESIAN_POINT('Ctrl Pts',(-13.4242572092542,2.64060328715728,5.45593349137977));
#82969=CARTESIAN_POINT('Ctrl Pts',(-13.342826504894,2.58847025424634,5.45094072753672));
#82970=CARTESIAN_POINT('Ctrl Pts',(-13.269001308176,2.54120636969085,5.44641428047015));
#82971=CARTESIAN_POINT('Ctrl Pts',(-13.1971953162039,2.49077887770757,5.44188783340359));
#82972=CARTESIAN_POINT('Ctrl Pts',(-13.1276888212995,2.43738653071547,5.43736138633702));
#82973=CARTESIAN_POINT('',(-15.7937992825329,-2.96922295374568,6.));
#82974=CARTESIAN_POINT('Ctrl Pts',(-15.7937992825329,-2.96922295374568,
6.));
#82975=CARTESIAN_POINT('Ctrl Pts',(-16.7765145099755,-2.70650147589437,
5.94732494375275));
#82976=CARTESIAN_POINT('Ctrl Pts',(-17.8761971489951,-1.66915693147179,
5.87785090484933));
#82977=CARTESIAN_POINT('Ctrl Pts',(-18.0726938053019,-0.328583276450114,
5.80837686594592));
#82978=CARTESIAN_POINT('Ctrl Pts',(-18.0703307438941,-0.00353868753125157,
5.79157788328974));
#82979=CARTESIAN_POINT('',(-14.2057854622994,-2.96911190730578,5.99999996471849));
#82980=CARTESIAN_POINT('Origin',(-15.,0.,6.));
#82981=CARTESIAN_POINT('',(-18.0736575411657,0.00192524165061634,5.70842344717746));
#82982=CARTESIAN_POINT('Ctrl Pts',(-14.2057854622994,-2.96911190730578,
5.99999996471849));
#82983=CARTESIAN_POINT('Ctrl Pts',(-14.2981329538255,-2.99381414911409,
5.99502017228295));
#82984=CARTESIAN_POINT('Ctrl Pts',(-14.3918009260944,-3.0142484885268,5.99004037984741));
#82985=CARTESIAN_POINT('Ctrl Pts',(-14.4863574076049,-3.03027614868309,
5.98506058741186));
#82986=CARTESIAN_POINT('Ctrl Pts',(-14.5807866776791,-3.04628224604818,
5.98008749453343));
#82987=CARTESIAN_POINT('Ctrl Pts',(-14.6761016489036,-3.05789337130818,
5.975114401655));
#82988=CARTESIAN_POINT('Ctrl Pts',(-14.7718563427238,-3.06502083543402,
5.97014130877657));
#82989=CARTESIAN_POINT('Ctrl Pts',(-14.8707044704539,-3.0723785581335,5.96500755605439));
#82990=CARTESIAN_POINT('Ctrl Pts',(-14.9700207596084,-3.07495783903088,
5.95987380333221));
#82991=CARTESIAN_POINT('Ctrl Pts',(-15.0693042032246,-3.07271853208448,
5.95474005061003));
#82992=CARTESIAN_POINT('Ctrl Pts',(-15.1653131834789,-3.0705530796327,5.94977561398513));
#82993=CARTESIAN_POINT('Ctrl Pts',(-15.2612909701088,-3.06388190765667,
5.94481117736023));
#82994=CARTESIAN_POINT('Ctrl Pts',(-15.3567818694496,-3.05272156405265,
5.93984674073533));
#82995=CARTESIAN_POINT('Ctrl Pts',(-15.4522414511916,-3.04156488064207,
5.93488393226804));
#82996=CARTESIAN_POINT('Ctrl Pts',(-15.5472140234408,-3.02592200199951,
5.92992112380074));
#82997=CARTESIAN_POINT('Ctrl Pts',(-15.6412484396551,-3.00586138879355,
5.92495831533345));
#82998=CARTESIAN_POINT('Ctrl Pts',(-15.7352782205293,-2.98580176445709,
5.91999575150324));
#82999=CARTESIAN_POINT('Ctrl Pts',(-15.8283695043764,-2.96132493159438,
5.91503318767304));
#83000=CARTESIAN_POINT('Ctrl Pts',(-15.9200818807813,-2.93255035466708,
5.91007062384283));
#83001=CARTESIAN_POINT('Ctrl Pts',(-16.0118152939033,-2.90376917751133,
5.90510692171422));
#83002=CARTESIAN_POINT('Ctrl Pts',(-16.1021687491958,-2.87068843159189,
5.90014321958561));
#83003=CARTESIAN_POINT('Ctrl Pts',(-16.1907186020685,-2.8334769207968,5.895179517457));
#83004=CARTESIAN_POINT('Ctrl Pts',(-16.279363489585,-2.79622547337207,5.89021048811835));
#83005=CARTESIAN_POINT('Ctrl Pts',(-16.3662005037129,-2.75483458692342,
5.88524145877971));
#83006=CARTESIAN_POINT('Ctrl Pts',(-16.4508278702327,-2.70952038947046,
5.88027242944107));
#83007=CARTESIAN_POINT('Ctrl Pts',(-16.5355097997349,-2.6641769759629,5.87530019635083));
#83008=CARTESIAN_POINT('Ctrl Pts',(-16.6179788668853,-2.61490544397536,
5.87032796326059));
#83009=CARTESIAN_POINT('Ctrl Pts',(-16.6978614993426,-2.56196576461322,
5.86535573017034));
#83010=CARTESIAN_POINT('Ctrl Pts',(-16.777862735832,-2.50894748419303,5.86037611466324));
#83011=CARTESIAN_POINT('Ctrl Pts',(-16.8552695203958,-2.45225045177839,
5.85539649915613));
#83012=CARTESIAN_POINT('Ctrl Pts',(-16.929740909553,-2.39217521766225,5.85041688364903));
#83013=CARTESIAN_POINT('Ctrl Pts',(-16.9471171151244,-2.37815802757672,
5.84925500358076));
#83014=CARTESIAN_POINT('Ctrl Pts',(-16.9643336718353,-2.36395708041279,
5.84809312351249));
#83015=CARTESIAN_POINT('Ctrl Pts',(-16.9813865454886,-2.34957647403879,
5.84693124344423));
#83016=CARTESIAN_POINT('Ctrl Pts',(-17.0538726013641,-2.28844933157971,
5.84199248032074));
#83017=CARTESIAN_POINT('Ctrl Pts',(-17.1236662966299,-2.22384719863751,
5.83705371719726));
#83018=CARTESIAN_POINT('Ctrl Pts',(-17.1904101659715,-2.15603932125758,
5.83211495407377));
#83019=CARTESIAN_POINT('Ctrl Pts',(-17.2600602784974,-2.08527887035407,
5.82696114128643));
#83020=CARTESIAN_POINT('Ctrl Pts',(-17.3263884968989,-2.01102738546575,
5.82180732849908));
#83021=CARTESIAN_POINT('Ctrl Pts',(-17.3890253810344,-1.93363905079863,
5.81665351571173));
#83022=CARTESIAN_POINT('Ctrl Pts',(-17.4489019566701,-1.85966109774477,
5.81172682330944));
#83023=CARTESIAN_POINT('Ctrl Pts',(-17.5054053086427,-1.78281729323004,
5.80680013090714));
#83024=CARTESIAN_POINT('Ctrl Pts',(-17.5582502566199,-1.70345468812772,
5.80187343850485));
#83025=CARTESIAN_POINT('Ctrl Pts',(-17.6110650497904,-1.62413736954947,
5.79694955741115));
#83026=CARTESIAN_POINT('Ctrl Pts',(-17.660225334983,-1.54230447853674,5.79202567631746));
#83027=CARTESIAN_POINT('Ctrl Pts',(-17.7054876831221,-1.45833420260055,
5.78710179522376));
#83028=CARTESIAN_POINT('Ctrl Pts',(-17.750737289915,-1.37438756428807,5.78217930020206));
#83029=CARTESIAN_POINT('Ctrl Pts',(-17.7920909261204,-1.28830513300759,
5.77725680518037));
#83030=CARTESIAN_POINT('Ctrl Pts',(-17.8293504193898,-1.20049092220581,
5.77233431015867));
#83031=CARTESIAN_POINT('Ctrl Pts',(-17.866610196384,-1.11267604271373,5.76741177765302));
#83032=CARTESIAN_POINT('Ctrl Pts',(-17.8997755947692,-1.02312977334097,
5.76248924514736));
#83033=CARTESIAN_POINT('Ctrl Pts',(-17.9286965110889,-0.932276244433962,
5.7575667126417));
#83034=CARTESIAN_POINT('Ctrl Pts',(-17.9576404750251,-0.841350312658586,
5.75264025727826));
#83035=CARTESIAN_POINT('Ctrl Pts',(-17.9823330691332,-0.749115472153399,
5.74771380191482));
#83036=CARTESIAN_POINT('Ctrl Pts',(-18.0026741953112,-0.656010614862657,
5.74278734655138));
#83037=CARTESIAN_POINT('Ctrl Pts',(-18.0230248956179,-0.562861935125983,
5.73785857241177));
#83038=CARTESIAN_POINT('Ctrl Pts',(-18.0390199757596,-0.468842867573405,
5.73292979827217));
#83039=CARTESIAN_POINT('Ctrl Pts',(-18.0506108997062,-0.374400038186194,
5.72800102413256));
#83040=CARTESIAN_POINT('Ctrl Pts',(-18.0622170327952,-0.279833284731336,
5.72306578265453));
#83041=CARTESIAN_POINT('Ctrl Pts',(-18.0694074453535,-0.184842108475051,
5.71813054117649));
#83042=CARTESIAN_POINT('Ctrl Pts',(-18.0721856531716,-0.08987526047971,
5.71319529969846));
#83043=CARTESIAN_POINT('Ctrl Pts',(-18.0730810634597,-0.0592676536020603,
5.71160468219146));
#83044=CARTESIAN_POINT('Ctrl Pts',(-18.0735185562359,-0.0286625483501631,
5.71001406468446));
#83045=CARTESIAN_POINT('Ctrl Pts',(-18.0734993970759,0.00192514259417154,
5.70842344717746));
#83046=CARTESIAN_POINT('Ctrl Pts',(-18.0766836350382,0.00192713709989245,
5.70842344717746));
#83047=CARTESIAN_POINT('Ctrl Pts',(-18.0776349419369,0.127164229732423,
5.70191765635247));
#83048=CARTESIAN_POINT('Ctrl Pts',(-18.0140094212094,1.26546671125655,5.64273680928023));
#83049=CARTESIAN_POINT('Ctrl Pts',(-16.5948036893957,3.25791148079165,5.53088090596076));
#83050=CARTESIAN_POINT('Ctrl Pts',(-14.156529652945,3.15709983619958,5.41926965443919));
#83051=CARTESIAN_POINT('Ctrl Pts',(-13.2206851146332,2.51416173457833,5.36033345916488));
#83052=CARTESIAN_POINT('Ctrl Pts',(-13.1256826865589,2.43995710119902,5.35407232013781));
#83053=CARTESIAN_POINT('Origin',(-15.,0.,3.));
#83054=CARTESIAN_POINT('',(-17.3614291533995,0.872615954171733,0.32975881722873));
#83055=CARTESIAN_POINT('',(-17.3614291890562,0.872615857679407,0.0533213468502638));
#83056=CARTESIAN_POINT('',(-17.3614291890287,0.872615857753799,3.));
#83057=CARTESIAN_POINT('',(-16.913465996665,1.63598720337497,0.));
#83058=CARTESIAN_POINT('Ctrl Pts',(-17.3614291890837,0.872615857605008,
0.0533213468502644));
#83059=CARTESIAN_POINT('Ctrl Pts',(-17.3052161900689,1.02473665110477,0.0434939346638048));
#83060=CARTESIAN_POINT('Ctrl Pts',(-17.2344350464082,1.17107267661228,0.0340532122102998));
#83061=CARTESIAN_POINT('Ctrl Pts',(-17.1011568765138,1.38988700371282,0.0189269413933175));
#83062=CARTESIAN_POINT('Ctrl Pts',(-17.0477914117863,1.46737654487933,0.0133363778978164));
#83063=CARTESIAN_POINT('Ctrl Pts',(-16.9764158275753,1.55951755727942,0.00618525948857481));
#83064=CARTESIAN_POINT('Ctrl Pts',(-16.9623709791679,1.57715396022876,0.00479206767144312));
#83065=CARTESIAN_POINT('Ctrl Pts',(-16.9366976029821,1.60851864428275,0.00226581726433723));
#83066=CARTESIAN_POINT('Ctrl Pts',(-16.9251550674062,1.62231555646376,0.00113715644275298));
#83067=CARTESIAN_POINT('Ctrl Pts',(-16.9134659966651,1.63598720337494,-1.35308431126191E-14));
#83068=CARTESIAN_POINT('',(-13.1119440673944,1.66524804319138,0.));
#83069=CARTESIAN_POINT('Origin',(-15.,0.,0.));
#83070=CARTESIAN_POINT('Ctrl Pts',(-13.1119440673944,1.66524804319138,2.16064552317416E-15));
#83071=CARTESIAN_POINT('Ctrl Pts',(-13.1135335123553,1.66705015369397,0.000157689880063195));
#83072=CARTESIAN_POINT('Ctrl Pts',(-13.1151255349311,1.66884998572192,0.000315530651660374));
#83073=CARTESIAN_POINT('Ctrl Pts',(-13.1324724607268,1.68840474846791,0.00203422419148989));
#83074=CARTESIAN_POINT('Ctrl Pts',(-13.1484745908993,1.7059376549406,0.00360924412967116));
#83075=CARTESIAN_POINT('Ctrl Pts',(-13.2534887681128,1.81777937908589,0.0138647376047754));
#83076=CARTESIAN_POINT('Ctrl Pts',(-13.3494226709774,1.90531206599647,0.0228556276482404));
#83077=CARTESIAN_POINT('Ctrl Pts',(-13.5355877911107,2.05051970210863,0.0391499519066325));
#83078=CARTESIAN_POINT('Ctrl Pts',(-13.623582970446,2.11059555403921,0.0464530866945166));
#83079=CARTESIAN_POINT('Ctrl Pts',(-13.7788341957787,2.202736759696,0.0585670985125662));
#83080=CARTESIAN_POINT('Ctrl Pts',(-13.8441880865476,2.23772110470361,0.0634565361499455));
#83081=CARTESIAN_POINT('Ctrl Pts',(-13.9474036428933,2.28724240695303,0.0708607840807191));
#83082=CARTESIAN_POINT('Ctrl Pts',(-13.9842281774554,2.30383263886003,0.0734430106906672));
#83083=CARTESIAN_POINT('Ctrl Pts',(-14.0552558746739,2.33379776538124,0.0783160517901265));
#83084=CARTESIAN_POINT('Ctrl Pts',(-14.0893833186159,2.34732421127126,0.0806113988119353));
#83085=CARTESIAN_POINT('Ctrl Pts',(-14.1714383348913,2.37778772791051,0.0860287056502805));
#83086=CARTESIAN_POINT('Ctrl Pts',(-14.2196076831033,2.39402950428948,0.0891277408921832));
#83087=CARTESIAN_POINT('Ctrl Pts',(-14.405553329791,2.45051727712314,0.100829173395792));
#83088=CARTESIAN_POINT('Ctrl Pts',(-14.5461873762118,2.48041537783897,0.109121425604108));
#83089=CARTESIAN_POINT('Ctrl Pts',(-14.7850155934075,2.51018443359966,0.123024089519485));
#83090=CARTESIAN_POINT('Ctrl Pts',(-14.882028683596,2.51660984285428,0.128629015144472));
#83091=CARTESIAN_POINT('Ctrl Pts',(-15.0364294410421,2.51788772643851,0.137783619794858));
#83092=CARTESIAN_POINT('Ctrl Pts',(-15.0936893712441,2.51640756498048,0.141230510496763));
#83093=CARTESIAN_POINT('Ctrl Pts',(-15.1761668073964,2.51145675548247,0.146332446298021));
#83094=CARTESIAN_POINT('Ctrl Pts',(-15.2014635092165,2.50955416643222,0.147915963725465));
#83095=CARTESIAN_POINT('Ctrl Pts',(-15.247739526031,2.50536954522139,0.150854040337095));
#83096=CARTESIAN_POINT('Ctrl Pts',(-15.2687261830582,2.50320545547813,0.152202679230776));
#83097=CARTESIAN_POINT('Ctrl Pts',(-15.321716423073,2.49706722557264,0.155647203925214));
#83098=CARTESIAN_POINT('Ctrl Pts',(-15.3536742692965,2.49274155642832,0.157760245281535));
#83099=CARTESIAN_POINT('Ctrl Pts',(-15.5316576101007,2.46515922978768,0.169696690307591));
#83100=CARTESIAN_POINT('Ctrl Pts',(-15.6754877712572,2.42968734194731,0.179959744111941));
#83101=CARTESIAN_POINT('Ctrl Pts',(-15.9109727885108,2.34907369416207,0.197107441612617));
#83102=CARTESIAN_POINT('Ctrl Pts',(-16.0045310908566,2.31061438230456,0.204022654996152));
#83103=CARTESIAN_POINT('Ctrl Pts',(-16.1599282872409,2.23550632759541,0.215582544968285));
#83104=CARTESIAN_POINT('Ctrl Pts',(-16.2229752173846,2.20164833410109,0.220296203449823));
#83105=CARTESIAN_POINT('Ctrl Pts',(-16.3186507052275,2.14488772362933,0.227485132641972));
#83106=CARTESIAN_POINT('Ctrl Pts',(-16.3523190521331,2.12382120287335,0.23002251074712));
#83107=CARTESIAN_POINT('Ctrl Pts',(-16.4158738302987,2.08193010866575,0.234831074233356));
#83108=CARTESIAN_POINT('Ctrl Pts',(-16.4458340838878,2.06123644956739,0.237106273146607));
#83109=CARTESIAN_POINT('Ctrl Pts',(-16.5164631128415,2.01015473018781,0.242497126511684));
#83110=CARTESIAN_POINT('Ctrl Pts',(-16.5566829838664,1.97917180465407,0.24558925166422));
#83111=CARTESIAN_POINT('Ctrl Pts',(-16.7442991373719,1.82538369300179,0.260176814510257));
#83112=CARTESIAN_POINT('Ctrl Pts',(-16.8782700861455,1.68721986885628,0.271036910978185));
#83113=CARTESIAN_POINT('Ctrl Pts',(-17.0392174994968,1.4780377503028,0.286288042746235));
#83114=CARTESIAN_POINT('Ctrl Pts',(-17.0807027192118,1.41904144931832,0.290485770188388));
#83115=CARTESIAN_POINT('Ctrl Pts',(-17.1455044627881,1.31792350532712,0.297648848234922));
#83116=CARTESIAN_POINT('Ctrl Pts',(-17.1702483661582,1.27676668014217,0.300556367568883));
#83117=CARTESIAN_POINT('Ctrl Pts',(-17.2053952931272,1.21432974395098,0.304993664207599));
#83118=CARTESIAN_POINT('Ctrl Pts',(-17.2167006205197,1.19356750296359,0.306473444302919));
#83119=CARTESIAN_POINT('Ctrl Pts',(-17.2373822371722,1.15427814178871,0.309287409043184));
#83120=CARTESIAN_POINT('Ctrl Pts',(-17.2468245989627,1.13578888961816,0.310617695718588));
#83121=CARTESIAN_POINT('Ctrl Pts',(-17.270915964066,1.08713897474704,0.314130599103508));
#83122=CARTESIAN_POINT('Ctrl Pts',(-17.285192619967,1.05679936520077,0.316333500626808));
#83123=CARTESIAN_POINT('Ctrl Pts',(-17.3214038409402,0.975679075861538,
0.32223831725814));
#83124=CARTESIAN_POINT('Ctrl Pts',(-17.3422709041098,0.924461039268354,
0.325981378466721));
#83125=CARTESIAN_POINT('Ctrl Pts',(-17.3614291533995,0.872615954171733,
0.32975881722873));
#83126=CARTESIAN_POINT('Origin',(-15.,0.,3.));
#83127=CARTESIAN_POINT('',(-17.361429188522,0.872615859124936,1.33336838650867));
#83128=CARTESIAN_POINT('',(-17.3614291890287,0.872615857753796,1.05617159787625));
#83129=CARTESIAN_POINT('',(-17.3614291890287,0.872615857753799,3.));
#83130=CARTESIAN_POINT('',(-17.5174978061968,-0.00332352138350004,0.1125849952481));
#83131=CARTESIAN_POINT('Ctrl Pts',(-17.3614291890287,0.872615857753796,
1.05617159787625));
#83132=CARTESIAN_POINT('Ctrl Pts',(-17.3326448870889,0.950510489374704,
1.05093100125945));
#83133=CARTESIAN_POINT('Ctrl Pts',(-17.2999832020769,1.02703116401984,1.04569040464266));
#83134=CARTESIAN_POINT('Ctrl Pts',(-17.2636046805941,1.10177134651095,1.04044980802587));
#83135=CARTESIAN_POINT('Ctrl Pts',(-17.2272362206276,1.17649085747555,1.03521066084535));
#83136=CARTESIAN_POINT('Ctrl Pts',(-17.1871531677912,1.2494304402801,1.02997151366483));
#83137=CARTESIAN_POINT('Ctrl Pts',(-17.1435634096145,1.32020534727064,1.02473236648432));
#83138=CARTESIAN_POINT('Ctrl Pts',(-17.0999725941995,1.39098197085576,1.01949309223205));
#83139=CARTESIAN_POINT('Ctrl Pts',(-17.0528751474684,1.45959342265606,1.01425381797978));
#83140=CARTESIAN_POINT('Ctrl Pts',(-17.0025232141706,1.52568247899355,1.00901454372751));
#83141=CARTESIAN_POINT('Ctrl Pts',(-16.952120986379,1.59183754899549,1.00377003617776));
#83142=CARTESIAN_POINT('Ctrl Pts',(-16.8984580591094,1.65546482379302,0.998525528628003));
#83143=CARTESIAN_POINT('Ctrl Pts',(-16.841827645515,1.71623925319773,0.993281021078248));
#83144=CARTESIAN_POINT('Ctrl Pts',(-16.7851691135384,1.77704385858963,0.988033909502522));
#83145=CARTESIAN_POINT('Ctrl Pts',(-16.7255404910154,1.83499247532486,0.982786797926795));
#83146=CARTESIAN_POINT('Ctrl Pts',(-16.6632709798934,1.88979784565554,0.977539686351068));
#83147=CARTESIAN_POINT('Ctrl Pts',(-16.6008925738527,1.94469905785563,0.972283398795334));
#83148=CARTESIAN_POINT('Ctrl Pts',(-16.5358644134693,1.99644575379372,0.9670271112396));
#83149=CARTESIAN_POINT('Ctrl Pts',(-16.4685476759482,2.04479191446642,0.961770823683865));
#83150=CARTESIAN_POINT('Ctrl Pts',(-16.4104051657852,2.08654924320464,0.957230886606063));
#83151=CARTESIAN_POINT('Ctrl Pts',(-16.350556005376,2.12577036497012,0.95269094952826));
#83152=CARTESIAN_POINT('Ctrl Pts',(-16.2892476054404,2.16232441180002,0.948151012450456));
#83153=CARTESIAN_POINT('Ctrl Pts',(-16.2182438678792,2.2046591318487,0.942893127704567));
#83154=CARTESIAN_POINT('Ctrl Pts',(-16.1450230554184,2.24357016117157,0.937635242958676));
#83155=CARTESIAN_POINT('Ctrl Pts',(-16.0699488301934,2.27881893768853,0.932377358212785));
#83156=CARTESIAN_POINT('Ctrl Pts',(-15.9949803266762,2.31401807585302,0.927126877773143));
#83157=CARTESIAN_POINT('Ctrl Pts',(-15.918164008624,2.34556501121923,0.921876397333499));
#83158=CARTESIAN_POINT('Ctrl Pts',(-15.8398902335713,2.37326581856131,0.916625916893855));
#83159=CARTESIAN_POINT('Ctrl Pts',(-15.7613129936211,2.4010740210387,0.911355080511142));
#83160=CARTESIAN_POINT('Ctrl Pts',(-15.6812673759639,2.42500596976104,0.906084244128428));
#83161=CARTESIAN_POINT('Ctrl Pts',(-15.6001709003809,2.4449133195956,0.900813407745713));
#83162=CARTESIAN_POINT('Ctrl Pts',(-15.5195303896874,2.46470874036663,0.895572206637671));
#83163=CARTESIAN_POINT('Ctrl Pts',(-15.4378512585436,2.48052458758556,0.890331005529628));
#83164=CARTESIAN_POINT('Ctrl Pts',(-15.3555598645567,2.49226471963081,0.885089804421585));
#83165=CARTESIAN_POINT('Ctrl Pts',(-15.2732951560398,2.50400104458363,0.87985030293131));
#83166=CARTESIAN_POINT('Ctrl Pts',(-15.1904190349098,2.51166421436965,0.874610801441035));
#83167=CARTESIAN_POINT('Ctrl Pts',(-15.1073665468774,2.51520946933086,0.86937129995076));
#83168=CARTESIAN_POINT('Ctrl Pts',(-15.024316013629,2.51875464084836,0.864131921781214));
#83169=CARTESIAN_POINT('Ctrl Pts',(-14.9410895822175,2.5181820716874,0.858892543611667));
#83170=CARTESIAN_POINT('Ctrl Pts',(-14.858124511103,2.51349907412958,0.85365316544212));
#83171=CARTESIAN_POINT('Ctrl Pts',(-14.7742954033543,2.50876730566861,0.848359221964331));
#83172=CARTESIAN_POINT('Ctrl Pts',(-14.6907336115004,2.49983900301017,0.843065278486542));
#83173=CARTESIAN_POINT('Ctrl Pts',(-14.6078853482802,2.4867754924614,0.837771335008753));
#83174=CARTESIAN_POINT('Ctrl Pts',(-14.5257736899565,2.47382812974075,0.832524460045574));
#83175=CARTESIAN_POINT('Ctrl Pts',(-14.4443633662088,2.4568189551323,0.827277585082395));
#83176=CARTESIAN_POINT('Ctrl Pts',(-14.3640771794608,2.4358588662559,0.822030710119216));
#83177=CARTESIAN_POINT('Ctrl Pts',(-14.2827106491997,2.41461673513823,0.816713232384122));
#83178=CARTESIAN_POINT('Ctrl Pts',(-14.2024992013692,2.38931671685081,0.811395754649029));
#83179=CARTESIAN_POINT('Ctrl Pts',(-14.1238638879225,2.36012537021103,0.806078276913937));
#83180=CARTESIAN_POINT('Ctrl Pts',(-14.0452285744758,2.33093402357125,0.800760799178844));
#83181=CARTESIAN_POINT('Ctrl Pts',(-13.9681698167597,2.29785159865797,0.795443321443751));
#83182=CARTESIAN_POINT('Ctrl Pts',(-13.893082930489,2.26109284445046,0.79012584370866));
#83183=CARTESIAN_POINT('Ctrl Pts',(-13.8189474965226,2.22479987332616,0.784875745601297));
#83184=CARTESIAN_POINT('Ctrl Pts',(-13.7464608376546,2.18478938452908,0.779625647493936));
#83185=CARTESIAN_POINT('Ctrl Pts',(-13.6760207366242,2.14123449443323,0.774375549386575));
#83186=CARTESIAN_POINT('Ctrl Pts',(-13.605680399304,2.09774129075429,0.769132886948089));
#83187=CARTESIAN_POINT('Ctrl Pts',(-13.5373812527803,2.05071389740047,0.763890224509603));
#83188=CARTESIAN_POINT('Ctrl Pts',(-13.4714983702567,2.00037221983111,0.758647562071117));
#83189=CARTESIAN_POINT('Ctrl Pts',(-13.405236922355,1.94974127719816,0.753374775108442));
#83190=CARTESIAN_POINT('Ctrl Pts',(-13.3414200243656,1.89575804321547,0.748101988145768));
#83191=CARTESIAN_POINT('Ctrl Pts',(-13.2804014184089,1.83869164576061,0.742829201183094));
#83192=CARTESIAN_POINT('Ctrl Pts',(-13.219839031771,1.78205191804966,0.73759583739699));
#83193=CARTESIAN_POINT('Ctrl Pts',(-13.1620335767745,1.72237529581021,0.732362473610887));
#83194=CARTESIAN_POINT('Ctrl Pts',(-13.1072979450464,1.65996541565613,0.727129109824783));
#83195=CARTESIAN_POINT('Ctrl Pts',(-13.0525799854307,1.59757568534566,0.721897435698419));
#83196=CARTESIAN_POINT('Ctrl Pts',(-13.0009301854049,1.53245479702817,0.716665761572055));
#83197=CARTESIAN_POINT('Ctrl Pts',(-12.9526231667737,1.4649417574663,0.711434087445692));
#83198=CARTESIAN_POINT('Ctrl Pts',(-12.9043170984839,1.39743004608469,0.706202516241761));
#83199=CARTESIAN_POINT('Ctrl Pts',(-12.8593539490163,1.32752665371892,0.700970945037832));
#83200=CARTESIAN_POINT('Ctrl Pts',(-12.8179659397959,1.25560089602911,0.695739373833902));
#83201=CARTESIAN_POINT('Ctrl Pts',(-12.7760110637684,1.18269001425678,0.690436148928323));
#83202=CARTESIAN_POINT('Ctrl Pts',(-12.7377302625247,1.107701362593,0.685132924022745));
#83203=CARTESIAN_POINT('Ctrl Pts',(-12.7033171764188,1.03104522590768,0.679829699117166));
#83204=CARTESIAN_POINT('Ctrl Pts',(-12.6693195724963,0.955314587707073,
0.67459050204845));
#83205=CARTESIAN_POINT('Ctrl Pts',(-12.6390969079577,0.877956970031112,
0.669351304979735));
#83206=CARTESIAN_POINT('Ctrl Pts',(-12.6127865685549,0.799386191229341,
0.664112107911019));
#83207=CARTESIAN_POINT('Ctrl Pts',(-12.585993924107,0.719375100980596,0.658776869087008));
#83208=CARTESIAN_POINT('Ctrl Pts',(-12.5632586093974,0.638106412233824,
0.653441630262997));
#83209=CARTESIAN_POINT('Ctrl Pts',(-12.5446715529995,0.556029196490907,
0.648106391438986));
#83210=CARTESIAN_POINT('Ctrl Pts',(-12.5260844966017,0.473951980747991,
0.642771152614975));
#83211=CARTESIAN_POINT('Ctrl Pts',(-12.5116457181982,0.391066741099775,
0.637435913790963));
#83212=CARTESIAN_POINT('Ctrl Pts',(-12.5013906609342,0.307827257943743,
0.632100674966951));
#83213=CARTESIAN_POINT('Ctrl Pts',(-12.4912682527072,0.225664476457947,
0.626834447390188));
#83214=CARTESIAN_POINT('Ctrl Pts',(-12.485184536481,0.142853551862634,0.621568219813424));
#83215=CARTESIAN_POINT('Ctrl Pts',(-12.4832109210679,0.0598245950088185,
0.61630199223666));
#83216=CARTESIAN_POINT('Ctrl Pts',(-12.4812400963258,-0.0230869597886339,
0.611043211049327));
#83217=CARTESIAN_POINT('Ctrl Pts',(-12.4833678382513,-0.106215478942918,
0.605784429861994));
#83218=CARTESIAN_POINT('Ctrl Pts',(-12.4896139375275,-0.189124475793081,
0.60052564867466));
#83219=CARTESIAN_POINT('Ctrl Pts',(-12.4958718842765,-0.272190732724241,
0.595256892739267));
#83220=CARTESIAN_POINT('Ctrl Pts',(-12.5062638709878,-0.355036171088218,
0.589988136803874));
#83221=CARTESIAN_POINT('Ctrl Pts',(-12.5207572668831,-0.437220448157504,
0.584719380868481));
#83222=CARTESIAN_POINT('Ctrl Pts',(-12.5351972505915,-0.519101853352908,
0.579470041761221));
#83223=CARTESIAN_POINT('Ctrl Pts',(-12.5537083992556,-0.600326505241181,
0.574220702653961));
#83224=CARTESIAN_POINT('Ctrl Pts',(-12.5762066114153,-0.680464443929934,
0.568971363546702));
#83225=CARTESIAN_POINT('Ctrl Pts',(-12.5986971988316,-0.760575223518061,
0.563723803463601));
#83226=CARTESIAN_POINT('Ctrl Pts',(-12.6251720416696,-0.839599579622999,
0.558476243380501));
#83227=CARTESIAN_POINT('Ctrl Pts',(-12.6554965123832,-0.917120301025145,
0.5532286832974));
#83228=CARTESIAN_POINT('Ctrl Pts',(-12.6858197490691,-0.994637867789994,
0.547981336759123));
#83229=CARTESIAN_POINT('Ctrl Pts',(-12.7199921338847,-1.07065149415662,
0.542733990220846));
#83230=CARTESIAN_POINT('Ctrl Pts',(-12.7578304822127,-1.14476290274696,
0.537486643682569));
#83231=CARTESIAN_POINT('Ctrl Pts',(-12.7959350221214,-1.21939568274665,
0.532202382227788));
#83232=CARTESIAN_POINT('Ctrl Pts',(-12.8377571101419,-1.29209894713812,
0.526918120773007));
#83233=CARTESIAN_POINT('Ctrl Pts',(-12.8830629103333,-1.36249169112816,
0.521633859318227));
#83234=CARTESIAN_POINT('Ctrl Pts',(-12.9281139033789,-1.4324885349443,0.516379317404273));
#83235=CARTESIAN_POINT('Ctrl Pts',(-12.9766092089694,-1.50020043601646,
0.51112477549032));
#83236=CARTESIAN_POINT('Ctrl Pts',(-13.028276749544,-1.5652838955318,0.505870233576366));
#83237=CARTESIAN_POINT('Ctrl Pts',(-13.0803826353464,-1.63091952036352,
0.500571112351172));
#83238=CARTESIAN_POINT('Ctrl Pts',(-13.1357145248397,-1.69388153391925,
0.495271991125978));
#83239=CARTESIAN_POINT('Ctrl Pts',(-13.1939548016703,-1.75385489467925,
0.489972869900785));
#83240=CARTESIAN_POINT('Ctrl Pts',(-13.2521950785009,-1.81382825543925,
0.484673748675591));
#83241=CARTESIAN_POINT('Ctrl Pts',(-13.3133433562412,-1.87081268452723,
0.479374627450397));
#83242=CARTESIAN_POINT('Ctrl Pts',(-13.3770487753447,-1.92453515748345,
0.474075506225204));
#83243=CARTESIAN_POINT('Ctrl Pts',(-13.4403122453009,-1.97788493685339,
0.468813147054786));
#83244=CARTESIAN_POINT('Ctrl Pts',(-13.5063221429355,-2.02820737021692,
0.463550787884368));
#83245=CARTESIAN_POINT('Ctrl Pts',(-13.5747571460486,-2.07520819612405,
0.458288428713951));
#83246=CARTESIAN_POINT('Ctrl Pts',(-13.6430971283048,-2.12214376217075,
0.453033376241201));
#83247=CARTESIAN_POINT('Ctrl Pts',(-13.7138551510125,-2.16576662421337,
0.447778323768452));
#83248=CARTESIAN_POINT('Ctrl Pts',(-13.7866764018457,-2.2058223174503,0.442523271295703));
#83249=CARTESIAN_POINT('Ctrl Pts',(-13.8597007062691,-2.24598970133012,
0.437253565720193));
#83250=CARTESIAN_POINT('Ctrl Pts',(-13.934799399838,-2.28256969880127,0.431983860144683));
#83251=CARTESIAN_POINT('Ctrl Pts',(-14.0115848495443,-2.31534916164921,
0.426714154569173));
#83252=CARTESIAN_POINT('Ctrl Pts',(-14.0880244836537,-2.34798099692506,
0.421468181958519));
#83253=CARTESIAN_POINT('Ctrl Pts',(-14.166135289611,-2.37684627000409,0.416222209347864));
#83254=CARTESIAN_POINT('Ctrl Pts',(-14.2455112625665,-2.40178121299297,
0.41097623673721));
#83255=CARTESIAN_POINT('Ctrl Pts',(-14.3248624773042,-2.42670837850555,
0.405731900401708));
#83256=CARTESIAN_POINT('Ctrl Pts',(-14.4054776368251,-2.44770751123073,
0.400487564066206));
#83257=CARTESIAN_POINT('Ctrl Pts',(-14.486933900383,-2.46466416118379,0.395243227730705));
#83258=CARTESIAN_POINT('Ctrl Pts',(-14.5683891181309,-2.48162059343187,
0.389998958726788));
#83259=CARTESIAN_POINT('Ctrl Pts',(-14.6506849680177,-2.4945345535338,0.384754689722871));
#83260=CARTESIAN_POINT('Ctrl Pts',(-14.7333880403175,-2.50334262795852,
0.379510420718955));
#83261=CARTESIAN_POINT('Ctrl Pts',(-14.816786124462,-2.51222472280211,0.374222080449331));
#83262=CARTESIAN_POINT('Ctrl Pts',(-14.9005978372215,-2.51693152990207,
0.368933740179708));
#83263=CARTESIAN_POINT('Ctrl Pts',(-14.9843748973317,-2.51745151019173,
0.363645399910085));
#83264=CARTESIAN_POINT('Ctrl Pts',(-15.0675738836329,-2.51796790254232,
0.358393549951753));
#83265=CARTESIAN_POINT('Ctrl Pts',(-15.1507382326642,-2.51435514771791,
0.353141699993422));
#83266=CARTESIAN_POINT('Ctrl Pts',(-15.2334320679974,-2.50665428801629,
0.34788985003509));
#83267=CARTESIAN_POINT('Ctrl Pts',(-15.3169877492946,-2.49887316894799,
0.342583264609821));
#83268=CARTESIAN_POINT('Ctrl Pts',(-15.4000625758693,-2.48691830414295,
0.337276679184551));
#83269=CARTESIAN_POINT('Ctrl Pts',(-15.4822173048577,-2.47088500762294,
0.331970093759281));
#83270=CARTESIAN_POINT('Ctrl Pts',(-15.564372033846,-2.45485171110292,0.326663508334012));
#83271=CARTESIAN_POINT('Ctrl Pts',(-15.6456062166517,-2.43474015815058,
0.321356922908741));
#83272=CARTESIAN_POINT('Ctrl Pts',(-15.7254979597234,-2.41069677903239,
0.316050337483472));
#83273=CARTESIAN_POINT('Ctrl Pts',(-15.8038427307388,-2.38711896036145,
0.310846505347241));
#83274=CARTESIAN_POINT('Ctrl Pts',(-15.8811971867098,-2.35966961191086,
0.305642673211009));
#83275=CARTESIAN_POINT('Ctrl Pts',(-15.9571460064262,-2.32844964995647,
0.300438841074778));
#83276=CARTESIAN_POINT('Ctrl Pts',(-16.0329861558088,-2.29727435865922,
0.295242454770849));
#83277=CARTESIAN_POINT('Ctrl Pts',(-16.1074242298212,-2.26233934147627,
0.29004606846692));
#83278=CARTESIAN_POINT('Ctrl Pts',(-16.1800592325574,-2.22379550715799,
0.28484968216299));
#83279=CARTESIAN_POINT('Ctrl Pts',(-16.2539238564564,-2.18459917318267,
0.279565327437105));
#83280=CARTESIAN_POINT('Ctrl Pts',(-16.325923316285,-2.14167083002662,0.27428097271122));
#83281=CARTESIAN_POINT('Ctrl Pts',(-16.3956564509007,-2.09522059007142,
0.268996617985334));
#83282=CARTESIAN_POINT('Ctrl Pts',(-16.4641097169547,-2.04962288890042,
0.263809251291323));
#83283=CARTESIAN_POINT('Ctrl Pts',(-16.5303787408325,-2.00063175712121,
0.258621884597311));
#83284=CARTESIAN_POINT('Ctrl Pts',(-16.5941099988484,-1.94849161188122,
0.253434517903299));
#83285=CARTESIAN_POINT('Ctrl Pts',(-16.6578228501835,-1.89636652560982,
0.248248649409796));
#83286=CARTESIAN_POINT('Ctrl Pts',(-16.7189990257932,-1.84109452913811,
0.243062780916293));
#83287=CARTESIAN_POINT('Ctrl Pts',(-16.7773169667484,-1.7829612025247,0.237876912422789));
#83288=CARTESIAN_POINT('Ctrl Pts',(-16.835636496752,-1.72482629189317,0.23269090262463));
#83289=CARTESIAN_POINT('Ctrl Pts',(-16.8910973045054,-1.66383022991061,
0.22750489282647));
#83290=CARTESIAN_POINT('Ctrl Pts',(-16.9434147849419,-1.60029535513585,
0.222318883028311));
#83291=CARTESIAN_POINT('Ctrl Pts',(-16.9974654145893,-1.53465572651663,
0.21696107350443));
#83292=CARTESIAN_POINT('Ctrl Pts',(-17.0481604449311,-1.46630652813774,
0.211603263980548));
#83293=CARTESIAN_POINT('Ctrl Pts',(-17.0952326766386,-1.39563830584638,
0.206245454456667));
#83294=CARTESIAN_POINT('Ctrl Pts',(-17.1408716867421,-1.32712173898402,
0.201050775680607));
#83295=CARTESIAN_POINT('Ctrl Pts',(-17.1831051609906,-1.25642578881495,
0.195856096904547));
#83296=CARTESIAN_POINT('Ctrl Pts',(-17.2217359743982,-1.18393222359437,
0.190661418128487));
#83297=CARTESIAN_POINT('Ctrl Pts',(-17.2621864980569,-1.10802383812701,
0.185222043230696));
#83298=CARTESIAN_POINT('Ctrl Pts',(-17.2986863508818,-1.03014485341659,
0.179782668332903));
#83299=CARTESIAN_POINT('Ctrl Pts',(-17.3310662766949,-0.950755627727631,
0.174343293435112));
#83300=CARTESIAN_POINT('Ctrl Pts',(-17.363446202508,-0.871366402038671,
0.16890391853732));
#83301=CARTESIAN_POINT('Ctrl Pts',(-17.3917060957219,-0.790467515069941,
0.163464543639529));
#83302=CARTESIAN_POINT('Ctrl Pts',(-17.415737281965,-0.708533439242165,
0.158025168741737));
#83303=CARTESIAN_POINT('Ctrl Pts',(-17.4466522592493,-0.603129150523376,
0.151027671834813));
#83304=CARTESIAN_POINT('Ctrl Pts',(-17.4706689005917,-0.495685522224355,
0.144030174927888));
#83305=CARTESIAN_POINT('Ctrl Pts',(-17.4875795798172,-0.386980728301084,
0.137032678020964));
#83306=CARTESIAN_POINT('Ctrl Pts',(-17.5040746181104,-0.280947746745211,
0.130207169837831));
#83307=CARTESIAN_POINT('Ctrl Pts',(-17.5138087928967,-0.173714442495203,
0.123381661654697));
#83308=CARTESIAN_POINT('Ctrl Pts',(-17.5166340645248,-0.0660245050990958,
0.116556153471564));
#83309=CARTESIAN_POINT('Ctrl Pts',(-17.5171819895709,-0.0451394286573785,
0.115232434063742));
#83310=CARTESIAN_POINT('Ctrl Pts',(-17.5174701965452,-0.0242372539493491,
0.113908714655921));
#83311=CARTESIAN_POINT('Ctrl Pts',(-17.5174978061968,-0.00332352138350004,
0.1125849952481));
#83312=CARTESIAN_POINT('Ctrl Pts',(-17.5174977222504,-0.00338651208338963,
0.111633905503722));
#83313=CARTESIAN_POINT('Ctrl Pts',(-17.5176325157458,0.0968175649154425,
0.104703074197213));
#83314=CARTESIAN_POINT('Ctrl Pts',(-17.5117846136227,0.196948044376628,
0.0978488253944215));
#83315=CARTESIAN_POINT('Ctrl Pts',(-17.4930720434123,0.354740893766269,
0.0872175436775509));
#83316=CARTESIAN_POINT('Ctrl Pts',(-17.4841264447284,0.412754141523008,
0.0833447591150981));
#83317=CARTESIAN_POINT('Ctrl Pts',(-17.4647998011908,0.514364129027663,
0.0766202001912281));
#83318=CARTESIAN_POINT('Ctrl Pts',(-17.4552678085838,0.558093984067512,
0.0737454561072239));
#83319=CARTESIAN_POINT('Ctrl Pts',(-17.4351215394682,0.63996442595149,0.0683922448439606));
#83320=CARTESIAN_POINT('Ctrl Pts',(-17.4247638172419,0.678153421756895,
0.0659072083612793));
#83321=CARTESIAN_POINT('Ctrl Pts',(-17.3981285586884,0.767925649809322,
0.0600836889126596));
#83322=CARTESIAN_POINT('Ctrl Pts',(-17.3810802704562,0.819260452293542,
0.0567682006828312));
#83323=CARTESIAN_POINT('Ctrl Pts',(-17.3620708144642,0.870878048526862,
0.053433613536233));
#83324=CARTESIAN_POINT('Ctrl Pts',(-17.3617502393738,0.87174704744106,0.0533774743223632));
#83325=CARTESIAN_POINT('Ctrl Pts',(-17.3614291890837,0.87261585760501,0.0533213468502636));
#83326=CARTESIAN_POINT('Ctrl Pts',(-17.3614291533995,0.872615954171733,
0.32975881722873));
#83327=CARTESIAN_POINT('Ctrl Pts',(-17.3835552367282,0.81273946672832,0.334121424873797));
#83328=CARTESIAN_POINT('Ctrl Pts',(-17.4034020623706,0.752026587676025,
0.338529625453672));
#83329=CARTESIAN_POINT('Ctrl Pts',(-17.4531844221817,0.577514795597414,
0.351064346283168));
#83330=CARTESIAN_POINT('Ctrl Pts',(-17.4774840866728,0.462291736318107,
0.359172488206155));
#83331=CARTESIAN_POINT('Ctrl Pts',(-17.5043312932454,0.268682296977471,
0.372328516818489));
#83332=CARTESIAN_POINT('Ctrl Pts',(-17.5114419898486,0.191119310229726,
0.377479436103626));
#83333=CARTESIAN_POINT('Ctrl Pts',(-17.516765524736,0.0729979165311001,
0.385137648848412));
#83334=CARTESIAN_POINT('Ctrl Pts',(-17.5176127964505,0.0326116499114517,
0.387723534903136));
#83335=CARTESIAN_POINT('Ctrl Pts',(-17.5173777526979,-0.0434495297615438,
0.392536475026815));
#83336=CARTESIAN_POINT('Ctrl Pts',(-17.5165094300388,-0.0791145299421246,
0.394769609835801));
#83337=CARTESIAN_POINT('Ctrl Pts',(-17.512756247774,-0.161369606599533,
0.399871355794675));
#83338=CARTESIAN_POINT('Ctrl Pts',(-17.5093331267655,-0.207922573269812,
0.402722574830289));
#83339=CARTESIAN_POINT('Ctrl Pts',(-17.4851893986466,-0.44566352085408,
0.417141889270126));
#83340=CARTESIAN_POINT('Ctrl Pts',(-17.4439084327773,-0.634113327432651,
0.428041337479941));
#83341=CARTESIAN_POINT('Ctrl Pts',(-17.3567675779103,-0.888430637067505,
0.44353417009997));
#83342=CARTESIAN_POINT('Ctrl Pts',(-17.328675493853,-0.959651781800779,
0.447973517484615));
#83343=CARTESIAN_POINT('Ctrl Pts',(-17.2770363992305,-1.07488963855831,
0.455485754108116));
#83344=CARTESIAN_POINT('Ctrl Pts',(-17.2553467882276,-1.11968417693967,
0.458492215238968));
#83345=CARTESIAN_POINT('Ctrl Pts',(-17.22134321923,-1.1849080213295,0.463041553373214));
#83346=CARTESIAN_POINT('Ctrl Pts',(-17.2100423362815,-1.20585467002197,
0.464529576566361));
#83347=CARTESIAN_POINT('Ctrl Pts',(-17.1883793902625,-1.24468020096113,
0.467344452902078));
#83348=CARTESIAN_POINT('Ctrl Pts',(-17.178091180958,-1.26259726143376,0.468666972891903));
#83349=CARTESIAN_POINT('Ctrl Pts',(-17.1509413459817,-1.30855966361013,
0.472117585430802));
#83350=CARTESIAN_POINT('Ctrl Pts',(-17.1337516128707,-1.33640595664184,
0.474264573196645));
#83351=CARTESIAN_POINT('Ctrl Pts',(-17.039450929768,-1.48270809215482,0.485816722063119));
#83352=CARTESIAN_POINT('Ctrl Pts',(-16.9530134946302,-1.59484054879456,
0.495621793098598));
#83353=CARTESIAN_POINT('Ctrl Pts',(-16.7867718132438,-1.7765910223426,0.512615649130391));
#83354=CARTESIAN_POINT('Ctrl Pts',(-16.7111297343397,-1.84955869676579,
0.519816267343447));
#83355=CARTESIAN_POINT('Ctrl Pts',(-16.5753940732101,-1.96501836852654,
0.531769505265099));
#83356=CARTESIAN_POINT('Ctrl Pts',(-16.5175957902642,-2.00999214156221,
0.536598870876882));
#83357=CARTESIAN_POINT('Ctrl Pts',(-16.4253816490581,-2.0754965339777,0.543913253657244));
#83358=CARTESIAN_POINT('Ctrl Pts',(-16.3923023927518,-2.09783055844111,
0.546464668245145));
#83359=CARTESIAN_POINT('Ctrl Pts',(-16.3282267632005,-2.13890873584394,
0.55127513820568));
#83360=CARTESIAN_POINT('Ctrl Pts',(-16.2973299084303,-2.15778873827146,
0.553538786079863));
#83361=CARTESIAN_POINT('Ctrl Pts',(-16.2229613386796,-2.20105775470535,
0.558862953888334));
#83362=CARTESIAN_POINT('Ctrl Pts',(-16.1791508181441,-2.22483561864094,
0.561901341018575));
#83363=CARTESIAN_POINT('Ctrl Pts',(-16.031732719489,-2.29926701070143,0.571841499385341));
#83364=CARTESIAN_POINT('Ctrl Pts',(-15.9253512859313,-2.34410529944111,
0.578556408502827));
#83365=CARTESIAN_POINT('Ctrl Pts',(-15.7198547933984,-2.41453963987603,
0.591090054750961));
#83366=CARTESIAN_POINT('Ctrl Pts',(-15.621532021519,-2.44169809770156,0.596912617368568));
#83367=CARTESIAN_POINT('Ctrl Pts',(-15.4662160344018,-2.4746073215871,0.606164010612973));
#83368=CARTESIAN_POINT('Ctrl Pts',(-15.4102151392395,-2.48450430093974,
0.609511242558185));
#83369=CARTESIAN_POINT('Ctrl Pts',(-15.31329076579,-2.49826740769255,0.615394868078066));
#83370=CARTESIAN_POINT('Ctrl Pts',(-15.2725184440567,-2.50304303151205,
0.617897181194153));
#83371=CARTESIAN_POINT('Ctrl Pts',(-15.2093224815791,-2.50888284619231,
0.621842671508584));
#83372=CARTESIAN_POINT('Ctrl Pts',(-15.1869691012376,-2.51064762646456,
0.623251156667712));
#83373=CARTESIAN_POINT('Ctrl Pts',(-15.1426703040893,-2.51355012673629,
0.626073189435645));
#83374=CARTESIAN_POINT('Ctrl Pts',(-15.1207277961168,-2.51469953492058,
0.627486072094262));
#83375=CARTESIAN_POINT('Ctrl Pts',(-15.0599929579003,-2.51708430562984,
0.631433278272996));
#83376=CARTESIAN_POINT('Ctrl Pts',(-15.0211840009243,-2.51770995525376,
0.633996569152672));
#83377=CARTESIAN_POINT('Ctrl Pts',(-14.8108185964556,-2.51623745568275,
0.648060437220967));
#83378=CARTESIAN_POINT('Ctrl Pts',(-14.6398367497722,-2.49750295198875,
0.660066422047367));
#83379=CARTESIAN_POINT('Ctrl Pts',(-14.35541507125,-2.43650493710748,0.679999278915355));
#83380=CARTESIAN_POINT('Ctrl Pts',(-14.2406522768677,-2.40321527523799,
0.688039210490641));
#83381=CARTESIAN_POINT('Ctrl Pts',(-14.0863649710764,-2.34629722665468,
0.698772555634754));
#83382=CARTESIAN_POINT('Ctrl Pts',(-14.0444837528991,-2.32955548769909,
0.701679465851918));
#83383=CARTESIAN_POINT('Ctrl Pts',(-13.9702810714025,-2.29755531859551,
0.706821705188407));
#83384=CARTESIAN_POINT('Ctrl Pts',(-13.9377929040945,-2.28271719880701,
0.709070337008699));
#83385=CARTESIAN_POINT('Ctrl Pts',(-13.8673524649943,-2.24871571480265,
0.713944720421659));
#83386=CARTESIAN_POINT('Ctrl Pts',(-13.8295473321898,-2.22927200851229,
0.716560034462634));
#83387=CARTESIAN_POINT('Ctrl Pts',(-13.7113806484636,-2.16466200265832,
0.724750958268619));
#83388=CARTESIAN_POINT('Ctrl Pts',(-13.6329951294246,-2.11603438860291,
0.730206023229071));
#83389=CARTESIAN_POINT('Ctrl Pts',(-13.4196449813503,-1.96686468615854,
0.745380059179249));
#83390=CARTESIAN_POINT('Ctrl Pts',(-13.2918501599983,-1.85695934035244,
0.754848757100814));
#83391=CARTESIAN_POINT('Ctrl Pts',(-13.1317932005299,-1.68870299272427,
0.768507028295722));
#83392=CARTESIAN_POINT('Ctrl Pts',(-13.0894098215822,-1.64059692989384,
0.772336417259867));
#83393=CARTESIAN_POINT('Ctrl Pts',(-13.0322553293579,-1.57050369135047,
0.777898153398103));
#83394=CARTESIAN_POINT('Ctrl Pts',(-13.0159217702844,-1.54981753055592,
0.779537513498898));
#83395=CARTESIAN_POINT('Ctrl Pts',(-12.9874979582772,-1.51263344933187,
0.782488384671607));
#83396=CARTESIAN_POINT('Ctrl Pts',(-12.9752789007632,-1.49623821614062,
0.783791345813231));
#83397=CARTESIAN_POINT('Ctrl Pts',(-12.9463398442183,-1.45640482452355,
0.786961001506182));
#83398=CARTESIAN_POINT('Ctrl Pts',(-12.9298204131927,-1.43282635194578,
0.788839760972054));
#83399=CARTESIAN_POINT('Ctrl Pts',(-12.859914929169,-1.32931597502486,0.797080747082635));
#83400=CARTESIAN_POINT('Ctrl Pts',(-12.810730703438,-1.24665219944856,0.803641852284902));
#83401=CARTESIAN_POINT('Ctrl Pts',(-12.6708138783061,-0.977561493700402,
0.824522576820951));
#83402=CARTESIAN_POINT('Ctrl Pts',(-12.5982717066286,-0.782600715743599,
0.838889060123552));
#83403=CARTESIAN_POINT('Ctrl Pts',(-12.5404867268985,-0.538946144549989,
0.855297518861489));
#83404=CARTESIAN_POINT('Ctrl Pts',(-12.5316094548605,-0.496706126852236,
0.858092548642426));
#83405=CARTESIAN_POINT('Ctrl Pts',(-12.5172701717136,-0.41854189053908,
0.863176754644976));
#83406=CARTESIAN_POINT('Ctrl Pts',(-12.5114914821592,-0.382688246636222,
0.865475263860691));
#83407=CARTESIAN_POINT('Ctrl Pts',(-12.5011014050085,-0.307965941793777,
0.870200535121905));
#83408=CARTESIAN_POINT('Ctrl Pts',(-12.4966166167801,-0.269089410729553,
0.8726227556154));
#83409=CARTESIAN_POINT('Ctrl Pts',(-12.4867492458804,-0.161593964858977,
0.879232219953701));
#83410=CARTESIAN_POINT('Ctrl Pts',(-12.4832709270209,-0.0928327669313311,
0.883360757948777));
#83411=CARTESIAN_POINT('Ctrl Pts',(-12.4817107107369,0.0707466317847089,
0.893028132897282));
#83412=CARTESIAN_POINT('Ctrl Pts',(-12.486157761215,0.165483170982915,0.898502500759125));
#83413=CARTESIAN_POINT('Ctrl Pts',(-12.5127570854783,0.421911468866452,
0.913335932456505));
#83414=CARTESIAN_POINT('Ctrl Pts',(-12.5452893646556,0.582039038458692,
0.92260511854225));
#83415=CARTESIAN_POINT('Ctrl Pts',(-12.6020148425295,0.767076418174483,
0.934408471148048));
#83416=CARTESIAN_POINT('Ctrl Pts',(-12.6114967506365,0.796109965945524,
0.936294311449801));
#83417=CARTESIAN_POINT('Ctrl Pts',(-12.6282544910687,0.844425168184754,
0.939500706381289));
#83418=CARTESIAN_POINT('Ctrl Pts',(-12.6352429454685,0.863802444978699,
0.940805549043224));
#83419=CARTESIAN_POINT('Ctrl Pts',(-12.6513024419976,0.906675349002907,
0.943737317989772));
#83420=CARTESIAN_POINT('Ctrl Pts',(-12.6604889263279,0.930122692365925,
0.945370142445873));
#83421=CARTESIAN_POINT('Ctrl Pts',(-12.6920802357719,1.00732519022705,0.950835216511538));
#83422=CARTESIAN_POINT('Ctrl Pts',(-12.7159972599234,1.06043769478327,0.954739033353897));
#83423=CARTESIAN_POINT('Ctrl Pts',(-12.7858793703816,1.20227013016722,0.965474745974864));
#83424=CARTESIAN_POINT('Ctrl Pts',(-12.8353188496068,1.2891617342377,0.972391216390137));
#83425=CARTESIAN_POINT('Ctrl Pts',(-12.9696476981395,1.49563399758236,0.989385977156253));
#83426=CARTESIAN_POINT('Ctrl Pts',(-13.0600756031843,1.61119692168597,0.999389481879473));
#83427=CARTESIAN_POINT('Ctrl Pts',(-13.1949281767611,1.7556005442937,1.01238688813328));
#83428=CARTESIAN_POINT('Ctrl Pts',(-13.2309367079026,1.79187980681812,1.01570340736094));
#83429=CARTESIAN_POINT('Ctrl Pts',(-13.2943801234735,1.85202205188942,1.02129517969685));
#83430=CARTESIAN_POINT('Ctrl Pts',(-13.3212718329469,1.87643193530091,1.02359336432171));
#83431=CARTESIAN_POINT('Ctrl Pts',(-13.3783380026123,1.92602235013558,1.0283279114817));
#83432=CARTESIAN_POINT('Ctrl Pts',(-13.4085929465998,1.95109548331557,1.0307595055537));
#83433=CARTESIAN_POINT('Ctrl Pts',(-13.4940547484666,2.0186089966816,1.0374265119159));
#83434=CARTESIAN_POINT('Ctrl Pts',(-13.5504554580865,2.05948421306682,1.04160153626649));
#83435=CARTESIAN_POINT('Ctrl Pts',(-13.6889747025622,2.15135963635004,1.05142000406807));
#83436=CARTESIAN_POINT('Ctrl Pts',(-13.7724762227648,2.20007328514741,1.0569959252357));
#83437=CARTESIAN_POINT('Ctrl Pts',(-13.9999715471583,2.31579713311458,1.07168128872143));
#83438=CARTESIAN_POINT('Ctrl Pts',(-14.1478353813586,2.3741897242527,1.08071679832936));
#83439=CARTESIAN_POINT('Ctrl Pts',(-14.3299749299033,2.42689806436197,1.0922727402276));
#83440=CARTESIAN_POINT('Ctrl Pts',(-14.3599169434052,2.43496638285326,1.09418625867067));
#83441=CARTESIAN_POINT('Ctrl Pts',(-14.4100528989628,2.44748767584125,1.09742490045056));
#83442=CARTESIAN_POINT('Ctrl Pts',(-14.4301659690668,2.45224848932349,1.09873355378819));
#83443=CARTESIAN_POINT('Ctrl Pts',(-14.4746919515494,2.46221050552374,1.10165420826288));
#83444=CARTESIAN_POINT('Ctrl Pts',(-14.4991257142135,2.46729689157235,1.10327166891477));
#83445=CARTESIAN_POINT('Ctrl Pts',(-14.5792526385346,2.48273774149783,1.10861511016226));
#83446=CARTESIAN_POINT('Ctrl Pts',(-14.6352172406197,2.49157532250733,1.11240858962044));
#83447=CARTESIAN_POINT('Ctrl Pts',(-14.7857773839676,2.51016983045862,1.12269915252817));
#83448=CARTESIAN_POINT('Ctrl Pts',(-14.8807081588065,2.51646818946665,1.12927404051608));
#83449=CARTESIAN_POINT('Ctrl Pts',(-15.1294620771118,2.51886306153653,1.1464446892016));
#83450=CARTESIAN_POINT('Ctrl Pts',(-15.2829923890487,2.50626395564869,1.15696427808092));
#83451=CARTESIAN_POINT('Ctrl Pts',(-15.484634773469,2.47093771492628,1.17042905232434));
#83452=CARTESIAN_POINT('Ctrl Pts',(-15.5345628333025,2.46061928034601,1.17373658441706));
#83453=CARTESIAN_POINT('Ctrl Pts',(-15.6194404852995,2.44037216436577,1.17931759947465));
#83454=CARTESIAN_POINT('Ctrl Pts',(-15.6545499493115,2.43119053174039,1.18161381551733));
#83455=CARTESIAN_POINT('Ctrl Pts',(-15.7272600474732,2.41048637662271,1.18634782926339));
#83456=CARTESIAN_POINT('Ctrl Pts',(-15.7648140403433,2.39883544671789,1.18878078244725));
#83457=CARTESIAN_POINT('Ctrl Pts',(-15.8682717451064,2.36406145098872,1.19546137755397));
#83458=CARTESIAN_POINT('Ctrl Pts',(-15.9335113184679,2.33906823684261,1.19964812237518));
#83459=CARTESIAN_POINT('Ctrl Pts',(-16.0867423289768,2.27293144358567,1.20950448362295));
#83460=CARTESIAN_POINT('Ctrl Pts',(-16.1735575998852,2.22934749926156,1.21510571054418));
#83461=CARTESIAN_POINT('Ctrl Pts',(-16.3943467622135,2.10202431611659,1.22976762849102));
#83462=CARTESIAN_POINT('Ctrl Pts',(-16.5233200012927,2.01052072242488,1.23875740209731));
#83463=CARTESIAN_POINT('Ctrl Pts',(-16.666434569669,1.88726511987068,1.25026600172275));
#83464=CARTESIAN_POINT('Ctrl Pts',(-16.6896244614534,1.86653228762496,1.25218513990339));
#83465=CARTESIAN_POINT('Ctrl Pts',(-16.7275772563391,1.831313865884,1.25542963989552));
#83466=CARTESIAN_POINT('Ctrl Pts',(-16.7425561710251,1.8170667610702,1.25673834793639));
#83467=CARTESIAN_POINT('Ctrl Pts',(-16.7751757085839,1.78526653022033,1.2596540881484));
#83468=CARTESIAN_POINT('Ctrl Pts',(-16.7927331828004,1.76763486006384,1.26126646309826));
#83469=CARTESIAN_POINT('Ctrl Pts',(-16.8490524592795,1.70937538113403,1.26657177865021));
#83470=CARTESIAN_POINT('Ctrl Pts',(-16.8867148416647,1.6677126047612,1.27033099157672));
#83471=CARTESIAN_POINT('Ctrl Pts',(-16.9833698683707,1.55332348173811,1.28048653997405));
#83472=CARTESIAN_POINT('Ctrl Pts',(-17.0397521464408,1.47850594623718,1.28695867289338));
#83473=CARTESIAN_POINT('Ctrl Pts',(-17.1786906859522,1.27101598920294,1.30419664743113));
#83474=CARTESIAN_POINT('Ctrl Pts',(-17.253304957287,1.13349204240167,1.31488676720222));
#83475=CARTESIAN_POINT('Ctrl Pts',(-17.3312570993131,0.951219606211523,
1.32792444222788));
#83476=CARTESIAN_POINT('Ctrl Pts',(-17.3468371067832,0.912104217466158,
1.33066246219695));
#83477=CARTESIAN_POINT('Ctrl Pts',(-17.361429188522,0.872615859124936,1.33336838650867));
#83478=CARTESIAN_POINT('Origin',(-15.,0.,3.));
#83479=CARTESIAN_POINT('',(-17.3614291132577,0.87261606280125,2.3307189689843));
#83480=CARTESIAN_POINT('',(-17.3614291890287,0.872615857753798,2.05625951847909));
#83481=CARTESIAN_POINT('',(-17.3614291890287,0.872615857753799,3.));
#83482=CARTESIAN_POINT('',(-17.5174999225306,0.000624546553775974,1.11258330254393));
#83483=CARTESIAN_POINT('Ctrl Pts',(-17.3614291890287,0.872615857753798,
2.0562595184791));
#83484=CARTESIAN_POINT('Ctrl Pts',(-17.3579183588427,0.88211668999871,2.05561541020025));
#83485=CARTESIAN_POINT('Ctrl Pts',(-17.3543505691999,0.891595309335236,
2.05497130192141));
#83486=CARTESIAN_POINT('Ctrl Pts',(-17.3507261017234,0.901051077728782,
2.05432719364256));
#83487=CARTESIAN_POINT('Ctrl Pts',(-17.3211460982113,0.978221493550537,
2.04907049723843));
#83488=CARTESIAN_POINT('Ctrl Pts',(-17.2877077514437,1.05407531900084,2.0438138008343));
#83489=CARTESIAN_POINT('Ctrl Pts',(-17.2505489208352,1.12820025036668,2.03855710443017));
#83490=CARTESIAN_POINT('Ctrl Pts',(-17.2134425427188,1.2022205488011,2.03330782824949));
#83491=CARTESIAN_POINT('Ctrl Pts',(-17.1726263174307,1.27451639191413,2.02805855206882));
#83492=CARTESIAN_POINT('Ctrl Pts',(-17.1282867028638,1.34469400251988,2.02280927588814));
#83493=CARTESIAN_POINT('Ctrl Pts',(-17.0837624472362,1.41516384995711,2.01753814043034));
#83494=CARTESIAN_POINT('Ctrl Pts',(-17.0356855587209,1.48349734301016,2.01226700497253));
#83495=CARTESIAN_POINT('Ctrl Pts',(-16.9842922536276,1.54931936739762,2.00699586951473));
#83496=CARTESIAN_POINT('Ctrl Pts',(-16.9332028355715,1.61475218817319,2.00175590211925));
#83497=CARTESIAN_POINT('Ctrl Pts',(-16.8788363990628,1.67770279135969,1.99651593472378));
#83498=CARTESIAN_POINT('Ctrl Pts',(-16.821468216685,1.73783192098843,1.99127596732831));
#83499=CARTESIAN_POINT('Ctrl Pts',(-16.7641187321055,1.79794145295363,1.98603770777592));
#83500=CARTESIAN_POINT('Ctrl Pts',(-16.7037697628315,1.85523100441582,1.98079944822352));
#83501=CARTESIAN_POINT('Ctrl Pts',(-16.6407352069614,1.9093963000481,1.97556118867113));
#83502=CARTESIAN_POINT('Ctrl Pts',(-16.5777022129079,1.9635602536187,1.97032305890788));
#83503=CARTESIAN_POINT('Ctrl Pts',(-16.5119841149943,2.0145998055727,1.96508492914463));
#83504=CARTESIAN_POINT('Ctrl Pts',(-16.443928775299,2.06225021320485,1.95984679938138));
#83505=CARTESIAN_POINT('Ctrl Pts',(-16.3751293912855,2.11042157944539,1.954551401508));
#83506=CARTESIAN_POINT('Ctrl Pts',(-16.303941731054,2.15512895127721,1.94925600363462));
#83507=CARTESIAN_POINT('Ctrl Pts',(-16.2307547169103,2.1961441384397,1.94396060576124));
#83508=CARTESIAN_POINT('Ctrl Pts',(-16.1582556254288,2.23677380260915,1.93871498207588));
#83509=CARTESIAN_POINT('Ctrl Pts',(-16.0837950534331,2.27378024822346,1.93346935839053));
#83510=CARTESIAN_POINT('Ctrl Pts',(-16.0077736161152,2.30698907423987,1.92822373470517));
#83511=CARTESIAN_POINT('Ctrl Pts',(-15.9306701610406,2.34067056350356,1.92290344973778));
#83512=CARTESIAN_POINT('Ctrl Pts',(-15.8519615197173,2.37044530624312,1.91758316477039));
#83513=CARTESIAN_POINT('Ctrl Pts',(-15.7720823641435,2.39618343892504,1.912262879803));
#83514=CARTESIAN_POINT('Ctrl Pts',(-15.6922032085696,2.42192157160695,1.90694259483561));
#83515=CARTESIAN_POINT('Ctrl Pts',(-15.6111540266284,2.44362302983869,1.90162230986822));
#83516=CARTESIAN_POINT('Ctrl Pts',(-15.5293791044952,2.46121189939506,1.89630202490083));
#83517=CARTESIAN_POINT('Ctrl Pts',(-15.4485811111899,2.47859064250592,1.89104529902492));
#83518=CARTESIAN_POINT('Ctrl Pts',(-15.3667782505564,2.4920183248603,1.88578857314902));
#83519=CARTESIAN_POINT('Ctrl Pts',(-15.2843911870634,2.5013851967901,1.88053184727311));
#83520=CARTESIAN_POINT('Ctrl Pts',(-15.202120412429,2.51073884743493,1.87528254123506));
#83521=CARTESIAN_POINT('Ctrl Pts',(-15.1192675272454,2.51604302130111,1.87003323519701));
#83522=CARTESIAN_POINT('Ctrl Pts',(-15.0362642248042,2.51723879598248,1.86478392915895));
#83523=CARTESIAN_POINT('Ctrl Pts',(-14.9529158675402,2.51843954164464,1.85951280111729));
#83524=CARTESIAN_POINT('Ctrl Pts',(-14.8694162997541,2.51549755241802,1.85424167307563));
#83525=CARTESIAN_POINT('Ctrl Pts',(-14.7862087535634,2.50840577916474,1.84897054503397));
#83526=CARTESIAN_POINT('Ctrl Pts',(-14.7034926121531,2.50135588830601,1.8437305470717));
#83527=CARTESIAN_POINT('Ctrl Pts',(-14.6210655169452,2.4902051330005,1.83849054910942));
#83528=CARTESIAN_POINT('Ctrl Pts',(-14.5393620086488,2.47499876584291,1.83325055114714));
#83529=CARTESIAN_POINT('Ctrl Pts',(-14.4576851264548,2.45979735424106,1.82801226083152));
#83530=CARTESIAN_POINT('Ctrl Pts',(-14.3767318157995,2.44054304008941,1.82277397051589));
#83531=CARTESIAN_POINT('Ctrl Pts',(-14.2969284164376,2.41733253781665,1.81753568020027));
#83532=CARTESIAN_POINT('Ctrl Pts',(-14.2171269920321,2.3941226099521,1.81229751952065));
#83533=CARTESIAN_POINT('Ctrl Pts',(-14.138475864793,2.36695681844558,1.80705935884104));
#83534=CARTESIAN_POINT('Ctrl Pts',(-14.0613868143877,2.33598192154707,1.80182119816143));
#83535=CARTESIAN_POINT('Ctrl Pts',(-13.983455945087,2.30466877617673,1.7965258363279));
#83536=CARTESIAN_POINT('Ctrl Pts',(-13.9071219299059,2.26946298869584,1.79123047449437));
#83537=CARTESIAN_POINT('Ctrl Pts',(-13.8327883460253,2.23056566924753,1.78593511266085));
#83538=CARTESIAN_POINT('Ctrl Pts',(-13.7591525261008,2.19203347611339,1.78068945800447));
#83539=CARTESIAN_POINT('Ctrl Pts',(-13.6874801096723,2.14987905464921,1.77544380334809));
#83540=CARTESIAN_POINT('Ctrl Pts',(-13.6181360221196,2.10434269942812,1.77019814869171));
#83541=CARTESIAN_POINT('Ctrl Pts',(-13.5478062905234,2.05815909887048,1.76487793326961));
#83542=CARTESIAN_POINT('Ctrl Pts',(-13.4798719930558,2.00849695994764,1.7595577178475));
#83543=CARTESIAN_POINT('Ctrl Pts',(-13.4146793346692,1.95564941594221,1.7542375024254));
#83544=CARTESIAN_POINT('Ctrl Pts',(-13.3494866762826,1.90280187193678,1.7489172870033));
#83545=CARTESIAN_POINT('Ctrl Pts',(-13.2870359773928,1.84676929628926,1.7435970715812));
#83546=CARTESIAN_POINT('Ctrl Pts',(-13.2276335093517,1.78788234311626,1.7382768561591));
#83547=CARTESIAN_POINT('Ctrl Pts',(-13.1689417340556,1.7296999150544,1.73302029193916));
#83548=CARTESIAN_POINT('Ctrl Pts',(-13.1130102909223,1.66851762084859,1.72776372771923));
#83549=CARTESIAN_POINT('Ctrl Pts',(-13.0601608943265,1.60462783663376,1.72250716349929));
#83550=CARTESIAN_POINT('Ctrl Pts',(-13.0073861005807,1.54082824001408,1.71725801950924));
#83551=CARTESIAN_POINT('Ctrl Pts',(-12.9576850030239,1.47432909740031,1.71200887551918));
#83552=CARTESIAN_POINT('Ctrl Pts',(-12.9113427684534,1.40545978921783,1.70675973152913));
#83553=CARTESIAN_POINT('Ctrl Pts',(-12.8648060897557,1.33630151714207,1.70148856302447));
#83554=CARTESIAN_POINT('Ctrl Pts',(-12.8216568603807,1.26475347508018,1.69621739451981));
#83555=CARTESIAN_POINT('Ctrl Pts',(-12.7821431293703,1.19118308895007,1.69094622601516));
#83556=CARTESIAN_POINT('Ctrl Pts',(-12.7428642719539,1.11805001259977,1.68570638986662));
#83557=CARTESIAN_POINT('Ctrl Pts',(-12.7071780338311,1.04291897808977,1.68046655371808));
#83558=CARTESIAN_POINT('Ctrl Pts',(-12.6752838786094,0.966178660987118,
1.67522671756955));
#83559=CARTESIAN_POINT('Ctrl Pts',(-12.6434001148738,0.889463346770761,
1.66998858862046));
#83560=CARTESIAN_POINT('Ctrl Pts',(-12.6153061570237,0.811140216822043,
1.66475045967138));
#83561=CARTESIAN_POINT('Ctrl Pts',(-12.5911538838185,0.731619189577037,
1.6595123307223));
#83562=CARTESIAN_POINT('Ctrl Pts',(-12.5670022052839,0.652100120276801,
1.65427433074498));
#83563=CARTESIAN_POINT('Ctrl Pts',(-12.5467921514062,0.5713836538708,1.64903633076766));
#83564=CARTESIAN_POINT('Ctrl Pts',(-12.5306257299106,0.489894850167558,
1.64379833079034));
#83565=CARTESIAN_POINT('Ctrl Pts',(-12.5142816764258,0.407510670928604,
1.63850277717592));
#83566=CARTESIAN_POINT('Ctrl Pts',(-12.5020707728335,0.324337546161918,
1.63320722356151));
#83567=CARTESIAN_POINT('Ctrl Pts',(-12.4940450286002,0.240823444283986,
1.62791166994709));
#83568=CARTESIAN_POINT('Ctrl Pts',(-12.4860951479878,0.158098762300121,
1.62266617273368));
#83569=CARTESIAN_POINT('Ctrl Pts',(-12.48225159958,0.0750399909802926,1.61742067552027));
#83570=CARTESIAN_POINT('Ctrl Pts',(-12.4825124454019,-0.00791596132666538,
1.61217517830687));
#83571=CARTESIAN_POINT('Ctrl Pts',(-12.4827770249985,-0.0920593539025686,
1.60685459649195));
#83572=CARTESIAN_POINT('Ctrl Pts',(-12.4872644023026,-0.176096469374805,
1.60153401467703));
#83573=CARTESIAN_POINT('Ctrl Pts',(-12.4959181350515,-0.259577086115441,
1.59621343286211));
#83574=CARTESIAN_POINT('Ctrl Pts',(-12.5045718678004,-0.343057702856078,
1.59089285104719));
#83575=CARTESIAN_POINT('Ctrl Pts',(-12.5173918181152,-0.425981348228918,
1.58557226923227));
#83576=CARTESIAN_POINT('Ctrl Pts',(-12.5342682813868,-0.507910761674344,
1.58025168741735));
#83577=CARTESIAN_POINT('Ctrl Pts',(-12.5509424231166,-0.588857973756139,
1.57499489078646));
#83578=CARTESIAN_POINT('Ctrl Pts',(-12.5716374750143,-0.669131681034995,
1.56973809415557));
#83579=CARTESIAN_POINT('Ctrl Pts',(-12.5962842586559,-0.748302669255232,
1.56448129752468));
#83580=CARTESIAN_POINT('Ctrl Pts',(-12.6208962491726,-0.82736189416728,
1.55923192175584));
#83581=CARTESIAN_POINT('Ctrl Pts',(-12.6494487546389,-0.905321055478407,
1.553982545987));
#83582=CARTESIAN_POINT('Ctrl Pts',(-12.6818216371413,-0.981761339620741,
1.54873317021816));
#83583=CARTESIAN_POINT('Ctrl Pts',(-12.7143285575393,-1.05851811997933,
1.54346205973722));
#83584=CARTESIAN_POINT('Ctrl Pts',(-12.7506874683974,-1.13374295575044,
1.53819094925628));
#83585=CARTESIAN_POINT('Ctrl Pts',(-12.7907261182731,-1.20702740876898,
1.53291983877534));
#83586=CARTESIAN_POINT('Ctrl Pts',(-12.8305289487565,-1.27988023146951,
1.5276797740483));
#83587=CARTESIAN_POINT('Ctrl Pts',(-12.8739680684985,-1.35081505642381,
1.52243970932127));
#83588=CARTESIAN_POINT('Ctrl Pts',(-12.9208268601991,-1.41945246652737,
1.51719964459423));
#83589=CARTESIAN_POINT('Ctrl Pts',(-12.9676703702129,-1.48806749245554,
1.51196128876803));
#83590=CARTESIAN_POINT('Ctrl Pts',(-13.0179310774233,-1.55438621109506,
1.50672293294184));
#83591=CARTESIAN_POINT('Ctrl Pts',(-13.0713485773765,-1.61805745881054,
1.50148457711564));
#83592=CARTESIAN_POINT('Ctrl Pts',(-13.1247647417676,-1.6817271145962,1.49624635226057));
#83593=CARTESIAN_POINT('Ctrl Pts',(-13.18133724479,-1.74274907852124,1.4910081274055));
#83594=CARTESIAN_POINT('Ctrl Pts',(-13.2407657562769,-1.80080568793864,
1.48576990255042));
#83595=CARTESIAN_POINT('Ctrl Pts',(-13.3008415902188,-1.85949467642785,
1.48047462056086));
#83596=CARTESIAN_POINT('Ctrl Pts',(-13.3638356979858,-1.91515296809219,
1.47517933857129));
#83597=CARTESIAN_POINT('Ctrl Pts',(-13.4294013462705,-1.96749234278134,
1.46988405658172));
#83598=CARTESIAN_POINT('Ctrl Pts',(-13.4943532602625,-2.01934178913228,
1.46463834164795));
#83599=CARTESIAN_POINT('Ctrl Pts',(-13.5618283590093,-2.06793397067668,
1.45939262671418));
#83600=CARTESIAN_POINT('Ctrl Pts',(-13.6314596067478,-2.11303181283129,
1.45414691178041));
#83601=CARTESIAN_POINT('Ctrl Pts',(-13.7020777788575,-2.15876885306085,
1.44882684626295));
#83602=CARTESIAN_POINT('Ctrl Pts',(-13.7749132735029,-2.2009114778222,1.44350678074548));
#83603=CARTESIAN_POINT('Ctrl Pts',(-13.8495582965948,-2.23926106943028,
1.43818671522802));
#83604=CARTESIAN_POINT('Ctrl Pts',(-13.9242033196866,-2.27761066103836,
1.43286664971055));
#83605=CARTESIAN_POINT('Ctrl Pts',(-14.0006574004068,-2.31216707685132,
1.42754658419309));
#83606=CARTESIAN_POINT('Ctrl Pts',(-14.0784945104588,-2.34278336231618,
1.42222651867563));
#83607=CARTESIAN_POINT('Ctrl Pts',(-14.1554076983103,-2.37303623416223,
1.41696960204225));
#83608=CARTESIAN_POINT('Ctrl Pts',(-14.2339532309517,-2.399552974658,1.41171268540887));
#83609=CARTESIAN_POINT('Ctrl Pts',(-14.3137337737756,-2.42215707928773,
1.40645576877549));
#83610=CARTESIAN_POINT('Ctrl Pts',(-14.3934017384898,-2.44472928732614,
1.40120627016305));
#83611=CARTESIAN_POINT('Ctrl Pts',(-14.4743008117969,-2.46339970165732,
1.39595677155062));
#83612=CARTESIAN_POINT('Ctrl Pts',(-14.5560145367786,-2.4780401849946,1.39070727293818));
#83613=CARTESIAN_POINT('Ctrl Pts',(-14.6380641997092,-2.49274085765681,
1.385436192813));
#83614=CARTESIAN_POINT('Ctrl Pts',(-14.720934789805,-2.50337821665985,1.38016511268782));
#83615=CARTESIAN_POINT('Ctrl Pts',(-14.8041901146933,-2.50987345075726,
1.37489403256264));
#83616=CARTESIAN_POINT('Ctrl Pts',(-14.886957593483,-2.51633062513155,1.36965383906096));
#83617=CARTESIAN_POINT('Ctrl Pts',(-14.9701048461394,-2.51869404784475,
1.36441364555928));
#83618=CARTESIAN_POINT('Ctrl Pts',(-15.0531957172911,-2.51693791454257,
1.3591734520576));
#83619=CARTESIAN_POINT('Ctrl Pts',(-15.1362595218497,-2.51518235329535,
1.35393496553267));
#83620=CARTESIAN_POINT('Ctrl Pts',(-15.2192665207753,-2.50930991101445,
1.34869647900775));
#83621=CARTESIAN_POINT('Ctrl Pts',(-15.301780307132,-2.49934689393595,1.34345799248282));
#83622=CARTESIAN_POINT('Ctrl Pts',(-15.3842920577936,-2.48938412265476,
1.33821963519645));
#83623=CARTESIAN_POINT('Ctrl Pts',(-15.4663101624699,-2.47533103357443,
1.33298127791007));
#83624=CARTESIAN_POINT('Ctrl Pts',(-15.5474044670369,-2.45726567539369,
1.3277429206237));
#83625=CARTESIAN_POINT('Ctrl Pts',(-15.629377676138,-2.43900452386718,1.32244778973288));
#83626=CARTESIAN_POINT('Ctrl Pts',(-15.7104064662015,-2.41664369278313,
1.31715265884206));
#83627=CARTESIAN_POINT('Ctrl Pts',(-15.790060066662,-2.3903161592279,1.31185752795124));
#83628=CARTESIAN_POINT('Ctrl Pts',(-15.8689723476672,-2.36423365053935,
1.30661167773983));
#83629=CARTESIAN_POINT('Ctrl Pts',(-15.946534517254,-2.33425819292832,1.30136582752842));
#83630=CARTESIAN_POINT('Ctrl Pts',(-16.0223474854582,-2.30056772753537,
1.296119977317));
#83631=CARTESIAN_POINT('Ctrl Pts',(-16.0992287593984,-2.2664025185955,1.29080020608648));
#83632=CARTESIAN_POINT('Ctrl Pts',(-16.1743107126428,-2.22841701001766,
1.28548043485596));
#83633=CARTESIAN_POINT('Ctrl Pts',(-16.2472042958861,-2.18684423183801,
1.28016066362544));
#83634=CARTESIAN_POINT('Ctrl Pts',(-16.3200978791295,-2.14527145365836,
1.27484089239492));
#83635=CARTESIAN_POINT('Ctrl Pts',(-16.3908027158774,-2.10011172217429,
1.2695211211644));
#83636=CARTESIAN_POINT('Ctrl Pts',(-16.458963058855,-2.05164154834528,1.26420134993388));
#83637=CARTESIAN_POINT('Ctrl Pts',(-16.5258768594739,-2.00405781554877,
1.25897886870935));
#83638=CARTESIAN_POINT('Ctrl Pts',(-16.5905910504883,-1.9531040037354,1.25375638748483));
#83639=CARTESIAN_POINT('Ctrl Pts',(-16.6527433969628,-1.89901172028921,
1.2485339062603));
#83640=CARTESIAN_POINT('Ctrl Pts',(-16.7148077447634,-1.84499602364115,
1.24331881930885));
#83641=CARTESIAN_POINT('Ctrl Pts',(-16.7743171005252,-1.78785098331981,
1.2381037323574));
#83642=CARTESIAN_POINT('Ctrl Pts',(-16.8309390359885,-1.72785083166735,
1.23288864540595));
#83643=CARTESIAN_POINT('Ctrl Pts',(-16.8874968861012,-1.66791858886896,
1.22767946094923));
#83644=CARTESIAN_POINT('Ctrl Pts',(-16.9411734901439,-1.6051379942373,1.22247027649251));
#83645=CARTESIAN_POINT('Ctrl Pts',(-16.99167143653,-1.53982178803601,1.21726109203579));
#83646=CARTESIAN_POINT('Ctrl Pts',(-17.0421384923936,-1.47454553695928,
1.212055094133));
#83647=CARTESIAN_POINT('Ctrl Pts',(-17.0894304642487,-1.40673712186122,
1.20684909623022));
#83648=CARTESIAN_POINT('Ctrl Pts',(-17.1332894007877,-1.33674327471159,
1.20164309832743));
#83649=CARTESIAN_POINT('Ctrl Pts',(-17.1771351667822,-1.26677044624498,
1.19643866375091));
#83650=CARTESIAN_POINT('Ctrl Pts',(-17.2175496963465,-1.19461388511103,
1.19123422917439));
#83651=CARTESIAN_POINT('Ctrl Pts',(-17.2543185061784,-1.12064906313328,
1.18602979459787));
#83652=CARTESIAN_POINT('Ctrl Pts',(-17.2910877251957,-1.04668341803063,
1.18082530210328));
#83653=CARTESIAN_POINT('Ctrl Pts',(-17.3242109373603,-0.970909891917941,
1.17562080960869));
#83654=CARTESIAN_POINT('Ctrl Pts',(-17.3535204181281,-0.893726966950397,
1.1704163171141));
#83655=CARTESIAN_POINT('Ctrl Pts',(-17.3828581303628,-0.816469697875104,
1.16520681155022));
#83656=CARTESIAN_POINT('Ctrl Pts',(-17.4083746099405,-0.737800757540424,
1.15999730598634));
#83657=CARTESIAN_POINT('Ctrl Pts',(-17.4299511964776,-0.65813633294112,
1.15478780042246));
#83658=CARTESIAN_POINT('Ctrl Pts',(-17.4515386754913,-0.578431691466635,
1.14957566495149));
#83659=CARTESIAN_POINT('Ctrl Pts',(-17.4691822018905,-0.497731022518042,
1.14436352948052));
#83660=CARTESIAN_POINT('Ctrl Pts',(-17.4828142452473,-0.416460890837208,
1.13915139400955));
#83661=CARTESIAN_POINT('Ctrl Pts',(-17.4964690143288,-0.335055275239358,
1.13393056948499));
#83662=CARTESIAN_POINT('Ctrl Pts',(-17.5060988917234,-0.25307876606046,
1.12870974496043));
#83663=CARTESIAN_POINT('Ctrl Pts',(-17.5116882685441,-0.170962837066912,
1.12348892043587));
#83664=CARTESIAN_POINT('Ctrl Pts',(-17.5155800936491,-0.113786367447792,
1.11985371447189));
#83665=CARTESIAN_POINT('Ctrl Pts',(-17.517514104616,-0.0565423669010007,
1.11621850850791));
#83666=CARTESIAN_POINT('Ctrl Pts',(-17.5174999225306,0.000624546553782374,
1.11258330254393));
#83667=CARTESIAN_POINT('Ctrl Pts',(-17.5174999225304,0.000624547370669188,
1.11258330249198));
#83668=CARTESIAN_POINT('Ctrl Pts',(-17.5174915904523,0.0342104800950757,
1.11044759539204));
#83669=CARTESIAN_POINT('Ctrl Pts',(-17.5168111821614,0.0677873313081131,
1.10831188829209));
#83670=CARTESIAN_POINT('Ctrl Pts',(-17.5154596174,0.10133687990857,1.10617618119214));
#83671=CARTESIAN_POINT('Ctrl Pts',(-17.5121328106533,0.183917358347414,
1.10091924864084));
#83672=CARTESIAN_POINT('Ctrl Pts',(-17.5047290348594,0.266485049122924,
1.09566231608955));
#83673=CARTESIAN_POINT('Ctrl Pts',(-17.4932470011056,0.348605280335514,
1.09040538353826));
#83674=CARTESIAN_POINT('Ctrl Pts',(-17.4817792084923,0.430623658011649,
1.08515497114849));
#83675=CARTESIAN_POINT('Ctrl Pts',(-17.4662432595015,0.512195225028043,
1.07990455875871));
#83676=CARTESIAN_POINT('Ctrl Pts',(-17.4466898348291,0.592887090552553,
1.07465414636895));
#83677=CARTESIAN_POINT('Ctrl Pts',(-17.4271585183416,0.673487721384712,
1.06940967038622));
#83678=CARTESIAN_POINT('Ctrl Pts',(-17.4036188623419,0.753210181893953,
1.0641651944035));
#83679=CARTESIAN_POINT('Ctrl Pts',(-17.376172897285,0.831630093375674,1.05892071842078));
#83680=CARTESIAN_POINT('Ctrl Pts',(-17.371377231226,0.845332497611128,1.05800434490594));
#83681=CARTESIAN_POINT('Ctrl Pts',(-17.3664624273925,0.858995160992436,
1.05708797139109));
#83682=CARTESIAN_POINT('Ctrl Pts',(-17.3614291890287,0.872615857753796,
1.05617159787625));
#83683=CARTESIAN_POINT('',(-17.5174990715549,-0.00216211011121049,1.38677810957484));
#83684=CARTESIAN_POINT('Ctrl Pts',(-17.361429188522,0.872615859124936,1.33336838650867));
#83685=CARTESIAN_POINT('Ctrl Pts',(-17.3644697119384,0.864387747443512,
1.33393221464368));
#83686=CARTESIAN_POINT('Ctrl Pts',(-17.3674673419817,0.856143442814553,
1.3344946565356));
#83687=CARTESIAN_POINT('Ctrl Pts',(-17.3826366100634,0.813734815422654,
1.33737516686039));
#83688=CARTESIAN_POINT('Ctrl Pts',(-17.3941124149619,0.779325048998579,
1.33967013449361));
#83689=CARTESIAN_POINT('Ctrl Pts',(-17.4164783306267,0.707097202009639,
1.34440453398241));
#83690=CARTESIAN_POINT('Ctrl Pts',(-17.4272334213277,0.669247459917327,
1.3468390565592));
#83691=CARTESIAN_POINT('Ctrl Pts',(-17.4546538286454,0.563368980426638,
1.35353294537761));
#83692=CARTESIAN_POINT('Ctrl Pts',(-17.4693750492632,0.494871834409698,
1.3577309577425));
#83693=CARTESIAN_POINT('Ctrl Pts',(-17.5054861443727,0.284467611793582,
1.37033664236042));
#83694=CARTESIAN_POINT('Ctrl Pts',(-17.5176222639292,0.141279561221942,
1.37850634702139));
#83695=CARTESIAN_POINT('Ctrl Pts',(-17.5174990715549,-0.00216211011121049,
1.38677810957484));
#83696=CARTESIAN_POINT('Ctrl Pts',(-17.5174990700656,-0.00216384354887156,
1.38677820953593));
#83697=CARTESIAN_POINT('Ctrl Pts',(-17.51741074099,-0.104929297953376,1.39270432233761));
#83698=CARTESIAN_POINT('Ctrl Pts',(-17.5110300750471,-0.207586802734071,
1.3986753730216));
#83699=CARTESIAN_POINT('Ctrl Pts',(-17.4951445603227,-0.335795742753872,
1.40649579315783));
#83700=CARTESIAN_POINT('Ctrl Pts',(-17.4914808689594,-0.361978067002406,
1.4081122615719));
#83701=CARTESIAN_POINT('Ctrl Pts',(-17.4837484833002,-0.411536795135612,
1.41121705589603));
#83702=CARTESIAN_POINT('Ctrl Pts',(-17.4797602707,-0.434922935711898,1.41270135868087));
#83703=CARTESIAN_POINT('Ctrl Pts',(-17.4716560460498,-0.478701706731114,
1.41552195544408));
#83704=CARTESIAN_POINT('Ctrl Pts',(-17.4676167067343,-0.499105799734577,
1.41685425623413));
#83705=CARTESIAN_POINT('Ctrl Pts',(-17.4564238192827,-0.552183836688912,
1.42036299168395));
#83706=CARTESIAN_POINT('Ctrl Pts',(-17.4488712189477,-0.584768729881325,
1.42255945597878));
#83707=CARTESIAN_POINT('Ctrl Pts',(-17.4102116686093,-0.737647178732982,
1.43303559146702));
#83708=CARTESIAN_POINT('Ctrl Pts',(-17.3708778124791,-0.855673738076037,
1.44161771255737));
#83709=CARTESIAN_POINT('Ctrl Pts',(-17.2788507738176,-1.07599470455397,
1.4581025758057));
#83710=CARTESIAN_POINT('Ctrl Pts',(-17.2275401150562,-1.17855597735989,
1.46598750706981));
#83711=CARTESIAN_POINT('Ctrl Pts',(-17.1304437310446,-1.34347210301674,
1.47885632062811));
#83712=CARTESIAN_POINT('Ctrl Pts',(-17.0884552579023,-1.40785808502855,
1.48393584376869));
#83713=CARTESIAN_POINT('Ctrl Pts',(-17.0199887772231,-1.50302492600982,
1.49152602486034));
#83714=CARTESIAN_POINT('Ctrl Pts',(-16.9956066370565,-1.53525015779285,
1.49411198496748));
#83715=CARTESIAN_POINT('Ctrl Pts',(-16.9480725587814,-1.59502764224625,
1.49894337157539));
#83716=CARTESIAN_POINT('Ctrl Pts',(-16.9250853592536,-1.62269727486359,
1.5011944533973));
#83717=CARTESIAN_POINT('Ctrl Pts',(-16.8697954236546,-1.68642031891409,
1.50642021843077));
#83718=CARTESIAN_POINT('Ctrl Pts',(-16.8370297964,-1.72205412664812,1.5093749748587));
#83719=CARTESIAN_POINT('Ctrl Pts',(-16.6757701912873,-1.88758520926889,
1.5233064672854));
#83720=CARTESIAN_POINT('Ctrl Pts',(-16.5344199516149,-2.0041818450257,1.53370215386311));
#83721=CARTESIAN_POINT('Ctrl Pts',(-16.3147676298489,-2.14839492329636,
1.5488468285158));
#83722=CARTESIAN_POINT('Ctrl Pts',(-16.2457951060086,-2.18911119093644,
1.55348594542009));
#83723=CARTESIAN_POINT('Ctrl Pts',(-16.1297280120013,-2.25036481123439,
1.56128820626082));
#83724=CARTESIAN_POINT('Ctrl Pts',(-16.0837362709733,-2.27287089488973,
1.56437912776286));
#83725=CARTESIAN_POINT('Ctrl Pts',(-16.0151056212476,-2.30389868207061,
1.56903615911648));
#83726=CARTESIAN_POINT('Ctrl Pts',(-15.9929764674198,-2.31352246331369,
1.57054442940889));
#83727=CARTESIAN_POINT('Ctrl Pts',(-15.9516568138439,-2.33079002381752,
1.57337910231776));
#83728=CARTESIAN_POINT('Ctrl Pts',(-15.932504673425,-2.33851827849744,1.57470072485983));
#83729=CARTESIAN_POINT('Ctrl Pts',(-15.8830141027774,-2.35778409374209,
1.57813284331709));
#83730=CARTESIAN_POINT('Ctrl Pts',(-15.8525443724825,-2.36897184358824,
1.5802617180655));
#83731=CARTESIAN_POINT('Ctrl Pts',(-15.6851471818416,-2.42678846124556,
1.59201154403098));
#83732=CARTESIAN_POINT('Ctrl Pts',(-15.5446197952672,-2.46213581091885,
1.60205391088852));
#83733=CARTESIAN_POINT('Ctrl Pts',(-15.3000216729287,-2.50168594680716,
1.61914428558574));
#83734=CARTESIAN_POINT('Ctrl Pts',(-15.1972744133894,-2.51187807177734,
1.62621330117869));
#83735=CARTESIAN_POINT('Ctrl Pts',(-15.0218425278818,-2.51844592440845,
1.63798321193597));
#83736=CARTESIAN_POINT('Ctrl Pts',(-14.9494121099834,-2.51803286362245,
1.64275764569538));
#83737=CARTESIAN_POINT('Ctrl Pts',(-14.8374217325841,-2.51255889790163,
1.65000628215555));
#83738=CARTESIAN_POINT('Ctrl Pts',(-14.7977990828646,-2.50968105360116,
1.65254522002841));
#83739=CARTESIAN_POINT('Ctrl Pts',(-14.7222821257896,-2.50239593756581,
1.65733920875892));
#83740=CARTESIAN_POINT('Ctrl Pts',(-14.6863825826926,-2.49815071133972,
1.65959867450862));
#83741=CARTESIAN_POINT('Ctrl Pts',(-14.6011634235553,-2.48620717972852,
1.66492234893989));
#83742=CARTESIAN_POINT('Ctrl Pts',(-14.5519560815547,-2.47781232388039,
1.66796416099419));
#83743=CARTESIAN_POINT('Ctrl Pts',(-14.3887109287107,-2.44493972746542,
1.67798371300989));
#83744=CARTESIAN_POINT('Ctrl Pts',(-14.2761261381144,-2.41400389357336,
1.68476868986902));
#83745=CARTESIAN_POINT('Ctrl Pts',(-14.0497333614593,-2.33452464324547,
1.69860126208235));
#83746=CARTESIAN_POINT('Ctrl Pts',(-13.9365473921558,-2.28518661595405,
1.70562348887135));
#83747=CARTESIAN_POINT('Ctrl Pts',(-13.7699258323203,-2.19748667984402,
1.71669718811635));
#83748=CARTESIAN_POINT('Ctrl Pts',(-13.7136125135431,-2.16500254353319,
1.72058055858812));
#83749=CARTESIAN_POINT('Ctrl Pts',(-13.6365675149431,-2.11649177913667,
1.7261830698941));
#83750=CARTESIAN_POINT('Ctrl Pts',(-13.6147293085288,-2.10226320281731,
1.72780516773122));
#83751=CARTESIAN_POINT('Ctrl Pts',(-13.5761280782184,-2.07625015261861,
1.73074128529458));
#83752=CARTESIAN_POINT('Ctrl Pts',(-13.5592813794292,-2.06459577281768,
1.73204728911199));
#83753=CARTESIAN_POINT('Ctrl Pts',(-13.5187576025879,-2.03582433159446,
1.73524821981792));
#83754=CARTESIAN_POINT('Ctrl Pts',(-13.4952337354723,-2.0184989619937,1.7371559007093));
#83755=CARTESIAN_POINT('Ctrl Pts',(-13.3932583319858,-1.9406206173743,1.74562723661071));
#83756=CARTESIAN_POINT('Ctrl Pts',(-13.3181257297811,-1.87587915831881,
1.75240065805066));
#83757=CARTESIAN_POINT('Ctrl Pts',(-13.1485513295577,-1.71136289228862,
1.7686757924878));
#83758=CARTESIAN_POINT('Ctrl Pts',(-13.0580568401493,-1.60794485962692,
1.77818910802633));
#83759=CARTESIAN_POINT('Ctrl Pts',(-12.92628381013,-1.42990023747465,1.79315092028478));
#83760=CARTESIAN_POINT('Ctrl Pts',(-12.8795623454426,-1.35965445253963,
1.79874748437558));
#83761=CARTESIAN_POINT('Ctrl Pts',(-12.8152444318241,-1.25154681982423,
1.80690886825791));
#83762=CARTESIAN_POINT('Ctrl Pts',(-12.7949220216378,-1.2153837985722,1.80956844024252));
#83763=CARTESIAN_POINT('Ctrl Pts',(-12.7587470892079,-1.14711467822045,
1.81446383365772));
#83764=CARTESIAN_POINT('Ctrl Pts',(-12.7426681718462,-1.11514121202083,
1.81670716260732));
#83765=CARTESIAN_POINT('Ctrl Pts',(-12.7076214894262,-1.04158292537489,
1.82176278251821));
#83766=CARTESIAN_POINT('Ctrl Pts',(-12.6890931827839,-0.999802135017713,
1.82455957570571));
#83767=CARTESIAN_POINT('Ctrl Pts',(-12.5957800124775,-0.772907773260703,
1.83939378298238));
#83768=CARTESIAN_POINT('Ctrl Pts',(-12.5420789946517,-0.579905236458507,
1.85069849313828));
#83769=CARTESIAN_POINT('Ctrl Pts',(-12.5006395735616,-0.310384398969156,
1.86644851325316));
#83770=CARTESIAN_POINT('Ctrl Pts',(-12.4926875744485,-0.23774824482131,
1.87069821484972));
#83771=CARTESIAN_POINT('Ctrl Pts',(-12.4847373231454,-0.116614366871532,
1.87793454077127));
#83772=CARTESIAN_POINT('Ctrl Pts',(-12.4829614961188,-0.0682770984409923,
1.88086159378687));
#83773=CARTESIAN_POINT('Ctrl Pts',(-12.4823915276552,0.00374558707273863,
1.88532066291344));
#83774=CARTESIAN_POINT('Ctrl Pts',(-12.4825380175491,0.027413775255064,
1.88680173826362));
#83775=CARTESIAN_POINT('Ctrl Pts',(-12.4834406661178,0.0718961410599484,
1.88962072421106));
#83776=CARTESIAN_POINT('Ctrl Pts',(-12.4841214615025,0.0927091808764392,
1.89095475279585));
#83777=CARTESIAN_POINT('Ctrl Pts',(-12.4865752790908,0.14707614294081,1.89447540692934));
#83778=CARTESIAN_POINT('Ctrl Pts',(-12.4887620110582,0.180606545600921,
1.89668231750773));
#83779=CARTESIAN_POINT('Ctrl Pts',(-12.5018894485058,0.334420250930173,
1.90694011608563));
#83780=CARTESIAN_POINT('Ctrl Pts',(-12.5208057433837,0.453855449612457,
1.91527511630195));
#83781=CARTESIAN_POINT('Ctrl Pts',(-12.5746765633848,0.684981153922177,
1.93166030484436));
#83782=CARTESIAN_POINT('Ctrl Pts',(-12.6089896275729,0.796533844033761,
1.93969037957492));
#83783=CARTESIAN_POINT('Ctrl Pts',(-12.6788026686794,0.977683206159806,
1.95275092826776));
#83784=CARTESIAN_POINT('Ctrl Pts',(-12.7100246190622,1.04873079468747,1.95788126928044));
#83785=CARTESIAN_POINT('Ctrl Pts',(-12.7624746842335,1.15452495130637,1.9655279382062));
#83786=CARTESIAN_POINT('Ctrl Pts',(-12.7813432755363,1.19038231334867,1.96812139822791));
#83787=CARTESIAN_POINT('Ctrl Pts',(-12.8185698656697,1.25716371334219,1.97295889718402));
#83788=CARTESIAN_POINT('Ctrl Pts',(-12.836740667003,1.28817984125442,1.97520878757044));
#83789=CARTESIAN_POINT('Ctrl Pts',(-12.8808052193339,1.35983097479106,1.98042007034532));
#83790=CARTESIAN_POINT('Ctrl Pts',(-12.9072139489706,1.40013349607472,1.98336189575687));
#83791=CARTESIAN_POINT('Ctrl Pts',(-13.0402730523914,1.59101138787177,1.99739280564575));
#83792=CARTESIAN_POINT('Ctrl Pts',(-13.1620991728174,1.73031017383203,2.00788578632071));
#83793=CARTESIAN_POINT('Ctrl Pts',(-13.3564731192859,1.90864067087109,2.02309228407537));
#83794=CARTESIAN_POINT('Ctrl Pts',(-13.4173788092537,1.95943833674866,2.02768791156971));
#83795=CARTESIAN_POINT('Ctrl Pts',(-13.521149642625,2.03798857909398,2.03542747270723));
#83796=CARTESIAN_POINT('Ctrl Pts',(-13.5626430888984,2.06746225958091,2.03850063859477));
#83797=CARTESIAN_POINT('Ctrl Pts',(-13.6250440309144,2.1090002945182,2.04313621795057));
#83798=CARTESIAN_POINT('Ctrl Pts',(-13.6452796817278,2.12205535097268,2.04464155400268));
#83799=CARTESIAN_POINT('Ctrl Pts',(-13.6832257670378,2.14577237408993,2.0474743278546));
#83800=CARTESIAN_POINT('Ctrl Pts',(-13.700885631735,2.15650995782518,2.04879707906495));
#83801=CARTESIAN_POINT('Ctrl Pts',(-13.7467085747113,2.18360424707422,2.05223766802096));
#83802=CARTESIAN_POINT('Ctrl Pts',(-13.7750598594629,2.19963367834657,2.05437406875671));
#83803=CARTESIAN_POINT('Ctrl Pts',(-13.9298220662405,2.28321430957237,2.06604533588087));
#83804=CARTESIAN_POINT('Ctrl Pts',(-14.0615086621974,2.34042240477489,2.07599291910889));
#83805=CARTESIAN_POINT('Ctrl Pts',(-14.3432295227119,2.43519038608521,2.09649672266226));
#83806=CARTESIAN_POINT('Ctrl Pts',(-14.4933357030283,2.47079013715364,2.10699315412295));
#83807=CARTESIAN_POINT('Ctrl Pts',(-14.6924010604153,2.49908128460314,2.12015392998989));
#83808=CARTESIAN_POINT('Ctrl Pts',(-14.7392086029188,2.50439867176429,2.12319754377254));
#83809=CARTESIAN_POINT('Ctrl Pts',(-14.8218461732262,2.5114441320951,2.12848549235195));
#83810=CARTESIAN_POINT('Ctrl Pts',(-14.8576141947806,2.51372570310347,2.13074631920287));
#83811=CARTESIAN_POINT('Ctrl Pts',(-14.9344821854733,2.51698287105086,2.13554992572323));
#83812=CARTESIAN_POINT('Ctrl Pts',(-14.975582230692,2.51771710722279,2.13808460016937));
#83813=CARTESIAN_POINT('Ctrl Pts',(-15.0982874490642,2.51690390813561,2.14556671967149));
#83814=CARTESIAN_POINT('Ctrl Pts',(-15.1798211683558,2.5123956434932,2.15042415253401));
#83815=CARTESIAN_POINT('Ctrl Pts',(-15.3062221260613,2.4992202191508,2.15787237779834));
#83816=CARTESIAN_POINT('Ctrl Pts',(-15.3513112372926,2.4932818327974,2.16051331582906));
#83817=CARTESIAN_POINT('Ctrl Pts',(-15.5284859290761,2.46504536084989,2.17088356622319));
#83818=CARTESIAN_POINT('Ctrl Pts',(-15.6588566633258,2.43344427486408,2.17848822351278));
#83819=CARTESIAN_POINT('Ctrl Pts',(-15.8503054310333,2.37051812648493,2.19032009531502));
#83820=CARTESIAN_POINT('Ctrl Pts',(-15.9136405727218,2.34683507862466,2.19435203607397));
#83821=CARTESIAN_POINT('Ctrl Pts',(-16.0002522883677,2.31041061455897,2.20012982753585));
#83822=CARTESIAN_POINT('Ctrl Pts',(-16.0244007212841,2.29980539971069,2.20177019813175));
#83823=CARTESIAN_POINT('Ctrl Pts',(-16.0669780447957,2.28030320266165,2.2047227136022));
#83824=CARTESIAN_POINT('Ctrl Pts',(-16.0854725850685,2.27155761974723,2.20602629616552));
#83825=CARTESIAN_POINT('Ctrl Pts',(-16.1297459239671,2.24995779261166,2.20919749154462));
#83826=CARTESIAN_POINT('Ctrl Pts',(-16.1554133750856,2.23688526346347,2.21107717725398));
#83827=CARTESIAN_POINT('Ctrl Pts',(-16.2604189583063,2.18111611071466,2.21892147788057));
#83828=CARTESIAN_POINT('Ctrl Pts',(-16.3376557556887,2.13461885474172,2.22505880398839));
#83829=CARTESIAN_POINT('Ctrl Pts',(-16.514387399488,2.01486129009422,2.23973937716109));
#83830=CARTESIAN_POINT('Ctrl Pts',(-16.6113240810356,1.93821364535464,2.24830757315026));
#83831=CARTESIAN_POINT('Ctrl Pts',(-16.7769960424481,1.78616469138696,2.26362274608836));
#83832=CARTESIAN_POINT('Ctrl Pts',(-16.8475341111643,1.71310279774354,2.27041108134033));
#83833=CARTESIAN_POINT('Ctrl Pts',(-16.9417663073569,1.60288644711555,2.27985280603844));
#83834=CARTESIAN_POINT('Ctrl Pts',(-16.969194033204,1.56906870448489,2.28265325612637));
#83835=CARTESIAN_POINT('Ctrl Pts',(-17.0174709722588,1.50628316749648,2.28768464482899));
#83836=CARTESIAN_POINT('Ctrl Pts',(-17.0386072114135,1.47755167462609,2.28992644383609));
#83837=CARTESIAN_POINT('Ctrl Pts',(-17.0843707274607,1.41249077309344,2.29487517146996));
#83838=CARTESIAN_POINT('Ctrl Pts',(-17.1086732255476,1.37594662036801,2.29756940987837));
#83839=CARTESIAN_POINT('Ctrl Pts',(-17.1825020268267,1.25837449706739,2.30599320188743));
#83840=CARTESIAN_POINT('Ctrl Pts',(-17.2284082296537,1.17516840427878,2.31159607240119));
#83841=CARTESIAN_POINT('Ctrl Pts',(-17.3035351786815,1.01868229294143,2.321691433626));
#83842=CARTESIAN_POINT('Ctrl Pts',(-17.3342056011023,0.946286943855907,
2.32620193476533));
#83843=CARTESIAN_POINT('Ctrl Pts',(-17.3614291132577,0.872616062801249,
2.3307189689843));
#83844=CARTESIAN_POINT('Origin',(-15.,0.,3.));
#83845=CARTESIAN_POINT('',(-17.3614291865442,0.872615864477069,3.32953388487208));
#83846=CARTESIAN_POINT('',(-17.3591485432458,0.871797030805385,3.05636277808387));
#83847=CARTESIAN_POINT('',(-17.3614291890287,0.872615857753799,3.));
#83848=CARTESIAN_POINT('',(-17.5150210530422,0.00159552408394636,2.11258330249198));
#83849=CARTESIAN_POINT('Ctrl Pts',(-17.3591485432458,0.871797030805393,
3.05636277808387));
#83850=CARTESIAN_POINT('Ctrl Pts',(-17.2624742437046,1.13962407251414,3.03840125408691));
#83851=CARTESIAN_POINT('Ctrl Pts',(-16.7111054856786,2.12729618132246,2.96776467384271));
#83852=CARTESIAN_POINT('Ctrl Pts',(-14.6622990804118,2.95164362565941,2.84445303735124));
#83853=CARTESIAN_POINT('Ctrl Pts',(-12.3431875092431,1.32950737222075,2.6864278686095));
#83854=CARTESIAN_POINT('Ctrl Pts',(-12.435070079852,-1.49912548760771,2.52840269986778));
#83855=CARTESIAN_POINT('Ctrl Pts',(-14.8545655401893,-2.96733705322818,
2.37037753112603));
#83856=CARTESIAN_POINT('Ctrl Pts',(-17.0925050104093,-1.89324215569749,
2.2317710653341));
#83857=CARTESIAN_POINT('Ctrl Pts',(-17.5114957050982,-0.525856969687278,
2.14583965578942));
#83858=CARTESIAN_POINT('Ctrl Pts',(-17.514587964214,0.00159524933330165,
2.11258330249198));
#83859=CARTESIAN_POINT('Ctrl Pts',(-17.5174994934027,0.00159709640131535,
2.11258330249198));
#83860=CARTESIAN_POINT('Ctrl Pts',(-17.5174399084259,0.0955207624432348,
2.10666815241494));
#83861=CARTESIAN_POINT('Ctrl Pts',(-17.5121200573974,0.189246299150487,
2.1007530023379));
#83862=CARTESIAN_POINT('Ctrl Pts',(-17.5016305128836,0.282225135325527,
2.09483785226086));
#83863=CARTESIAN_POINT('Ctrl Pts',(-17.4910921020488,0.375637120304911,
2.08889514601847));
#83864=CARTESIAN_POINT('Ctrl Pts',(-17.4753358468603,0.468295220825688,
2.08295243977609));
#83865=CARTESIAN_POINT('Ctrl Pts',(-17.4545031557752,0.559661065547269,
2.0770097335337));
#83866=CARTESIAN_POINT('Ctrl Pts',(-17.4335578999204,0.651520585100958,
2.07103491721215));
#83867=CARTESIAN_POINT('Ctrl Pts',(-17.4074813199554,0.742073642382098,
2.0650601008906));
#83868=CARTESIAN_POINT('Ctrl Pts',(-17.3764652582008,0.830794274513616,
2.05908528456905));
#83869=CARTESIAN_POINT('Ctrl Pts',(-17.3715756163645,0.844780966894033,
2.05814336253907));
#83870=CARTESIAN_POINT('Ctrl Pts',(-17.36656330763,0.858722163962524,2.05720144050908));
#83871=CARTESIAN_POINT('Ctrl Pts',(-17.3614291890287,0.872615857753798,
2.0562595184791));
#83872=CARTESIAN_POINT('Ctrl Pts',(-17.3614291132577,0.872616062801249,
2.3307189689843));
#83873=CARTESIAN_POINT('Ctrl Pts',(-17.3869176511553,0.803640280654235,
2.33494812932253));
#83874=CARTESIAN_POINT('Ctrl Pts',(-17.4093845944515,0.733546376936331,
2.33918337490291));
#83875=CARTESIAN_POINT('Ctrl Pts',(-17.4475770545046,0.593537990326144,
2.34768363991974));
#83876=CARTESIAN_POINT('Ctrl Pts',(-17.4634478885576,0.523778120690173,
2.35193855498513));
#83877=CARTESIAN_POINT('Ctrl Pts',(-17.4811557921531,0.42707253811359,2.35797832605816));
#83878=CARTESIAN_POINT('Ctrl Pts',(-17.485562893351,0.400626985064299,2.35964437732084));
#83879=CARTESIAN_POINT('Ctrl Pts',(-17.4925832577244,0.353910301453609,
2.36262075381162));
#83880=CARTESIAN_POINT('Ctrl Pts',(-17.4953734322925,0.333669219728799,
2.36392175561438));
#83881=CARTESIAN_POINT('Ctrl Pts',(-17.5014365699172,0.285343125753982,
2.36705506296288));
#83882=CARTESIAN_POINT('Ctrl Pts',(-17.5044831872879,0.257234160904541,
2.36889855783631));
#83883=CARTESIAN_POINT('Ctrl Pts',(-17.5139636711795,0.153480180741025,
2.37576605195838));
#83884=CARTESIAN_POINT('Ctrl Pts',(-17.5174479275044,0.0776112731086758,
2.38090973185285));
#83885=CARTESIAN_POINT('Ctrl Pts',(-17.5176287541216,-0.188935286467546,
2.39917147469878));
#83886=CARTESIAN_POINT('Ctrl Pts',(-17.4961013173271,-0.379005005466573,
2.4124777376111));
#83887=CARTESIAN_POINT('Ctrl Pts',(-17.4383781101692,-0.629724805593542,
2.42965284337106));
#83888=CARTESIAN_POINT('Ctrl Pts',(-17.4208666769519,-0.694007916179942,
2.43402885887995));
#83889=CARTESIAN_POINT('Ctrl Pts',(-17.3891540940823,-0.79451452594344,
2.44082725258749));
#83890=CARTESIAN_POINT('Ctrl Pts',(-17.3766294435179,-0.831230039400335,
2.44330154751165));
#83891=CARTESIAN_POINT('Ctrl Pts',(-17.3506779834146,-0.90191585483675,
2.44805130092728));
#83892=CARTESIAN_POINT('Ctrl Pts',(-17.3373506479433,-0.935912047144666,
2.4503293330029));
#83893=CARTESIAN_POINT('Ctrl Pts',(-17.3030431418918,-1.01811664327379,
2.45582941542707));
#83894=CARTESIAN_POINT('Ctrl Pts',(-17.2812830733585,-1.06598186561352,
2.45902460782333));
#83895=CARTESIAN_POINT('Ctrl Pts',(-17.2302624345133,-1.16947943238262,
2.46594597607649));
#83896=CARTESIAN_POINT('Ctrl Pts',(-17.2003853960593,-1.22476835188526,
2.46965145327467));
#83897=CARTESIAN_POINT('Ctrl Pts',(-17.0884854260482,-1.41450535764004,
2.48250615460954));
#83898=CARTESIAN_POINT('Ctrl Pts',(-16.9959582236296,-1.54231808056167,
2.49139888008759));
#83899=CARTESIAN_POINT('Ctrl Pts',(-16.8430807155802,-1.71650301940684,
2.50494194940342));
#83900=CARTESIAN_POINT('Ctrl Pts',(-16.7916135705348,-1.77015480798999,
2.50935076384188));
#83901=CARTESIAN_POINT('Ctrl Pts',(-16.7196785540355,-1.83878845814315,
2.51544589712765));
#83902=CARTESIAN_POINT('Ctrl Pts',(-16.7012452905341,-1.8558560483638,2.51700234238244));
#83903=CARTESIAN_POINT('Ctrl Pts',(-16.6672745382308,-1.88637858348403,
2.51986776946221));
#83904=CARTESIAN_POINT('Ctrl Pts',(-16.6518225725973,-1.89992386613791,
2.52117035535816));
#83905=CARTESIAN_POINT('Ctrl Pts',(-16.6167841688128,-1.92988814335971,
2.52412462446931));
#83906=CARTESIAN_POINT('Ctrl Pts',(-16.5971119346455,-1.94619953681524,
2.52578285106987));
#83907=CARTESIAN_POINT('Ctrl Pts',(-16.5296616708102,-2.00041513491911,
2.53145715195341));
#83908=CARTESIAN_POINT('Ctrl Pts',(-16.4807585070886,-2.03687962349371,
2.5355520773628));
#83909=CARTESIAN_POINT('Ctrl Pts',(-16.341054817694,-2.13335802089972,2.54709805472074));
#83910=CARTESIAN_POINT('Ctrl Pts',(-16.2476137687162,-2.18931573646796,
2.55464623928563));
#83911=CARTESIAN_POINT('Ctrl Pts',(-16.031226118663,-2.30053662382151,2.57141026218501));
#83912=CARTESIAN_POINT('Ctrl Pts',(-15.9068558602498,-2.3523428817155,2.58056541460202));
#83913=CARTESIAN_POINT('Ctrl Pts',(-15.7306682603886,-2.40966919262813,
2.59274881752035));
#83914=CARTESIAN_POINT('Ctrl Pts',(-15.6819430288102,-2.42390924611142,
2.59604138677518));
#83915=CARTESIAN_POINT('Ctrl Pts',(-15.5977273827775,-2.44578057055992,
2.60160552763582));
#83916=CARTESIAN_POINT('Ctrl Pts',(-15.5624430135173,-2.4541350210893,2.60389947277222));
#83917=CARTESIAN_POINT('Ctrl Pts',(-15.4884699675048,-2.46997065715485,
2.60863583515606));
#83918=CARTESIAN_POINT('Ctrl Pts',(-15.4497612082208,-2.47731166420063,
2.61107325210743));
#83919=CARTESIAN_POINT('Ctrl Pts',(-15.341511634753,-2.49521978280486,2.61778781615758));
#83920=CARTESIAN_POINT('Ctrl Pts',(-15.2716746789872,-2.50378634934609,
2.62200294065662));
#83921=CARTESIAN_POINT('Ctrl Pts',(-15.1036660455121,-2.51728143140701,
2.63195348661318));
#83922=CARTESIAN_POINT('Ctrl Pts',(-15.0053862713122,-2.51940963883767,
2.63761846333319));
#83923=CARTESIAN_POINT('Ctrl Pts',(-14.7521420585386,-2.5100712673857,2.65219511752568));
#83924=CARTESIAN_POINT('Ctrl Pts',(-14.5979327152573,-2.4900245068108,2.6610443197688));
#83925=CARTESIAN_POINT('Ctrl Pts',(-14.4159570548383,-2.44901712298245,
2.67240531685714));
#83926=CARTESIAN_POINT('Ctrl Pts',(-14.385476799177,-2.44154706182681,2.67434067751713));
#83927=CARTESIAN_POINT('Ctrl Pts',(-14.3351271545209,-2.42820494099491,
2.67760374666496));
#83928=CARTESIAN_POINT('Ctrl Pts',(-14.3151767245409,-2.42265395595961,
2.67891433348294));
#83929=CARTESIAN_POINT('Ctrl Pts',(-14.2715416262838,-2.40993088612659,
2.6818227040949));
#83930=CARTESIAN_POINT('Ctrl Pts',(-14.2478920542708,-2.40265519806397,
2.68342557336208));
#83931=CARTESIAN_POINT('Ctrl Pts',(-14.1718478476851,-2.37802783629761,
2.6886572462396));
#83932=CARTESIAN_POINT('Ctrl Pts',(-14.1199182211979,-2.35930233665988,
2.69234993039285));
#83933=CARTESIAN_POINT('Ctrl Pts',(-13.9842510961954,-2.3052793935945,2.70224648429402));
#83934=CARTESIAN_POINT('Ctrl Pts',(-13.9017362945269,-2.26712913761037,
2.70852228853673));
#83935=CARTESIAN_POINT('Ctrl Pts',(-13.6793151093378,-2.14929667704887,
2.72589983870378));
#83936=CARTESIAN_POINT('Ctrl Pts',(-13.5446892707445,-2.06052645496528,
2.73692813818312));
#83937=CARTESIAN_POINT('Ctrl Pts',(-13.380064154688,-1.9277380070008,2.7508334931422));
#83938=CARTESIAN_POINT('Ctrl Pts',(-13.3416488487547,-1.89479234315044,
2.7541154614739));
#83939=CARTESIAN_POINT('Ctrl Pts',(-13.2774696440001,-1.83630288694201,
2.75966768746456));
#83940=CARTESIAN_POINT('Ctrl Pts',(-13.2512180440227,-1.81132023996692,
2.76196006325521));
#83941=CARTESIAN_POINT('Ctrl Pts',(-13.1975302524656,-1.75797193951023,
2.76669825813417));
#83942=CARTESIAN_POINT('Ctrl Pts',(-13.1702030867015,-1.72951035200085,
2.76913896422233));
#83943=CARTESIAN_POINT('Ctrl Pts',(-13.0958090604157,-1.64829002239326,
2.77587837790422));
#83944=CARTESIAN_POINT('Ctrl Pts',(-13.0502772942259,-1.5941724413033,2.78011423432863));
#83945=CARTESIAN_POINT('Ctrl Pts',(-12.9465514001448,-1.45978387913291,
2.79013376201575));
#83946=CARTESIAN_POINT('Ctrl Pts',(-12.8907015728942,-1.37785404332529,
2.79584546032297));
#83947=CARTESIAN_POINT('Ctrl Pts',(-12.7610826846142,-1.16127742400947,
2.81036259986223));
#83948=CARTESIAN_POINT('Ctrl Pts',(-12.6945349330085,-1.02280790805782,
2.81911120884958));
#83949=CARTESIAN_POINT('Ctrl Pts',(-12.6299729532501,-0.849573634692896,
2.8303670547454));
#83950=CARTESIAN_POINT('Ctrl Pts',(-12.6195028212696,-0.819778342378454,
2.83231412650748));
#83951=CARTESIAN_POINT('Ctrl Pts',(-12.6030913109298,-0.770107097637757,
2.83559060136096));
#83952=CARTESIAN_POINT('Ctrl Pts',(-12.596830275966,-0.750340893720218,
2.83690254208553));
#83953=CARTESIAN_POINT('Ctrl Pts',(-12.5836631794991,-0.706915754798818,
2.83980559072895));
#83954=CARTESIAN_POINT('Ctrl Pts',(-12.5768596178438,-0.683230626323396,
2.84140160002731));
#83955=CARTESIAN_POINT('Ctrl Pts',(-12.5561247863127,-0.606837882382302,
2.84658127016461));
#83956=CARTESIAN_POINT('Ctrl Pts',(-12.5435582261136,-0.553779008773233,
2.8502271556168));
#83957=CARTESIAN_POINT('Ctrl Pts',(-12.5150477716154,-0.413193494008731,
2.85994458156858));
#83958=CARTESIAN_POINT('Ctrl Pts',(-12.5020031031935,-0.325156460661742,
2.86608542144575));
#83959=CARTESIAN_POINT('Ctrl Pts',(-12.4781983189133,-0.0730060907433333,
2.88357178997894));
#83960=CARTESIAN_POINT('Ctrl Pts',(-12.4788076964045,0.0917477238429772,
2.89484652088946));
#83961=CARTESIAN_POINT('Ctrl Pts',(-12.5005808669617,0.305358351967433,
2.90895873790014));
#83962=CARTESIAN_POINT('Ctrl Pts',(-12.5071857424341,0.355270871363622,
2.91222298124398));
#83963=CARTESIAN_POINT('Ctrl Pts',(-12.5211060233838,0.440682757340842,
2.9177553079748));
#83964=CARTESIAN_POINT('Ctrl Pts',(-12.5276990472702,0.476282331932242,
2.92004508361057));
#83965=CARTESIAN_POINT('Ctrl Pts',(-12.5430969509735,0.550452351395346,
2.92478650809586));
#83966=CARTESIAN_POINT('Ctrl Pts',(-12.5520477533316,0.588982558360689,
2.92723285236229));
#83967=CARTESIAN_POINT('Ctrl Pts',(-12.5796722141068,0.696351346534435,
2.93401499948102));
#83968=CARTESIAN_POINT('Ctrl Pts',(-12.6003687714435,0.764632627008571,
2.93828651460151));
#83969=CARTESIAN_POINT('Ctrl Pts',(-12.6571642681183,0.926841873644022,
2.94842560670099));
#83970=CARTESIAN_POINT('Ctrl Pts',(-12.6960464175674,1.01966392427488,2.95421851629432));
#83971=CARTESIAN_POINT('Ctrl Pts',(-12.806563482134,1.24466043223553,2.96863469749068));
#83972=CARTESIAN_POINT('Ctrl Pts',(-12.8846626119122,1.37320096601879,2.97721004938609));
#83973=CARTESIAN_POINT('Ctrl Pts',(-12.9926754001392,1.51969505002037,2.98828525906537));
#83974=CARTESIAN_POINT('Ctrl Pts',(-13.0121037247994,1.54502209456754,2.99025227605026));
#83975=CARTESIAN_POINT('Ctrl Pts',(-13.0449666736673,1.58621650140448,2.99355169319552));
#83976=CARTESIAN_POINT('Ctrl Pts',(-13.0581255019231,1.60229881892036,2.99486604922211));
#83977=CARTESIAN_POINT('Ctrl Pts',(-13.0872170304606,1.63696876509306,2.99776057623168));
#83978=CARTESIAN_POINT('Ctrl Pts',(-13.1032231558638,1.65548872478016,2.99934534512335));
#83979=CARTESIAN_POINT('Ctrl Pts',(-13.1550175808511,1.71368043431677,3.00444101542798));
#83980=CARTESIAN_POINT('Ctrl Pts',(-13.1917980664131,1.75244562621497,3.00801151178949));
#83981=CARTESIAN_POINT('Ctrl Pts',(-13.2908870688405,1.85043915937773,3.01744525799798));
#83982=CARTESIAN_POINT('Ctrl Pts',(-13.3550451955013,1.90769876580335,3.0233736901728));
#83983=CARTESIAN_POINT('Ctrl Pts',(-13.5545629362486,2.06820265521756,3.04105265507564));
#83984=CARTESIAN_POINT('Ctrl Pts',(-13.6976113851656,2.16114567730894,3.05273857469013));
#83985=CARTESIAN_POINT('Ctrl Pts',(-13.893258716429,2.2617274372317,3.06718804843629));
#83986=CARTESIAN_POINT('Ctrl Pts',(-13.9382258410366,2.28318275130165,3.07041658358145));
#83987=CARTESIAN_POINT('Ctrl Pts',(-14.0168604523089,2.31787584077405,3.07590891744927));
#83988=CARTESIAN_POINT('Ctrl Pts',(-14.0502296614099,2.33174790806057,3.07819355462035));
#83989=CARTESIAN_POINT('Ctrl Pts',(-14.1209204821693,2.35936564147681,3.08294215743068));
#83990=CARTESIAN_POINT('Ctrl Pts',(-14.1582926148763,2.37295511612319,3.08540041986946));
#83991=CARTESIAN_POINT('Ctrl Pts',(-14.2648110442874,2.4088545878647,3.09227349976952));
#83992=CARTESIAN_POINT('Ctrl Pts',(-14.3346250801505,2.42906582920409,3.09662092320177));
#83993=CARTESIAN_POINT('Ctrl Pts',(-14.5060424418368,2.47074445920202,3.10701856413908));
#83994=CARTESIAN_POINT('Ctrl Pts',(-14.6082871056264,2.48900276700779,3.11298808776827));
#83995=CARTESIAN_POINT('Ctrl Pts',(-14.8538657903651,2.51734516716821,3.12720309371405));
#83996=CARTESIAN_POINT('Ctrl Pts',(-14.9974916362546,2.52158018074536,3.13541620335771));
#83997=CARTESIAN_POINT('Ctrl Pts',(-15.1731847622204,2.51174705460864,3.14611277298168));
#83998=CARTESIAN_POINT('Ctrl Pts',(-15.2056510780705,2.50929743751347,3.14811730249084));
#83999=CARTESIAN_POINT('Ctrl Pts',(-15.2586326898,2.50426485818008,3.15144737695365));
#84000=CARTESIAN_POINT('Ctrl Pts',(-15.2791808960018,2.50205742394284,3.15275358573873));
#84001=CARTESIAN_POINT('Ctrl Pts',(-15.3236139009028,2.49672994168545,3.15561346334708));
#84002=CARTESIAN_POINT('Ctrl Pts',(-15.3474845935808,2.49351974291422,3.15717141546744));
#84003=CARTESIAN_POINT('Ctrl Pts',(-15.4216621063144,2.48245837924733,3.16207232464232));
#84004=CARTESIAN_POINT('Ctrl Pts',(-15.4717768600345,2.47342361427633,3.1654689918391));
#84005=CARTESIAN_POINT('Ctrl Pts',(-15.5991938543346,2.44643968908259,3.17427004021474));
#84006=CARTESIAN_POINT('Ctrl Pts',(-15.675984552029,2.42634378855768,3.17973070112641));
#84007=CARTESIAN_POINT('Ctrl Pts',(-15.9276072548158,2.34762120089638,3.19792656820457));
#84008=CARTESIAN_POINT('Ctrl Pts',(-16.0969729444548,2.2734228541718,3.21062117286218));
#84009=CARTESIAN_POINT('Ctrl Pts',(-16.2984913392214,2.15732449941014,3.22586609457039));
#84010=CARTESIAN_POINT('Ctrl Pts',(-16.3395521488667,2.13207160133538,3.22898437688953));
#84011=CARTESIAN_POINT('Ctrl Pts',(-16.409928326851,2.0859530884859,3.23435421242933));
#84012=CARTESIAN_POINT('Ctrl Pts',(-16.4395673938858,2.065609863513,3.23662399936454));
#84013=CARTESIAN_POINT('Ctrl Pts',(-16.5016550814389,2.0210092879739,3.24140132552338));
#84014=CARTESIAN_POINT('Ctrl Pts',(-16.5339745908237,1.99658928449236,3.24390180703324));
#84015=CARTESIAN_POINT('Ctrl Pts',(-16.6263707956021,1.92320787851969,3.25110496930146));
#84016=CARTESIAN_POINT('Ctrl Pts',(-16.6847953962513,1.87223838778244,3.25572839910409));
#84017=CARTESIAN_POINT('Ctrl Pts',(-16.8248440830177,1.73818632373008,3.26711846813765));
#84018=CARTESIAN_POINT('Ctrl Pts',(-16.9032306394381,1.65198732895874,3.27377864117047));
#84019=CARTESIAN_POINT('Ctrl Pts',(-17.0504374048973,1.46566502219285,3.2874442656608));
#84020=CARTESIAN_POINT('Ctrl Pts',(-17.1185413576125,1.36537328062916,3.29443675963154));
#84021=CARTESIAN_POINT('Ctrl Pts',(-17.1959856569462,1.23149602238749,3.30382291363717));
#84022=CARTESIAN_POINT('Ctrl Pts',(-17.2122269693059,1.2020761383984,3.30588892962065));
#84023=CARTESIAN_POINT('Ctrl Pts',(-17.2375711821288,1.15391295818733,3.30929100820269));
#84024=CARTESIAN_POINT('Ctrl Pts',(-17.2470393750153,1.13536511017195,3.31060591107133));
#84025=CARTESIAN_POINT('Ctrl Pts',(-17.2667746720633,1.09549029391578,3.31344669567697));
#84026=CARTESIAN_POINT('Ctrl Pts',(-17.2769728588546,1.07413262464057,3.31497607552966));
#84027=CARTESIAN_POINT('Ctrl Pts',(-17.3070868092074,1.0087095630365,3.31967743761322));
#84028=CARTESIAN_POINT('Ctrl Pts',(-17.3260344989279,0.964213345029977,
3.32289740531873));
#84029=CARTESIAN_POINT('Ctrl Pts',(-17.3497558351271,0.903731126947436,
3.32727908574531));
#84030=CARTESIAN_POINT('Ctrl Pts',(-17.3556698601044,0.888201464170371,
3.32840458537843));
#84031=CARTESIAN_POINT('Ctrl Pts',(-17.3614291865442,0.872615864477068,
3.32953388487208));
#84032=CARTESIAN_POINT('Origin',(-15.,0.,3.));
#84033=CARTESIAN_POINT('',(-17.3578782887762,0.871321062777569,4.33113094084205));
#84034=CARTESIAN_POINT('',(-17.3614291890287,0.872615857753799,4.05617654298853));
#84035=CARTESIAN_POINT('',(-17.3614291890287,0.872615857753799,3.));
#84036=CARTESIAN_POINT('',(-17.5174991368084,-0.00208474675815134,3.11258330249198));
#84037=CARTESIAN_POINT('Ctrl Pts',(-17.3614291890287,0.872615857753799,
4.05617654298853));
#84038=CARTESIAN_POINT('Ctrl Pts',(-17.3326458200154,0.950507964736045,
4.05093731159241));
#84039=CARTESIAN_POINT('Ctrl Pts',(-17.2999869751406,1.02702172058073,4.04569808019629));
#84040=CARTESIAN_POINT('Ctrl Pts',(-17.2636144934765,1.10175118557831,4.04045884880017));
#84041=CARTESIAN_POINT('Ctrl Pts',(-17.2272502797581,1.17646366358085,4.03522080835059));
#84042=CARTESIAN_POINT('Ctrl Pts',(-17.1871743080278,1.249392242068,4.02998276790101));
#84043=CARTESIAN_POINT('Ctrl Pts',(-17.1435956684316,1.32015296851596,4.02474472745143));
#84044=CARTESIAN_POINT('Ctrl Pts',(-17.1000138112337,1.3909189195379,4.01950630025441));
#84045=CARTESIAN_POINT('Ctrl Pts',(-17.0529290156622,1.45951630881581,4.01426787305739));
#84046=CARTESIAN_POINT('Ctrl Pts',(-17.0025945105235,1.52558889495866,4.00902944586036));
#84047=CARTESIAN_POINT('Ctrl Pts',(-16.9522080313203,1.5917297058877,4.00378560960345));
#84048=CARTESIAN_POINT('Ctrl Pts',(-16.8985654223714,1.65534014057156,3.99854177334654));
#84049=CARTESIAN_POINT('Ctrl Pts',(-16.8419608225546,1.71609631960855,3.99329793708963));
#84050=CARTESIAN_POINT('Ctrl Pts',(-16.7853255760493,1.7768853930693,3.988051261731));
#84051=CARTESIAN_POINT('Ctrl Pts',(-16.7257254759839,1.83481681200538,3.98280458637238));
#84052=CARTESIAN_POINT('Ctrl Pts',(-16.6634904713541,1.88960464164179,3.97755791101376));
#84053=CARTESIAN_POINT('Ctrl Pts',(-16.6011493175152,1.94448591844372,3.97230228682573));
#84054=CARTESIAN_POINT('Ctrl Pts',(-16.5361646442827,1.99621260983414,3.9670466626377));
#84055=CARTESIAN_POINT('Ctrl Pts',(-16.468898079244,2.04454021305361,3.96179103844968));
#84056=CARTESIAN_POINT('Ctrl Pts',(-16.4212781545174,2.07875270519151,3.95807043181425));
#84057=CARTESIAN_POINT('Ctrl Pts',(-16.3725152707675,2.11126259752159,3.95434982517882));
#84058=CARTESIAN_POINT('Ctrl Pts',(-16.322745146686,2.14199708844773,3.9506292185434));
#84059=CARTESIAN_POINT('Ctrl Pts',(-16.2524270553321,2.1854205433928,3.94537253168335));
#84060=CARTESIAN_POINT('Ctrl Pts',(-16.1798394464329,2.22545734520791,3.9401158448233));
#84061=CARTESIAN_POINT('Ctrl Pts',(-16.1053419672033,2.26186325526968,3.93485915796325));
#84062=CARTESIAN_POINT('Ctrl Pts',(-16.030949644946,2.29821777654194,3.92960989118346));
#84063=CARTESIAN_POINT('Ctrl Pts',(-15.9546532181557,2.3309513856163,3.92436062440367));
#84064=CARTESIAN_POINT('Ctrl Pts',(-15.8768397418617,2.35986404631538,3.91911135762388));
#84065=CARTESIAN_POINT('Ctrl Pts',(-15.7987020560729,2.3888971714836,3.91384021979795));
#84066=CARTESIAN_POINT('Ctrl Pts',(-15.7190350506276,2.41407718762873,3.90856908197203));
#84067=CARTESIAN_POINT('Ctrl Pts',(-15.6382540307266,2.43524907191465,3.9032979441461));
#84068=CARTESIAN_POINT('Ctrl Pts',(-15.5579508403316,2.45629572194359,3.89805798573813));
#84069=CARTESIAN_POINT('Ctrl Pts',(-15.4765472288899,2.47338140804105,3.89281802733017));
#84070=CARTESIAN_POINT('Ctrl Pts',(-15.3944678088657,2.48640330553366,3.8875780689222));
#84071=CARTESIAN_POINT('Ctrl Pts',(-15.3124151379961,2.49942095927368,3.88233981818296));
#84072=CARTESIAN_POINT('Ctrl Pts',(-15.2296875510342,2.5083773825551,3.87710156744371));
#84073=CARTESIAN_POINT('Ctrl Pts',(-15.146719160104,2.51322098870321,3.87186331670446));
#84074=CARTESIAN_POINT('Ctrl Pts',(-15.0637528219605,2.51806447501184,3.86662519556892));
#84075=CARTESIAN_POINT('Ctrl Pts',(-14.9805461520855,2.51879532071795,3.86138707443338));
#84076=CARTESIAN_POINT('Ctrl Pts',(-14.8975362952314,2.51541396974834,3.85614895329784));
#84077=CARTESIAN_POINT('Ctrl Pts',(-14.813618588759,2.51199563813205,3.85085354467316));
#84078=CARTESIAN_POINT('Ctrl Pts',(-14.7299025079231,2.50437461424801,3.84555813604848));
#84079=CARTESIAN_POINT('Ctrl Pts',(-14.6468356846868,2.4926053069809,3.8402627274238));
#84080=CARTESIAN_POINT('Ctrl Pts',(-14.5645499434984,2.48094666717722,3.8350171118266));
#84081=CARTESIAN_POINT('Ctrl Pts',(-14.4829017474058,2.4652175785989,3.82977149622941));
#84082=CARTESIAN_POINT('Ctrl Pts',(-14.4023154018894,2.44552231050575,3.82452588063222));
#84083=CARTESIAN_POINT('Ctrl Pts',(-14.3205816300957,2.42554661192524,3.81920557549379));
#84084=CARTESIAN_POINT('Ctrl Pts',(-14.2399406560968,2.40149104198238,3.81388527035537));
#84085=CARTESIAN_POINT('Ctrl Pts',(-14.1608168632588,2.37351593906786,3.80856496521694));
#84086=CARTESIAN_POINT('Ctrl Pts',(-14.0816930704208,2.34554083615334,3.80324466007851));
#84087=CARTESIAN_POINT('Ctrl Pts',(-14.0040868857404,2.31364644493991,3.79792435494008));
#84088=CARTESIAN_POINT('Ctrl Pts',(-13.9283976203273,2.27804183233754,3.79260404980165));
#84089=CARTESIAN_POINT('Ctrl Pts',(-13.8536134524737,2.24286298219697,3.78734736524628));
#84090=CARTESIAN_POINT('Ctrl Pts',(-13.7804262398426,2.20393315497003,3.78209068069091));
#84091=CARTESIAN_POINT('Ctrl Pts',(-13.709237021646,2.16142017750155,3.77683399613554));
#84092=CARTESIAN_POINT('Ctrl Pts',(-13.6381482914769,2.11896720975581,3.77158473171871));
#84093=CARTESIAN_POINT('Ctrl Pts',(-13.5690523463221,2.07294137281064,3.76633546730188));
#84094=CARTESIAN_POINT('Ctrl Pts',(-13.5023281726944,2.02355759683165,3.76108620288505));
#84095=CARTESIAN_POINT('Ctrl Pts',(-13.4353259555236,1.97396803576314,3.75581506447567));
#84096=CARTESIAN_POINT('Ctrl Pts',(-13.370715748042,1.92099268608187,3.75054392606629));
#84097=CARTESIAN_POINT('Ctrl Pts',(-13.308854265586,1.86489473026583,3.74527278765691));
#84098=CARTESIAN_POINT('Ctrl Pts',(-13.2473587372881,1.80912863329598,3.7400328317369));
#84099=CARTESIAN_POINT('Ctrl Pts',(-13.1885798478623,1.75027708590773,3.73479287581688));
#84100=CARTESIAN_POINT('Ctrl Pts',(-13.1328356743309,1.68863957994255,3.72955291989687));
#84101=CARTESIAN_POINT('Ctrl Pts',(-13.0771096679175,1.6270221617422,3.72431467168713));
#84102=CARTESIAN_POINT('Ctrl Pts',(-13.0244167221458,1.56262092998962,3.71907642347739));
#84103=CARTESIAN_POINT('Ctrl Pts',(-12.9750371856855,1.49577132297807,3.71383817526764));
#84104=CARTESIAN_POINT('Ctrl Pts',(-12.9256588713244,1.42892337043423,3.70860005669984));
#84105=CARTESIAN_POINT('Ctrl Pts',(-12.8795940763273,1.35962753465171,3.70336193813203));
#84106=CARTESIAN_POINT('Ctrl Pts',(-12.8370812244144,1.28825021646396,3.69812381956423));
#84107=CARTESIAN_POINT('Ctrl Pts',(-12.7941033796426,1.2160921945182,3.6928284080222));
#84108=CARTESIAN_POINT('Ctrl Pts',(-12.7547559148056,1.14180728256877,3.68753299648018));
#84109=CARTESIAN_POINT('Ctrl Pts',(-12.719237781177,1.06580014598871,3.68223758493815));
#84110=CARTESIAN_POINT('Ctrl Pts',(-12.6840536636373,0.990507788139913,
3.67699197197707));
#84111=CARTESIAN_POINT('Ctrl Pts',(-12.6526272758111,0.913525916800646,
3.671746359016));
#84112=CARTESIAN_POINT('Ctrl Pts',(-12.6251030621893,0.835266894338282,
3.66650074605492));
#84113=CARTESIAN_POINT('Ctrl Pts',(-12.5971869019666,0.755893458281015,
3.66118043522242));
#84114=CARTESIAN_POINT('Ctrl Pts',(-12.5732850637082,0.67520668328761,3.65586012438992));
#84115=CARTESIAN_POINT('Ctrl Pts',(-12.5534950705602,0.59364962749637,3.65053981355742));
#84116=CARTESIAN_POINT('Ctrl Pts',(-12.5337050774122,0.512092571705129,
3.64521950272493));
#84117=CARTESIAN_POINT('Ctrl Pts',(-12.5180269576855,0.429665726434531,
3.63989919189243));
#84118=CARTESIAN_POINT('Ctrl Pts',(-12.5065037224533,0.346817767509945,
3.63457888105993));
#84119=CARTESIAN_POINT('Ctrl Pts',(-12.4951182891101,0.264960555109053,
3.62932219375577));
#84120=CARTESIAN_POINT('Ctrl Pts',(-12.4877470890919,0.18239196057308,3.6240655064516));
#84121=CARTESIAN_POINT('Ctrl Pts',(-12.4844686202709,0.0995395780488252,
3.61880881914744));
#84122=CARTESIAN_POINT('Ctrl Pts',(-12.4811947791833,0.0168041460788885,
3.61355955193761));
#84123=CARTESIAN_POINT('Ctrl Pts',(-12.4820022120968,-0.0662138212331839,
3.60831028472778));
#84124=CARTESIAN_POINT('Ctrl Pts',(-12.4869179159025,-0.149079470713462,
3.60306101751796));
#84125=CARTESIAN_POINT('Ctrl Pts',(-12.491854100459,-0.232290371003117,
3.5977898798013));
#84126=CARTESIAN_POINT('Ctrl Pts',(-12.5009329329858,-0.315347215037223,
3.59251874208464));
#84127=CARTESIAN_POINT('Ctrl Pts',(-12.5141288277071,-0.397807446842296,
3.58724760436798));
#84128=CARTESIAN_POINT('Ctrl Pts',(-12.5272466683683,-0.479779924233319,
3.5820076455679));
#84129=CARTESIAN_POINT('Ctrl Pts',(-12.5444329271818,-0.561162367680381,
3.57676768676782));
#84130=CARTESIAN_POINT('Ctrl Pts',(-12.5656104984621,-0.64152474995281,
3.57152772796774));
#84131=CARTESIAN_POINT('Ctrl Pts',(-12.5867811680472,-0.721860942410311,
3.56628947685162));
#84132=CARTESIAN_POINT('Ctrl Pts',(-12.6119404492328,-0.801177288403083,
3.5610512257355));
#84133=CARTESIAN_POINT('Ctrl Pts',(-12.6409605175132,-0.879055726372575,
3.55581297461938));
#84134=CARTESIAN_POINT('Ctrl Pts',(-12.6699798676975,-0.956932237254603,
3.55057485312281));
#84135=CARTESIAN_POINT('Ctrl Pts',(-12.7028596530037,-1.03337047914813,
3.54533673162624));
#84136=CARTESIAN_POINT('Ctrl Pts',(-12.7394232122634,-1.10797059380949,
3.54009861012967));
#84137=CARTESIAN_POINT('Ctrl Pts',(-12.7763866484607,-1.18338657175096,
3.53480320197871));
#84138=CARTESIAN_POINT('Ctrl Pts',(-12.8171147307613,-1.25692353151196,
3.52950779382776));
#84139=CARTESIAN_POINT('Ctrl Pts',(-12.8613771856309,-1.32819377647239,
3.5242123856768));
#84140=CARTESIAN_POINT('Ctrl Pts',(-12.9052234447086,-1.39879387387489,
3.51896676976161));
#84141=CARTESIAN_POINT('Ctrl Pts',(-12.9525375723219,-1.46716935666535,
3.51372115384643));
#84142=CARTESIAN_POINT('Ctrl Pts',(-13.0030530720546,-1.53297397791662,
3.50847553793125));
#84143=CARTESIAN_POINT('Ctrl Pts',(-13.0542878237437,-1.59971554135044,
3.5031552336624));
#84144=CARTESIAN_POINT('Ctrl Pts',(-13.1088155092712,-1.66381208411523,
3.49783492939356));
#84145=CARTESIAN_POINT('Ctrl Pts',(-13.1663182913934,-1.72493989504607,
3.49251462512471));
#84146=CARTESIAN_POINT('Ctrl Pts',(-13.2238210735156,-1.78606770597692,
3.48719432085587));
#84147=CARTESIAN_POINT('Ctrl Pts',(-13.2842985561663,-1.84422649297438,
3.48187401658703));
#84148=CARTESIAN_POINT('Ctrl Pts',(-13.3473984190091,-1.89913513592538,
3.47655371231818));
#84149=CARTESIAN_POINT('Ctrl Pts',(-13.4097437609029,-1.95338720500255,
3.47129702595348));
#84150=CARTESIAN_POINT('Ctrl Pts',(-13.4748777887539,-2.00466549675405,
3.46604033958878));
#84151=CARTESIAN_POINT('Ctrl Pts',(-13.542485224122,-2.05267068184285,3.46078365322407));
#84152=CARTESIAN_POINT('Ctrl Pts',(-13.6099972278478,-2.10060810495213,
3.45553438696354));
#84153=CARTESIAN_POINT('Ctrl Pts',(-13.6799753312175,-2.14528133384807,
3.450285120703));
#84154=CARTESIAN_POINT('Ctrl Pts',(-13.7520700424885,-2.18643021181684,
3.44503585444246));
#84155=CARTESIAN_POINT('Ctrl Pts',(-13.8244651449489,-2.22775054147983,
3.43976471648971));
#84156=CARTESIAN_POINT('Ctrl Pts',(-13.8989941790308,-2.26551677425097,
3.43449357853696));
#84157=CARTESIAN_POINT('Ctrl Pts',(-13.9752724768328,-2.29950858951725,
3.42922244058421));
#84158=CARTESIAN_POINT('Ctrl Pts',(-14.0510995691444,-2.33329933456931,
3.42398248275023));
#84159=CARTESIAN_POINT('Ctrl Pts',(-14.1286548620561,-2.36336000224891,
3.41874252491625));
#84160=CARTESIAN_POINT('Ctrl Pts',(-14.2075360388061,-2.38952026988868,
3.41350256708228));
#84161=CARTESIAN_POINT('Ctrl Pts',(-14.2863915083938,-2.41567201196792,
3.4082643169364));
#84162=CARTESIAN_POINT('Ctrl Pts',(-14.3665715662811,-2.43792573358534,
3.40302606679052));
#84163=CARTESIAN_POINT('Ctrl Pts',(-14.4476562125589,-2.45616013127712,
3.39778781664463));
#84164=CARTESIAN_POINT('Ctrl Pts',(-14.5287388523686,-2.47439407775231,
3.3925496961211));
#84165=CARTESIAN_POINT('Ctrl Pts',(-14.6107255859485,-2.48860879794204,
3.38731157559756));
#84166=CARTESIAN_POINT('Ctrl Pts',(-14.6931849831347,-2.49873383845218,
3.38207345507403));
#84167=CARTESIAN_POINT('Ctrl Pts',(-14.7765462299916,-2.5089696154552,3.37677804578256));
#84168=CARTESIAN_POINT('Ctrl Pts',(-14.8603900673708,-2.51502563260598,
3.3714826364911));
#84169=CARTESIAN_POINT('Ctrl Pts',(-14.9442659649256,-2.51688298642077,
3.36618722719963));
#84170=CARTESIAN_POINT('Ctrl Pts',(-15.0273531518726,-2.51872287497201,
3.36094161225437));
#84171=CARTESIAN_POINT('Ctrl Pts',(-15.110471334073,-2.5164428059925,3.35569599730912));
#84172=CARTESIAN_POINT('Ctrl Pts',(-15.1931849133998,-2.51007685922856,
3.35045038236386));
#84173=CARTESIAN_POINT('Ctrl Pts',(-15.2770762388958,-2.50362026870968,
3.34513007589929));
#84174=CARTESIAN_POINT('Ctrl Pts',(-15.3605508609467,-2.49296059169368,
3.33980976943472));
#84175=CARTESIAN_POINT('Ctrl Pts',(-15.4431640113846,-2.47818722234893,
3.33448946297016));
#84176=CARTESIAN_POINT('Ctrl Pts',(-15.5257771618225,-2.46341385300418,
3.32916915650559));
#84177=CARTESIAN_POINT('Ctrl Pts',(-15.6075283796236,-2.44452696351927,
3.32384885004102));
#84178=CARTESIAN_POINT('Ctrl Pts',(-15.6879897347522,-2.42166809758803,
3.31852854357646));
#84179=CARTESIAN_POINT('Ctrl Pts',(-15.7674889341989,-2.3990825776339,3.31327185725707));
#84180=CARTESIAN_POINT('Ctrl Pts',(-15.846020607845,-2.37253675293294,3.30801517093768));
#84181=CARTESIAN_POINT('Ctrl Pts',(-15.9231618085221,-2.34213119301335,
3.30275848461829));
#84182=CARTESIAN_POINT('Ctrl Pts',(-16.0001941200367,-2.31176855225924,
3.29750921840859));
#84183=CARTESIAN_POINT('Ctrl Pts',(-16.0758394317685,-2.27755716600603,
3.2922599521989));
#84184=CARTESIAN_POINT('Ctrl Pts',(-16.149688918676,-2.23964765985046,3.28701068598921));
#84185=CARTESIAN_POINT('Ctrl Pts',(-16.2238461091416,-2.20158019877307,
3.28173954802444));
#84186=CARTESIAN_POINT('Ctrl Pts',(-16.2961920223794,-2.15978385801918,
3.27646841005967));
#84187=CARTESIAN_POINT('Ctrl Pts',(-16.3663319852265,-2.11446048819715,
3.2711972720949));
#84188=CARTESIAN_POINT('Ctrl Pts',(-16.4360570513818,-2.06940521826339,
3.26595731432491));
#84189=CARTESIAN_POINT('Ctrl Pts',(-16.5036018011638,-2.02086478346146,
3.26071735655493));
#84190=CARTESIAN_POINT('Ctrl Pts',(-16.5686037995229,-1.96908312930725,
3.25547739878494));
#84191=CARTESIAN_POINT('Ctrl Pts',(-16.6335846138464,-1.91731835070199,
3.25023914870787));
#84192=CARTESIAN_POINT('Ctrl Pts',(-16.6960239622171,-1.86231473778499,
3.2450008986308));
#84193=CARTESIAN_POINT('Ctrl Pts',(-16.7555908091454,-1.80435782505698,
3.23976264855373));
#84194=CARTESIAN_POINT('Ctrl Pts',(-16.8151561820169,-1.74640234654574,
3.23452452810375));
#84195=CARTESIAN_POINT('Ctrl Pts',(-16.8718488650438,-1.68549403586695,
3.22928640765377));
#84196=CARTESIAN_POINT('Ctrl Pts',(-16.925374171573,-1.62195577912576,3.2240482872038));
#84197=CARTESIAN_POINT('Ctrl Pts',(-16.9794848801979,-1.55772260943477,
3.21875287783971));
#84198=CARTESIAN_POINT('Ctrl Pts',(-17.0303581823909,-1.49080197123738,
3.21345746847561));
#84199=CARTESIAN_POINT('Ctrl Pts',(-17.0777321367213,-1.42156090901366,
3.20816205911152));
#84200=CARTESIAN_POINT('Ctrl Pts',(-17.1246606179321,-1.35297094363052,
3.20291644425081));
#84201=CARTESIAN_POINT('Ctrl Pts',(-17.1681550948794,-1.28210444033667,
3.19767082939009));
#84202=CARTESIAN_POINT('Ctrl Pts',(-17.2080061625757,-1.20934487886118,
3.19242521452938));
#84203=CARTESIAN_POINT('Ctrl Pts',(-17.248424665409,-1.13554930168715,3.1871049079136));
#84204=CARTESIAN_POINT('Ctrl Pts',(-17.2850949728687,-1.05980677511648,
3.18178460129782));
#84205=CARTESIAN_POINT('Ctrl Pts',(-17.3178490028582,-0.982538676057817,
3.17646429468204));
#84206=CARTESIAN_POINT('Ctrl Pts',(-17.3506030328476,-0.905270576999156,
3.17114398806627));
#84207=CARTESIAN_POINT('Ctrl Pts',(-17.3794406777545,-0.826477385673053,
3.16582368145049));
#84208=CARTESIAN_POINT('Ctrl Pts',(-17.4042467347159,-0.746594862430815,
3.16050337483471));
#84209=CARTESIAN_POINT('Ctrl Pts',(-17.4339138432341,-0.651058377554528,
3.15414048878773));
#84210=CARTESIAN_POINT('Ctrl Pts',(-17.4579043977056,-0.553681574447381,
3.14777760274075));
#84211=CARTESIAN_POINT('Ctrl Pts',(-17.4760270826673,-0.455078164602668,
3.14141471669378));
#84212=CARTESIAN_POINT('Ctrl Pts',(-17.4939245284781,-0.35770025464125,
3.13513091225381));
#84213=CARTESIAN_POINT('Ctrl Pts',(-17.5060990149422,-0.259126055024416,
3.12884710781385));
#84214=CARTESIAN_POINT('Ctrl Pts',(-17.5124125335096,-0.159967219966266,
3.12256330337389));
#84215=CARTESIAN_POINT('Ctrl Pts',(-17.5157549312281,-0.107472203039025,
3.11923663641326));
#84216=CARTESIAN_POINT('Ctrl Pts',(-17.517455471861,-0.0548136774819967,
3.11590996945262));
#84217=CARTESIAN_POINT('Ctrl Pts',(-17.5174991368084,-0.00208474675815134,
3.11258330249198));
#84218=CARTESIAN_POINT('Ctrl Pts',(-17.5158506929074,-0.00208338167800927,
3.11258330249198));
#84219=CARTESIAN_POINT('Ctrl Pts',(-17.5134950467056,0.294763138477447,
3.09384312768927));
#84220=CARTESIAN_POINT('Ctrl Pts',(-17.4600137745389,0.592359407396509,
3.07510295288657));
#84221=CARTESIAN_POINT('Ctrl Pts',(-17.3591485432458,0.871797030805393,
3.05636277808387));
#84222=CARTESIAN_POINT('',(-17.5137714174146,0.00044567345935998,3.38754613095039));
#84223=CARTESIAN_POINT('Ctrl Pts',(-17.3614291865442,0.872615864477068,
3.32953388487208));
#84224=CARTESIAN_POINT('Ctrl Pts',(-17.3809756275514,0.819720268412054,
3.33336658756098));
#84225=CARTESIAN_POINT('Ctrl Pts',(-17.3987401945501,0.766180343022783,
3.33724267734535));
#84226=CARTESIAN_POINT('Ctrl Pts',(-17.4666913825592,0.535757271946432,
3.35380824336746));
#84227=CARTESIAN_POINT('Ctrl Pts',(-17.4992277272465,0.354234193360712,
3.36651646510683));
#84228=CARTESIAN_POINT('Ctrl Pts',(-17.5139281816499,0.13801801640971,3.38080025921794));
#84229=CARTESIAN_POINT('Ctrl Pts',(-17.5155142151089,0.105224851673531,
3.38294571868902));
#84230=CARTESIAN_POINT('Ctrl Pts',(-17.517147176403,0.048473737035035,3.38662289728093));
#84231=CARTESIAN_POINT('Ctrl Pts',(-17.5174943818047,0.0245295727084708,
3.38816339559275));
#84232=CARTESIAN_POINT('Ctrl Pts',(-17.5174999323689,0.000583543289451465,
3.38969342428349));
#84233=CARTESIAN_POINT('Ctrl Pts',(-17.5135466719092,0.000437363012700809,
3.38741669750803));
#84234=CARTESIAN_POINT('Ctrl Pts',(-17.512848798928,-0.445064979324669,
3.41547689838276));
#84235=CARTESIAN_POINT('Ctrl Pts',(-17.1880561406799,-1.72782200703888,
3.49621215550473));
#84236=CARTESIAN_POINT('Ctrl Pts',(-15.1454344547701,-2.96733695176447,
3.62962246887397));
#84237=CARTESIAN_POINT('Ctrl Pts',(-12.593960767586,-1.74276188959023,3.78764763761569));
#84238=CARTESIAN_POINT('Ctrl Pts',(-12.2259104525059,1.06333032658794,3.94567280635744));
#84239=CARTESIAN_POINT('Ctrl Pts',(-14.3752804154246,2.90447128399857,4.10369797509916));
#84240=CARTESIAN_POINT('Ctrl Pts',(-16.5838217551577,2.25841194757869,4.23218401992738));
#84241=CARTESIAN_POINT('Ctrl Pts',(-17.231678627738,1.21621768087466,4.30799500850834));
#84242=CARTESIAN_POINT('Ctrl Pts',(-17.3578782887762,0.871321062777582,
4.33113094084205));
#84243=CARTESIAN_POINT('Origin',(-15.,0.,3.));
#84244=CARTESIAN_POINT('',(-17.3614291890287,0.872615857753799,5.33098035402157));
#84245=CARTESIAN_POINT('',(-17.3614291890287,0.872615857753801,5.05624492860065));
#84246=CARTESIAN_POINT('',(-17.3614291890287,0.872615857753799,3.));
#84247=CARTESIAN_POINT('',(-17.517499506146,0.00157688125814863,5.38741669754798));
#84248=CARTESIAN_POINT('Ctrl Pts',(-17.3614291890287,0.872615857753799,
5.33098035402157));
#84249=CARTESIAN_POINT('Ctrl Pts',(-17.3901822610416,0.794805738991659,
5.3362220473329));
#84250=CARTESIAN_POINT('Ctrl Pts',(-17.4150567487437,0.715650742612291,
5.34146374064422));
#84251=CARTESIAN_POINT('Ctrl Pts',(-17.4359499453844,0.635573845891745,
5.34670543395554));
#84252=CARTESIAN_POINT('Ctrl Pts',(-17.4568769901463,0.555367220219244,
5.35195561909669));
#84253=CARTESIAN_POINT('Ctrl Pts',(-17.4738097794136,0.474236165619432,
5.35720580423783));
#84254=CARTESIAN_POINT('Ctrl Pts',(-17.486696953703,0.392612417587985,5.36245598937898));
#84255=CARTESIAN_POINT('Ctrl Pts',(-17.4911507150723,0.364403542031883,
5.364270434597));
#84256=CARTESIAN_POINT('Ctrl Pts',(-17.4951217376959,0.336135847325646,
5.36608487981503));
#84257=CARTESIAN_POINT('Ctrl Pts',(-17.4986093480335,0.307827185154029,
5.36789932503306));
#84258=CARTESIAN_POINT('Ctrl Pts',(-17.5111143622989,0.206324955825689,
5.37440511585805));
#84259=CARTESIAN_POINT('Ctrl Pts',(-17.5174353191478,0.104051732231825,
5.38091090668304));
#84260=CARTESIAN_POINT('Ctrl Pts',(-17.5174995061456,0.00157688188738101,
5.38741669750803));
#84261=CARTESIAN_POINT('',(-13.0865340033349,1.63598720337492,6.));
#84262=CARTESIAN_POINT('Ctrl Pts',(-17.517499506146,0.00157688125815036,
5.38741669754798));
#84263=CARTESIAN_POINT('Ctrl Pts',(-17.5175506917775,-0.0801412578474424,
5.39260471312289));
#84264=CARTESIAN_POINT('Ctrl Pts',(-17.5136187948921,-0.162011558498384,
5.39779272869779));
#84265=CARTESIAN_POINT('Ctrl Pts',(-17.5056857952746,-0.24360817999176,
5.4029807442727));
#84266=CARTESIAN_POINT('Ctrl Pts',(-17.4977635242424,-0.32509445024975,
5.4081617435776));
#84267=CARTESIAN_POINT('Ctrl Pts',(-17.4858509458476,-0.406307308451282,
5.4133427428825));
#84268=CARTESIAN_POINT('Ctrl Pts',(-17.469982063722,-0.486821173421537,
5.41852374218741));
#84269=CARTESIAN_POINT('Ctrl Pts',(-17.4541250536408,-0.567274803262042,
5.42370086541251));
#84270=CARTESIAN_POINT('Ctrl Pts',(-17.4343177025306,-0.647030014235198,
5.42887798863762));
#84271=CARTESIAN_POINT('Ctrl Pts',(-17.4106456605887,-0.725667795265136,
5.43405511186272));
#84272=CARTESIAN_POINT('Ctrl Pts',(-17.3869837657392,-0.804271867972273,
5.43923001589829));
#84273=CARTESIAN_POINT('Ctrl Pts',(-17.3594606041422,-0.88175900826378,
5.44440491993386));
#84274=CARTESIAN_POINT('Ctrl Pts',(-17.3282122408189,-0.957723348207147,
5.44957982396943));
#84275=CARTESIAN_POINT('Ctrl Pts',(-17.2969672898254,-1.03367939282381,
5.45475416290406));
#84276=CARTESIAN_POINT('Ctrl Pts',(-17.2619981263441,-1.10811252969544,
5.4599285018387));
#84277=CARTESIAN_POINT('Ctrl Pts',(-17.2234891423927,-1.18063638926725,
5.46510284077333));
#84278=CARTESIAN_POINT('Ctrl Pts',(-17.1849469545557,-1.25322278162183,
5.47028164121642));
#84279=CARTESIAN_POINT('Ctrl Pts',(-17.1428590711736,-1.32389618834014,
5.47546044165951));
#84280=CARTESIAN_POINT('Ctrl Pts',(-17.0974557680501,-1.39229506609533,
5.48063924210259));
#84281=CARTESIAN_POINT('Ctrl Pts',(-17.0520337642731,-1.4607221158913,5.48582017558327));
#84282=CARTESIAN_POINT('Ctrl Pts',(-17.0032939027791,-1.52687238923967,
5.49100110906394));
#84283=CARTESIAN_POINT('Ctrl Pts',(-16.9515082126632,-1.59041565193128,
5.49618204254462));
#84284=CARTESIAN_POINT('Ctrl Pts',(-16.8996343119159,-1.65406715285072,
5.50137180111602));
#84285=CARTESIAN_POINT('Ctrl Pts',(-16.8447045358485,-1.71510241925704,
5.50656155968743));
#84286=CARTESIAN_POINT('Ctrl Pts',(-16.7870291651781,-1.77322672346285,
5.51175131825883));
#84287=CARTESIAN_POINT('Ctrl Pts',(-16.7345255570165,-1.82613900919618,
5.51647571009749));
#84288=CARTESIAN_POINT('Ctrl Pts',(-16.6797473282794,-1.87663927633195,
5.52120010193614));
#84289=CARTESIAN_POINT('Ctrl Pts',(-16.6229512374387,-1.9245351467033,5.52592449377479));
#84290=CARTESIAN_POINT('Ctrl Pts',(-16.5596876662159,-1.97788501218986,
5.53118686122199));
#84291=CARTESIAN_POINT('Ctrl Pts',(-16.4936776611168,-2.02820751974803,
5.5364492286692));
#84292=CARTESIAN_POINT('Ctrl Pts',(-16.4252425458023,-2.07520840775929,
5.54171159611641));
#84293=CARTESIAN_POINT('Ctrl Pts',(-16.3569024508384,-2.12214403627861,
5.54696665690537));
#84294=CARTESIAN_POINT('Ctrl Pts',(-16.2861443106519,-2.16576694867464,
5.55222171769432));
#84295=CARTESIAN_POINT('Ctrl Pts',(-16.213322938943,-2.20582268005266,5.55747677848328));
#84296=CARTESIAN_POINT('Ctrl Pts',(-16.1402986576109,-2.24599002280477,
5.56274648198467));
#84297=CARTESIAN_POINT('Ctrl Pts',(-16.0651999919237,-2.28256998106267,
5.56801618548606));
#84298=CARTESIAN_POINT('Ctrl Pts',(-15.9884145738686,-2.3153494077923,5.57328588898744));
#84299=CARTESIAN_POINT('Ctrl Pts',(-15.9119748195411,-2.34798127188417,
5.57853186994617));
#84300=CARTESIAN_POINT('Ctrl Pts',(-15.8338638904551,-2.37684656188086,
5.5837778509049));
#84301=CARTESIAN_POINT('Ctrl Pts',(-15.7544877926499,-2.4017815097844,5.58902383186362));
#84302=CARTESIAN_POINT('Ctrl Pts',(-15.6751364531732,-2.42670868018759,
5.59426817653986));
#84303=CARTESIAN_POINT('Ctrl Pts',(-15.5945211671943,-2.44770780581581,
5.59951252121609));
#84304=CARTESIAN_POINT('Ctrl Pts',(-15.5130647766136,-2.4646644365914,5.60475686589233));
#84305=CARTESIAN_POINT('Ctrl Pts',(-15.4316094321405,-2.48162084960066,
5.61000114321781));
#84306=CARTESIAN_POINT('Ctrl Pts',(-15.3493134549685,-2.49453477841334,
5.6152454205433));
#84307=CARTESIAN_POINT('Ctrl Pts',(-15.266610255963,-2.50334280940812,5.62048969786879));
#84308=CARTESIAN_POINT('Ctrl Pts',(-15.1832123322294,-2.51222482976499,
5.62577802825611));
#84309=CARTESIAN_POINT('Ctrl Pts',(-15.0994007833268,-2.51693157891885,
5.63106635864342));
#84310=CARTESIAN_POINT('Ctrl Pts',(-15.0156238870574,-2.51745151773638,
5.63635468903073));
#84311=CARTESIAN_POINT('Ctrl Pts',(-14.9324247782823,-2.51796787067093,
5.64160654717688));
#84312=CARTESIAN_POINT('Ctrl Pts',(-14.8492603069933,-2.5143550643388,5.64685840532304));
#84313=CARTESIAN_POINT('Ctrl Pts',(-14.766566350805,-2.50665414076683,5.65211026346919));
#84314=CARTESIAN_POINT('Ctrl Pts',(-14.683010975526,-2.49887299703264,5.65741682997708));
#84315=CARTESIAN_POINT('Ctrl Pts',(-14.5999364514597,-2.48691813775506,
5.66272339648497));
#84316=CARTESIAN_POINT('Ctrl Pts',(-14.5177820160702,-2.47088487509529,
5.66802996299286));
#84317=CARTESIAN_POINT('Ctrl Pts',(-14.4356275806807,-2.45485161243553,
5.67333652950076));
#84318=CARTESIAN_POINT('Ctrl Pts',(-14.3543936825517,-2.43474012166965,
5.67864309600865));
#84319=CARTESIAN_POINT('Ctrl Pts',(-14.2745022103349,-2.41069683021135,
5.68394966251654));
#84320=CARTESIAN_POINT('Ctrl Pts',(-14.1961576792013,-2.38711908975994,
5.68915347781064));
#84321=CARTESIAN_POINT('Ctrl Pts',(-14.1188034503992,-2.35966984140079,
5.69435729310473));
#84322=CARTESIAN_POINT('Ctrl Pts',(-14.0428548434092,-2.32844999929455,
5.69956110839883));
#84323=CARTESIAN_POINT('Ctrl Pts',(-13.9670149075025,-2.29727482810716,
5.70475747781252));
#84324=CARTESIAN_POINT('Ctrl Pts',(-13.8925770325293,-2.26233995083739,
5.70995384722621));
#84325=CARTESIAN_POINT('Ctrl Pts',(-13.8199422128753,-2.22379627417764,
5.71515021663989));
#84326=CARTESIAN_POINT('Ctrl Pts',(-13.7460774761305,-2.18459994185093,
5.72043457558233));
#84327=CARTESIAN_POINT('Ctrl Pts',(-13.6740779020757,-2.14167158844339,
5.72571893452476));
#84328=CARTESIAN_POINT('Ctrl Pts',(-13.604344655256,-2.0952213268978,5.73100329346719));
#84329=CARTESIAN_POINT('Ctrl Pts',(-13.5358915569486,-2.04962378963984,
5.73619064324186));
#84330=CARTESIAN_POINT('Ctrl Pts',(-13.4696226850228,-2.0006328384358,5.74137799301654));
#84331=CARTESIAN_POINT('Ctrl Pts',(-13.4058915618119,-1.94849288869568,
5.74656534279121));
#84332=CARTESIAN_POINT('Ctrl Pts',(-13.3421788451239,-1.89636799777022,
5.75175119437996));
#84333=CARTESIAN_POINT('Ctrl Pts',(-13.2810027870364,-1.84109621155005,
5.75693704596871));
#84334=CARTESIAN_POINT('Ctrl Pts',(-13.2226849451813,-1.78296310839982,
5.76212289755745));
#84335=CARTESIAN_POINT('Ctrl Pts',(-13.164365513943,-1.72482842090131,5.76730889048039));
#84336=CARTESIAN_POINT('Ctrl Pts',(-13.1089047865671,-1.66383259523297,
5.77249488340333));
#84337=CARTESIAN_POINT('Ctrl Pts',(-13.0565873668425,-1.6002979682808,5.77768087632627));
#84338=CARTESIAN_POINT('Ctrl Pts',(-13.0025364217307,-1.53465813642051,
5.78303870590393));
#84339=CARTESIAN_POINT('Ctrl Pts',(-12.9518411019522,-1.46630870913287,
5.7883965354816));
#84340=CARTESIAN_POINT('Ctrl Pts',(-12.9047686108457,-1.3956402387086,5.79375436505926));
#84341=CARTESIAN_POINT('Ctrl Pts',(-12.8591296664014,-1.32712390741102,
5.7989490271791));
#84342=CARTESIAN_POINT('Ctrl Pts',(-12.8168962386622,-1.25642820507263,
5.80414368929893));
#84343=CARTESIAN_POINT('Ctrl Pts',(-12.7782654509723,-1.18393489840308,
5.80933835141876));
#84344=CARTESIAN_POINT('Ctrl Pts',(-12.7378145389097,-1.10802600426515,
5.81477776472534));
#84345=CARTESIAN_POINT('Ctrl Pts',(-12.7013143561152,-1.0301464821464,5.82021717803193));
#84346=CARTESIAN_POINT('Ctrl Pts',(-12.6689341617185,-0.950756702630547,
5.82565659133851));
#84347=CARTESIAN_POINT('Ctrl Pts',(-12.6365539673218,-0.871366923114693,
5.83109600464509));
#84348=CARTESIAN_POINT('Ctrl Pts',(-12.6082938669127,-0.790467465934306,
5.83653541795168));
#84349=CARTESIAN_POINT('Ctrl Pts',(-12.5842625352617,-0.708532816078131,
5.84197483125826));
#84350=CARTESIAN_POINT('Ctrl Pts',(-12.5604075507015,-0.627199420341229,
5.84737432897769));
#84351=CARTESIAN_POINT('Ctrl Pts',(-12.5406282933367,-0.544537571501273,
5.85277382669713));
#84352=CARTESIAN_POINT('Ctrl Pts',(-12.5250648886467,-0.460979874387583,
5.85817332441656));
#84353=CARTESIAN_POINT('Ctrl Pts',(-12.5095258535533,-0.377553014158294,
5.86356436745757));
#84354=CARTESIAN_POINT('Ctrl Pts',(-12.4981896199338,-0.293233516083529,
5.86895541049858));
#84355=CARTESIAN_POINT('Ctrl Pts',(-12.4911461993907,-0.208467880423357,
5.87434645353959));
#84356=CARTESIAN_POINT('Ctrl Pts',(-12.4841138157941,-0.123835071389566,
5.87972904888768));
#84357=CARTESIAN_POINT('Ctrl Pts',(-12.4813608876519,-0.0387579436036267,
5.88511164423578));
#84358=CARTESIAN_POINT('Ctrl Pts',(-12.4829259670636,0.0463094236313834,
5.89049423958387));
#84359=CARTESIAN_POINT('Ctrl Pts',(-12.4844896004099,0.131298192320445,
5.89587186164806));
#84360=CARTESIAN_POINT('Ctrl Pts',(-12.4903632997179,0.216276789606525,
5.90124948371226));
#84361=CARTESIAN_POINT('Ctrl Pts',(-12.5005336242105,0.300789106016054,
5.90662710577646));
#84362=CARTESIAN_POINT('Ctrl Pts',(-12.5106969819602,0.385243530901373,
5.91200104413216));
#84363=CARTESIAN_POINT('Ctrl Pts',(-12.5251510591745,0.469231883712493,
5.91737498248785));
#84364=CARTESIAN_POINT('Ctrl Pts',(-12.5438305052846,0.552302148492445,
5.92274892084355));
#84365=CARTESIAN_POINT('Ctrl Pts',(-12.562501615029,0.635335340218851,5.92812046088856));
#84366=CARTESIAN_POINT('Ctrl Pts',(-12.5853942467993,0.717450839630115,
5.93349200093357));
#84367=CARTESIAN_POINT('Ctrl Pts',(-12.6123919578486,0.798206794667818,
5.93886354097857));
#84368=CARTESIAN_POINT('Ctrl Pts',(-12.6393919087419,0.87896944956017,5.9442355266692));
#84369=CARTESIAN_POINT('Ctrl Pts',(-12.6704974923905,0.958371923001608,
5.94960751235982));
#84370=CARTESIAN_POINT('Ctrl Pts',(-12.7055425620702,1.03598808657666,5.95497949805045));
#84371=CARTESIAN_POINT('Ctrl Pts',(-12.7405870578792,1.11360297916988,5.96035139577362));
#84372=CARTESIAN_POINT('Ctrl Pts',(-12.7795707285717,1.18943122984611,5.96572329349679));
#84373=CARTESIAN_POINT('Ctrl Pts',(-12.8222800921186,1.26306858595125,5.97109519121996));
#84374=CARTESIAN_POINT('Ctrl Pts',(-12.8650202361876,1.33675901229866,5.97647096045521));
#84375=CARTESIAN_POINT('Ctrl Pts',(-12.9114912178688,1.4082550182372,5.98184672969046));
#84376=CARTESIAN_POINT('Ctrl Pts',(-12.9614347488706,1.4771790571517,5.98722249892571));
#84377=CARTESIAN_POINT('Ctrl Pts',(-13.0010044980607,1.53178686878043,5.99148166595047));
#84378=CARTESIAN_POINT('Ctrl Pts',(-13.0427531278297,1.58478068023668,5.99574083297524));
#84379=CARTESIAN_POINT('Ctrl Pts',(-13.0865340033349,1.63598720337491,6.));
#84380=CARTESIAN_POINT('',(-16.9136749826265,1.63574273981861,5.99999801496045));
#84381=CARTESIAN_POINT('Origin',(-15.,0.,6.));
#84382=CARTESIAN_POINT('',(-17.5174994024224,0.00173459013034562,5.11258330243345));
#84383=CARTESIAN_POINT('Ctrl Pts',(-16.9136749826265,1.63574273981861,5.99999801496045));
#84384=CARTESIAN_POINT('Ctrl Pts',(-16.8601965196756,1.69830783282948,5.99476349978788));
#84385=CARTESIAN_POINT('Ctrl Pts',(-16.8035449309859,1.75836640750039,5.98952898461531));
#84386=CARTESIAN_POINT('Ctrl Pts',(-16.7439851401069,1.81557761637624,5.98429446944274));
#84387=CARTESIAN_POINT('Ctrl Pts',(-16.6845090819951,1.8727083942639,5.97906731326916));
#84388=CARTESIAN_POINT('Ctrl Pts',(-16.6221332740411,1.92699943625717,5.97384015709558));
#84389=CARTESIAN_POINT('Ctrl Pts',(-16.557162345648,1.97814349310056,5.96861300092199));
#84390=CARTESIAN_POINT('Ctrl Pts',(-16.4922644958838,2.02923002363727,5.96339172419966));
#84391=CARTESIAN_POINT('Ctrl Pts',(-16.4247776903303,2.07717631690996,5.95817044747733));
#84392=CARTESIAN_POINT('Ctrl Pts',(-16.3550417101776,2.12171350886001,5.95294917075501));
#84393=CARTESIAN_POINT('Ctrl Pts',(-16.2853482658885,2.16622353509269,5.94773107878056));
#84394=CARTESIAN_POINT('Ctrl Pts',(-16.2134087614017,2.20732833758437,5.94251298680611));
#84395=CARTESIAN_POINT('Ctrl Pts',(-16.1395932525319,2.2448014319275,5.93729489483166));
#84396=CARTESIAN_POINT('Ctrl Pts',(-16.0658000387901,2.28226320795219,5.93207837892206));
#84397=CARTESIAN_POINT('Ctrl Pts',(-15.9901323607169,2.31609524368733,5.92686186301246));
#84398=CARTESIAN_POINT('Ctrl Pts',(-15.9129849843731,2.34611693406559,5.92164534710286));
#84399=CARTESIAN_POINT('Ctrl Pts',(-15.8358371547648,2.37613880083048,5.91642880054463));
#84400=CARTESIAN_POINT('Ctrl Pts',(-15.757210044023,2.40235011060392,5.9112122539864));
#84401=CARTESIAN_POINT('Ctrl Pts',(-15.6775171570007,2.4246188879842,5.90599570742817));
#84402=CARTESIAN_POINT('Ctrl Pts',(-15.5977474302612,2.44690913687365,5.90077413108652));
#84403=CARTESIAN_POINT('Ctrl Pts',(-15.5169103242883,2.46524913643255,5.89555255474486));
#84404=CARTESIAN_POINT('Ctrl Pts',(-15.4354326403361,2.47955735278093,5.89033097840321));
#84405=CARTESIAN_POINT('Ctrl Pts',(-15.3539147288184,2.49387263345271,5.88510682403904));
#84406=CARTESIAN_POINT('Ctrl Pts',(-15.271756071707,2.50415210913948,5.87988266967487));
#84407=CARTESIAN_POINT('Ctrl Pts',(-15.1893893031049,2.51036609717974,5.8746585153107));
#84408=CARTESIAN_POINT('Ctrl Pts',(-15.106883223358,2.51659059525703,5.86942552506602));
#84409=CARTESIAN_POINT('Ctrl Pts',(-15.0241687948877,2.51873585959447,5.86419253482135));
#84410=CARTESIAN_POINT('Ctrl Pts',(-14.9416790545137,2.51682437156779,5.85895954457667));
#84411=CARTESIAN_POINT('Ctrl Pts',(-14.8784767303382,2.51535981991115,5.85495011086586));
#84412=CARTESIAN_POINT('Ctrl Pts',(-14.8154063246288,2.51151487864047,5.85094067715504));
#84413=CARTESIAN_POINT('Ctrl Pts',(-14.7526593292125,2.50532010780546,5.84693124344423));
#84414=CARTESIAN_POINT('Ctrl Pts',(-14.6702583922819,2.49718497850584,5.84166595397276));
#84415=CARTESIAN_POINT('Ctrl Pts',(-14.5881137877399,2.48496590139176,5.83640066450129));
#84416=CARTESIAN_POINT('Ctrl Pts',(-14.5066608682957,2.46868846781631,5.83113537502982));
#84417=CARTESIAN_POINT('Ctrl Pts',(-14.4253200203583,2.45243343044863,5.82587733009825));
#84418=CARTESIAN_POINT('Ctrl Pts',(-14.3446694138389,2.43213121875691,5.82061928516668));
#84419=CARTESIAN_POINT('Ctrl Pts',(-14.2651391662254,2.40785917465787,5.81536124023511));
#84420=CARTESIAN_POINT('Ctrl Pts',(-14.1854437442759,2.3835367205716,5.81009227500459));
#84421=CARTESIAN_POINT('Ctrl Pts',(-14.1068738011778,2.35522798594923,5.80482330977406));
#84422=CARTESIAN_POINT('Ctrl Pts',(-14.0298517638134,2.32306234307735,5.79955434454353));
#84423=CARTESIAN_POINT('Ctrl Pts',(-13.9531201457552,2.29101798398354,5.79430524647414));
#84424=CARTESIAN_POINT('Ctrl Pts',(-13.8779252111009,2.25514591893329,5.78905614840474));
#84425=CARTESIAN_POINT('Ctrl Pts',(-13.8046676830752,2.21562336648521,5.78380705033534));
#84426=CARTESIAN_POINT('Ctrl Pts',(-13.7314323779831,2.17611280334497,5.77855954459864));
#84427=CARTESIAN_POINT('Ctrl Pts',(-13.6601337160636,2.13295417041961,5.77331203886195));
#84428=CARTESIAN_POINT('Ctrl Pts',(-13.5911487758554,2.08637112667577,5.76806453312525));
#84429=CARTESIAN_POINT('Ctrl Pts',(-13.5221641904685,2.03978832252991,5.76281705437888));
#84430=CARTESIAN_POINT('Ctrl Pts',(-13.4554936831094,1.98978140064578,5.75756957563252));
#84431=CARTESIAN_POINT('Ctrl Pts',(-13.3914850943114,1.9366171661373,5.75232209688615));
#84432=CARTESIAN_POINT('Ctrl Pts',(-13.3270228658242,1.88307614771168,5.74703742837085));
#84433=CARTESIAN_POINT('Ctrl Pts',(-13.2652608096926,1.82633317558718,5.74175275985554));
#84434=CARTESIAN_POINT('Ctrl Pts',(-13.2065187026773,1.76670062154112,5.73646809134024));
#84435=CARTESIAN_POINT('Ctrl Pts',(-13.1481049378488,1.70740138688368,5.73121296176565));
#84436=CARTESIAN_POINT('Ctrl Pts',(-13.0926777140496,1.64524517442741,5.72595783219106));
#84437=CARTESIAN_POINT('Ctrl Pts',(-13.0405117460184,1.58057332398982,5.72070270261647));
#84438=CARTESIAN_POINT('Ctrl Pts',(-12.9879059427514,1.51535619547806,5.7154032646308));
#84439=CARTESIAN_POINT('Ctrl Pts',(-12.9386169285418,1.44758119327516,5.71010382664514));
#84440=CARTESIAN_POINT('Ctrl Pts',(-12.8928815082733,1.37762763903144,5.70480438865948));
#84441=CARTESIAN_POINT('Ctrl Pts',(-12.8471460880048,1.30767408478771,5.69950495067382));
#84442=CARTESIAN_POINT('Ctrl Pts',(-12.8049644468416,1.23554241740766,5.69420551268816));
#84443=CARTESIAN_POINT('Ctrl Pts',(-12.7665250421787,1.16163499550633,5.68890607470249));
#84444=CARTESIAN_POINT('Ctrl Pts',(-12.7284410731948,1.08841096958696,5.68365563875929));
#84445=CARTESIAN_POINT('Ctrl Pts',(-12.6938903941338,1.01317465067371,5.67840520281609));
#84446=CARTESIAN_POINT('Ctrl Pts',(-12.6630904979597,0.936301356014029,
5.67315476687288));
#84447=CARTESIAN_POINT('Ctrl Pts',(-12.6323346458374,0.85953799066573,5.66791183908723));
#84448=CARTESIAN_POINT('Ctrl Pts',(-12.6053190939635,0.781142724539222,
5.66266891130157));
#84449=CARTESIAN_POINT('Ctrl Pts',(-12.5822153011964,0.701515074842446,
5.65742598351592));
#84450=CARTESIAN_POINT('Ctrl Pts',(-12.5589802614831,0.621435080114545,
5.65215327195112));
#84451=CARTESIAN_POINT('Ctrl Pts',(-12.5397017903316,0.540109073435913,
5.64688056038632));
#84452=CARTESIAN_POINT('Ctrl Pts',(-12.5245049589619,0.457963483037581,
5.64160784882152));
#84453=CARTESIAN_POINT('Ctrl Pts',(-12.5094212832647,0.376429549062439,
5.63637439788996));
#84454=CARTESIAN_POINT('Ctrl Pts',(-12.4983587538537,0.294088656736649,
5.63114094695839));
#84455=CARTESIAN_POINT('Ctrl Pts',(-12.4913891062827,0.211370844542663,
5.62590749602682));
#84456=CARTESIAN_POINT('Ctrl Pts',(-12.4844217981767,0.128680797804159,
5.62067580178037));
#84457=CARTESIAN_POINT('Ctrl Pts',(-12.4815446823358,0.0456145428386839,
5.61544410753391));
#84458=CARTESIAN_POINT('Ctrl Pts',(-12.482777705359,-0.0373921029430333,
5.61021241328745));
#84459=CARTESIAN_POINT('Ctrl Pts',(-12.4840106883402,-0.120396053103662,
5.60498088893902));
#84460=CARTESIAN_POINT('Ctrl Pts',(-12.4893535369254,-0.203339935605386,
5.59974936459058));
#84461=CARTESIAN_POINT('Ctrl Pts',(-12.4987740843549,-0.285788678756373,
5.59451784024215));
#84462=CARTESIAN_POINT('Ctrl Pts',(-12.5083234801227,-0.369365104096854,
5.58921476238537));
#84463=CARTESIAN_POINT('Ctrl Pts',(-12.5220629271967,-0.452432256540895,
5.58391168452859));
#84464=CARTESIAN_POINT('Ctrl Pts',(-12.5399048951221,-0.534544970003299,
5.5786086066718));
#84465=CARTESIAN_POINT('Ctrl Pts',(-12.5575312290757,-0.615665287861296,
5.57336962060949));
#84466=CARTESIAN_POINT('Ctrl Pts',(-12.5791612747311,-0.695853676048327,
5.56813063454718));
#84467=CARTESIAN_POINT('Ctrl Pts',(-12.6046601177278,-0.7746954875279,5.56289164848487));
#84468=CARTESIAN_POINT('Ctrl Pts',(-12.6306268756755,-0.854984080822838,
5.55755652473085));
#84469=CARTESIAN_POINT('Ctrl Pts',(-12.6606056605673,-0.933875712213862,
5.55222140097683));
#84470=CARTESIAN_POINT('Ctrl Pts',(-12.6944032211741,-1.01095486717645,
5.54688627722281));
#84471=CARTESIAN_POINT('Ctrl Pts',(-12.728200781781,-1.08803402213904,5.54155115346879));
#84472=CARTESIAN_POINT('Ctrl Pts',(-12.7658168358398,-1.1633002836756,5.53621602971477));
#84473=CARTESIAN_POINT('Ctrl Pts',(-12.8070106502183,-1.23636724388184,
5.53088090596075));
#84474=CARTESIAN_POINT('Ctrl Pts',(-12.8476084736572,-1.30837707337739,
5.52562297062609));
#84475=CARTESIAN_POINT('Ctrl Pts',(-12.8918310921115,-1.37851681878063,
5.52036503529143));
#84476=CARTESIAN_POINT('Ctrl Pts',(-12.9394814179558,-1.44639877732612,
5.51510709995677));
#84477=CARTESIAN_POINT('Ctrl Pts',(-12.9870645433647,-1.51418500311242,
5.50985657979792));
#84478=CARTESIAN_POINT('Ctrl Pts',(-13.0380655113944,-1.5797193927513,5.50460605963908));
#84479=CARTESIAN_POINT('Ctrl Pts',(-13.0922418902519,-1.64263971846856,
5.49935553948023));
#84480=CARTESIAN_POINT('Ctrl Pts',(-13.1466277812793,-1.70580337115317,
5.49408471438601));
#84481=CARTESIAN_POINT('Ctrl Pts',(-13.2042134634477,-1.76633228979876,
5.4888138892918));
#84482=CARTESIAN_POINT('Ctrl Pts',(-13.2647102936331,-1.82389031604891,
5.48354306419758));
#84483=CARTESIAN_POINT('Ctrl Pts',(-13.3248672587503,-1.88112498713392,
5.4783018500652));
#84484=CARTESIAN_POINT('Ctrl Pts',(-13.3879024126295,-1.93542173658785,
5.47306063593282));
#84485=CARTESIAN_POINT('Ctrl Pts',(-13.4534935008024,-1.98648531279234,
5.46781942180044));
#84486=CARTESIAN_POINT('Ctrl Pts',(-13.5190631933413,-2.03753223219757,
5.46257991733781));
#84487=CARTESIAN_POINT('Ctrl Pts',(-13.5871868008729,-2.08534779016708,
5.45734041287518));
#84488=CARTESIAN_POINT('Ctrl Pts',(-13.6575090010332,-2.12967701018091,
5.45210090841256));
#84489=CARTESIAN_POINT('Ctrl Pts',(-13.7278294112263,-2.17400510184766,
5.44686153731522));
#84490=CARTESIAN_POINT('Ctrl Pts',(-13.8003479123409,-2.21484678715634,
5.44162216621789));
#84491=CARTESIAN_POINT('Ctrl Pts',(-13.8746813908686,-2.25199118069822,
5.43638279512056));
#84492=CARTESIAN_POINT('Ctrl Pts',(-13.9497888020879,-2.2895223079305,5.43108887362876));
#84493=CARTESIAN_POINT('Ctrl Pts',(-14.0267487836657,-2.32327847440813,
5.42579495213697));
#84494=CARTESIAN_POINT('Ctrl Pts',(-14.1051436162847,-2.35309122273742,
5.42050103064517));
#84495=CARTESIAN_POINT('Ctrl Pts',(-14.1828412936084,-2.38263885008021,
5.4152541873252));
#84496=CARTESIAN_POINT('Ctrl Pts',(-14.2619479411992,-2.40831283198857,
5.41000734400523));
#84497=CARTESIAN_POINT('Ctrl Pts',(-14.342041527954,-2.429999361947,5.40476050068526));
#84498=CARTESIAN_POINT('Ctrl Pts',(-14.4232130941935,-2.45197777088524,
5.39944304010755));
#84499=CARTESIAN_POINT('Ctrl Pts',(-14.5053978855086,-2.46986048981595,
5.39412557952984));
#84500=CARTESIAN_POINT('Ctrl Pts',(-14.5881477291731,-2.48358288708365,
5.38880811895214));
#84501=CARTESIAN_POINT('Ctrl Pts',(-14.6708975728377,-2.49730528435134,
5.38349065837443));
#84502=CARTESIAN_POINT('Ctrl Pts',(-14.7542119789289,-2.50686736759322,
5.37817319779672));
#84503=CARTESIAN_POINT('Ctrl Pts',(-14.8376411648922,-2.51225911455456,
5.37285573721902));
#84504=CARTESIAN_POINT('Ctrl Pts',(-14.9201316740945,-2.5175901980021,5.36759810434566));
#84505=CARTESIAN_POINT('Ctrl Pts',(-15.0030356775818,-2.51886382893295,
5.3623404714723));
#84506=CARTESIAN_POINT('Ctrl Pts',(-15.0859207937919,-2.51603335971409,
5.35708283859894));
#84507=CARTESIAN_POINT('Ctrl Pts',(-15.1686892613134,-2.51320687396702,
5.35183260507552));
#84508=CARTESIAN_POINT('Ctrl Pts',(-15.2514384374779,-2.50628777674198,
5.3465823715521));
#84509=CARTESIAN_POINT('Ctrl Pts',(-15.3337325172041,-2.49528131820053,
5.34133213802868));
#84510=CARTESIAN_POINT('Ctrl Pts',(-15.4163505109539,-2.48423153763296,
5.33606123929737));
#84511=CARTESIAN_POINT('Ctrl Pts',(-15.4985093486618,-2.46906212071437,
5.33079034056606));
#84512=CARTESIAN_POINT('Ctrl Pts',(-15.5797697411648,-2.44983127933939,
5.32551944183476));
#84513=CARTESIAN_POINT('Ctrl Pts',(-15.6605687069665,-2.43070963782707,
5.32027847322488));
#84514=CARTESIAN_POINT('Ctrl Pts',(-15.7404789506386,-2.40757268016484,
5.315037504615));
#84515=CARTESIAN_POINT('Ctrl Pts',(-15.819077180215,-2.3805291056509,5.30979653600512));
#84516=CARTESIAN_POINT('Ctrl Pts',(-15.8976500117061,-2.35349426994715,
5.30455726095206));
#84517=CARTESIAN_POINT('Ctrl Pts',(-15.9749112356448,-2.32255547450268,
5.29931798589899));
#84518=CARTESIAN_POINT('Ctrl Pts',(-16.0504532418526,-2.28787111452574,
5.29407871084593));
#84519=CARTESIAN_POINT('Ctrl Pts',(-16.1259935631639,-2.25318752815229,
5.28883955265019));
#84520=CARTESIAN_POINT('Ctrl Pts',(-16.1998143245709,-2.21475873667251,
5.28360039445445));
#84521=CARTESIAN_POINT('Ctrl Pts',(-16.2715296766866,-2.1727904941124,5.27836123625871));
#84522=CARTESIAN_POINT('Ctrl Pts',(-16.3439987649109,-2.13038116078311,
5.27306701394359));
#84523=CARTESIAN_POINT('Ctrl Pts',(-16.4143175040774,-2.0843577657645,5.26777279162847));
#84524=CARTESIAN_POINT('Ctrl Pts',(-16.4821165896087,-2.03497829590555,
5.26247856931335));
#84525=CARTESIAN_POINT('Ctrl Pts',(-16.5493067545363,-1.98604231545892,
5.25723189573762));
#84526=CARTESIAN_POINT('Ctrl Pts',(-16.6140220197145,-1.93381064268263,
5.25198522216188));
#84527=CARTESIAN_POINT('Ctrl Pts',(-16.675936614042,-1.87857465002416,5.24673854858615));
#84528=CARTESIAN_POINT('Ctrl Pts',(-16.7386928733409,-1.82258778108712,
5.24142055190134));
#84529=CARTESIAN_POINT('Ctrl Pts',(-16.7985713958735,-1.76351464093587,
5.23610255521653));
#84530=CARTESIAN_POINT('Ctrl Pts',(-16.8552732205997,-1.70169548595674,
5.23078455853172));
#84531=CARTESIAN_POINT('Ctrl Pts',(-16.9119750453259,-1.63987633097761,
5.22546656184691));
#84532=CARTESIAN_POINT('Ctrl Pts',(-16.9654999110301,-1.57531157616454,
5.22014856516209));
#84533=CARTESIAN_POINT('Ctrl Pts',(-17.0155937543497,-1.50837265535626,
5.21483056847728));
#84534=CARTESIAN_POINT('Ctrl Pts',(-17.0652590935927,-1.44200633186824,
5.20955806207845));
#84535=CARTESIAN_POINT('Ctrl Pts',(-17.1117359074679,-1.37306056413704,
5.20428555567962));
#84536=CARTESIAN_POINT('Ctrl Pts',(-17.1547466573534,-1.30187291723276,
5.1990130492808));
#84537=CARTESIAN_POINT('Ctrl Pts',(-17.197696533977,-1.23078602244963,5.19374800507838));
#84538=CARTESIAN_POINT('Ctrl Pts',(-17.2371898539945,-1.15746393684039,
5.18848296087597));
#84539=CARTESIAN_POINT('Ctrl Pts',(-17.272990456247,-1.08227567459038,5.18321791667355));
#84540=CARTESIAN_POINT('Ctrl Pts',(-17.3087509397028,-1.00717166965515,
5.17795877257407));
#84541=CARTESIAN_POINT('Ctrl Pts',(-17.3408267304195,-0.930206052660622,
5.17269962847459));
#84542=CARTESIAN_POINT('Ctrl Pts',(-17.3690266765522,-0.851773946410638,
5.16744048437511));
#84543=CARTESIAN_POINT('Ctrl Pts',(-17.3972030141169,-0.773407502332921,
5.16218574315147));
#84544=CARTESIAN_POINT('Ctrl Pts',(-17.4215098023069,-0.693577437973085,
5.15693100192783));
#84545=CARTESIAN_POINT('Ctrl Pts',(-17.4418038266195,-0.612699210303533,
5.15167626070419));
#84546=CARTESIAN_POINT('Ctrl Pts',(-17.4620878926168,-0.531860669729495,
5.14642409799177));
#84547=CARTESIAN_POINT('Ctrl Pts',(-17.4783629982323,-0.449975431039625,
5.14117193527934));
#84548=CARTESIAN_POINT('Ctrl Pts',(-17.4905360163053,-0.367473266355765,
5.13591977256691));
#84549=CARTESIAN_POINT('Ctrl Pts',(-17.5027088852941,-0.284972112083975,
5.13066767417824));
#84550=CARTESIAN_POINT('Ctrl Pts',(-17.5107796928322,-0.201854497924812,
5.12541557578956));
#84551=CARTESIAN_POINT('Ctrl Pts',(-17.51470677117,-0.118558445635614,5.12016347740088));
#84552=CARTESIAN_POINT('Ctrl Pts',(-17.5165960440205,-0.0784856595574208,
5.11763675243125));
#84553=CARTESIAN_POINT('Ctrl Pts',(-17.5175270361368,-0.0383716548339769,
5.11511002746161));
#84554=CARTESIAN_POINT('Ctrl Pts',(-17.517499402423,0.00173458920130465,
5.11258330249198));
#84555=CARTESIAN_POINT('Ctrl Pts',(-17.5174994024224,0.00173459013034678,
5.11258330243345));
#84556=CARTESIAN_POINT('Ctrl Pts',(-17.5174339072919,0.0967910238682339,
5.1065946722231));
#84557=CARTESIAN_POINT('Ctrl Pts',(-17.5119806399526,0.191636187933136,
5.10060604201275));
#84558=CARTESIAN_POINT('Ctrl Pts',(-17.5012351672351,0.28570769710728,5.0946174118024));
#84559=CARTESIAN_POINT('Ctrl Pts',(-17.4899274076477,0.38470176072171,5.08831540979126));
#84560=CARTESIAN_POINT('Ctrl Pts',(-17.4727588141368,0.482838716783771,
5.08201340778011));
#84561=CARTESIAN_POINT('Ctrl Pts',(-17.4498986037571,0.579485186444757,
5.07571140576897));
#84562=CARTESIAN_POINT('Ctrl Pts',(-17.4270383933775,0.676131656105743,
5.06940940375783));
#84563=CARTESIAN_POINT('Ctrl Pts',(-17.3984867566974,0.771287459178277,
5.06310740174669));
#84564=CARTESIAN_POINT('Ctrl Pts',(-17.3644692274603,0.864344562309186,
5.05680539973555));
#84565=CARTESIAN_POINT('Ctrl Pts',(-17.363460773153,0.867103252860236,5.05661857602391));
#84566=CARTESIAN_POINT('Ctrl Pts',(-17.3624474254085,0.869860357624826,
5.05643175231228));
#84567=CARTESIAN_POINT('Ctrl Pts',(-17.3614291890287,0.872615857753804,
5.05624492860065));
#84568=CARTESIAN_POINT('Origin',(15.,0.,3.));
#84569=CARTESIAN_POINT('',(12.6385711154041,0.872616681594025,0.329758541657823));
#84570=CARTESIAN_POINT('',(12.638571011945,0.872616401618522,0.0533220355972278));
#84571=CARTESIAN_POINT('',(12.6385710119932,0.872616401748847,3.));
#84572=CARTESIAN_POINT('',(13.0865340033349,1.63598720337496,0.));
#84573=CARTESIAN_POINT('Ctrl Pts',(12.6385710118969,0.872616401488192,0.0533220355972278));
#84574=CARTESIAN_POINT('Ctrl Pts',(12.7166299025009,1.08385529951616,0.0396751487715243));
#84575=CARTESIAN_POINT('Ctrl Pts',(12.8226742739707,1.28365497417919,0.0268312150403422));
#84576=CARTESIAN_POINT('Ctrl Pts',(12.9793449478575,1.50222218660785,0.0106203823935272));
#84577=CARTESIAN_POINT('Ctrl Pts',(13.0057407311186,1.53709073746681,0.007956856747876));
#84578=CARTESIAN_POINT('Ctrl Pts',(13.0423686652523,1.58294336564474,0.00432561398330578));
#84579=CARTESIAN_POINT('Ctrl Pts',(13.051811403343,1.59455050544773,0.00339493848341432));
#84580=CARTESIAN_POINT('Ctrl Pts',(13.0696718411553,1.61610931727312,0.0016434387339535));
#84581=CARTESIAN_POINT('Ctrl Pts',(13.0780644827079,1.62608117251209,0.000823946587482173));
#84582=CARTESIAN_POINT('Ctrl Pts',(13.0865340033349,1.63598720337495,-1.60982338570648E-14));
#84583=CARTESIAN_POINT('',(16.8880578635265,1.66524585391345,0.));
#84584=CARTESIAN_POINT('Origin',(15.,0.,0.));
#84585=CARTESIAN_POINT('Ctrl Pts',(16.8880578635265,1.66524585391345,3.08840071030179E-15));
#84586=CARTESIAN_POINT('Ctrl Pts',(16.886468234627,1.66704817717801,0.000157709303802153));
#84587=CARTESIAN_POINT('Ctrl Pts',(16.8848760275067,1.66884822143744,0.000315569528701009));
#84588=CARTESIAN_POINT('Ctrl Pts',(16.8675293390091,1.68840274915651,0.0020342519324443));
#84589=CARTESIAN_POINT('Ctrl Pts',(16.8515276439882,1.70593522077278,0.00360923991232524));
#84590=CARTESIAN_POINT('Ctrl Pts',(16.746920121793,1.81734419855081,0.0138250880846664));
#84591=CARTESIAN_POINT('Ctrl Pts',(16.6514572692786,1.90450911841386,0.0227735767256802));
#84592=CARTESIAN_POINT('Ctrl Pts',(16.4655835905919,2.04970103866705,0.0390520747993906));
#84593=CARTESIAN_POINT('Ctrl Pts',(16.3773252408062,2.11002087102476,0.0463805523543274));
#84594=CARTESIAN_POINT('Ctrl Pts',(16.2216753731421,2.20245891379776,0.0585289141545112));
#84595=CARTESIAN_POINT('Ctrl Pts',(16.1562045639331,2.23752290892545,0.0634280294569529));
#84596=CARTESIAN_POINT('Ctrl Pts',(16.0528497743807,2.28712612817112,0.0708430408491615));
#84597=CARTESIAN_POINT('Ctrl Pts',(16.0160083287123,2.30372870673535,0.0734266879775329));
#84598=CARTESIAN_POINT('Ctrl Pts',(15.94497261254,2.33370512157807,0.0783006526532379));
#84599=CARTESIAN_POINT('Ctrl Pts',(15.910854614212,2.34723175800297,0.0805955447360372));
#84600=CARTESIAN_POINT('Ctrl Pts',(15.8288656360263,2.37768053869943,0.0860089184852513));
#84601=CARTESIAN_POINT('Ctrl Pts',(15.7807538665597,2.39391038027243,0.0891045683531706));
#84602=CARTESIAN_POINT('Ctrl Pts',(15.5990595642084,2.44914125421226,0.100539787843066));
#84603=CARTESIAN_POINT('Ctrl Pts',(15.462808046805,2.47850325418664,0.108591467885766));
#84604=CARTESIAN_POINT('Ctrl Pts',(15.2253859502372,2.50939468051778,0.122422059661358));
#84605=CARTESIAN_POINT('Ctrl Pts',(15.125273894214,2.516379343425,0.128200030717063));
#84606=CARTESIAN_POINT('Ctrl Pts',(14.9667513012163,2.51795474179782,0.137591990224574));
#84607=CARTESIAN_POINT('Ctrl Pts',(14.9084866311484,2.5165106479514,0.141096639099316));
#84608=CARTESIAN_POINT('Ctrl Pts',(14.8248665008829,2.51153044071001,0.146267321924945));
#84609=CARTESIAN_POINT('Ctrl Pts',(14.7994295285805,2.50962711623503,0.14785907411809));
#84610=CARTESIAN_POINT('Ctrl Pts',(14.7530459802166,2.50544681514215,0.15080313989314));
#84611=CARTESIAN_POINT('Ctrl Pts',(14.7320916688765,2.50329284006455,0.152149268741038));
#84612=CARTESIAN_POINT('Ctrl Pts',(14.6794099856822,2.49720849657372,0.155572683213796));
#84613=CARTESIAN_POINT('Ctrl Pts',(14.6477270715622,2.49293637939985,0.157666654694749));
#84614=CARTESIAN_POINT('Ctrl Pts',(14.4673669781114,2.46511000129541,0.169756462952325));
#84615=CARTESIAN_POINT('Ctrl Pts',(14.3209665486788,2.42886252867742,0.180210756369125));
#84616=CARTESIAN_POINT('Ctrl Pts',(14.0843315655944,2.34719445402622,0.197453226058448));
#84617=CARTESIAN_POINT('Ctrl Pts',(13.9919860859851,2.30904336494997,0.204280269545649));
#84618=CARTESIAN_POINT('Ctrl Pts',(13.8382433131025,2.23454018949238,0.215718581124496));
#84619=CARTESIAN_POINT('Ctrl Pts',(13.7756768419529,2.20088228388439,0.220396685642392));
#84620=CARTESIAN_POINT('Ctrl Pts',(13.6805397286415,2.14438828975984,0.227545574717692));
#84621=CARTESIAN_POINT('Ctrl Pts',(13.6469483082922,2.12335299794718,0.230077301403896));
#84622=CARTESIAN_POINT('Ctrl Pts',(13.5834506362853,2.08147104146295,0.234881828283064));
#84623=CARTESIAN_POINT('Ctrl Pts',(13.5534733149894,2.06075097106388,0.237158484389709));
#84624=CARTESIAN_POINT('Ctrl Pts',(13.482662082323,2.00949999029175,0.242563725080266));
#84625=CARTESIAN_POINT('Ctrl Pts',(13.4422844013235,1.97836478432708,0.245668417791289));
#84626=CARTESIAN_POINT('Ctrl Pts',(13.279613462669,1.84485899511896,0.258319460919686));
#84627=CARTESIAN_POINT('Ctrl Pts',(13.1662371057772,1.73221062665261,0.267457248192311));
#84628=CARTESIAN_POINT('Ctrl Pts',(13.00517208062,1.53850980009479,0.281947428721557));
#84629=CARTESIAN_POINT('Ctrl Pts',(12.9500342716112,1.46423683991663,0.287272277954226));
#84630=CARTESIAN_POINT('Ctrl Pts',(12.8683536417112,1.34052439862417,0.296051962677933));
#84631=CARTESIAN_POINT('Ctrl Pts',(12.8391588983321,1.29293721878651,0.299410139190968));
#84632=CARTESIAN_POINT('Ctrl Pts',(12.7992790396188,1.22280495597283,0.304390131558912));
#84633=CARTESIAN_POINT('Ctrl Pts',(12.7873077518174,1.20100691329311,0.305942156141811));
#84634=CARTESIAN_POINT('Ctrl Pts',(12.7660063472958,1.16082025214006,0.308817609561179));
#84635=CARTESIAN_POINT('Ctrl Pts',(12.7565759229868,1.1424883350368,0.310135114495249));
#84636=CARTESIAN_POINT('Ctrl Pts',(12.7335338142861,1.09631101818298,0.313466563384216));
#84637=CARTESIAN_POINT('Ctrl Pts',(12.720209704722,1.06832711268394,0.315496282044171));
#84638=CARTESIAN_POINT('Ctrl Pts',(12.6824463866629,0.985089492982362,0.321550207798017));
#84639=CARTESIAN_POINT('Ctrl Pts',(12.6594887716053,0.929222931042817,0.325634208538604));
#84640=CARTESIAN_POINT('Ctrl Pts',(12.6385711154041,0.872616681594026,0.329758541657824));
#84641=CARTESIAN_POINT('Origin',(15.,0.,3.));
#84642=CARTESIAN_POINT('',(12.6385710124998,0.872616403119952,1.33336808075876));
#84643=CARTESIAN_POINT('',(12.6385710119932,0.872616401748846,1.05617156246159));
#84644=CARTESIAN_POINT('',(12.6385710119932,0.872616401748847,3.));
#84645=CARTESIAN_POINT('',(12.4825021902374,-0.00332081924700182,0.112584992770917));
#84646=CARTESIAN_POINT('Ctrl Pts',(12.6385710119932,0.872616401748845,1.05617156246159));
#84647=CARTESIAN_POINT('Ctrl Pts',(12.6673553413416,0.950511052350811,1.05093096369482));
#84648=CARTESIAN_POINT('Ctrl Pts',(12.7000170560672,1.02703174438234,1.04569036492805));
#84649=CARTESIAN_POINT('Ctrl Pts',(12.736395609459,1.10177194242888,1.04044976616129));
#84650=CARTESIAN_POINT('Ctrl Pts',(12.7727641011313,1.17649146854538,1.03521061685939));
#84651=CARTESIAN_POINT('Ctrl Pts',(12.8128471878283,1.2494310646912,1.02997146755749));
#84652=CARTESIAN_POINT('Ctrl Pts',(12.85643698191,1.32020598297274,1.0247323182556));
#84653=CARTESIAN_POINT('Ctrl Pts',(12.9000278329709,1.39098261742689,1.01949304191315));
#84654=CARTESIAN_POINT('Ctrl Pts',(12.9471253173508,1.4595940780719,1.0142537655707));
#84655=CARTESIAN_POINT('Ctrl Pts',(12.9974772901859,1.52568314098265,1.00901448922826));
#84656=CARTESIAN_POINT('Ctrl Pts',(13.0478795569234,1.59183821673646,1.00376997965188));
#84657=CARTESIAN_POINT('Ctrl Pts',(13.1015425249499,1.6554654950733,0.998525470075494));
#84658=CARTESIAN_POINT('Ctrl Pts',(13.1581729809938,1.71623992555195,0.993280960499111));
#84659=CARTESIAN_POINT('Ctrl Pts',(13.2148315550953,1.77704453164743,0.988033846927755));
#84660=CARTESIAN_POINT('Ctrl Pts',(13.2744602214017,1.83499314665331,0.982786733356399));
#84661=CARTESIAN_POINT('Ctrl Pts',(13.3367297778327,1.8897985125541,0.977539619785042));
#84662=CARTESIAN_POINT('Ctrl Pts',(13.3991082283029,1.94469971947257,0.972283330310994));
#84663=CARTESIAN_POINT('Ctrl Pts',(13.4641364345657,1.99644640751603,0.967027040836946));
#84664=CARTESIAN_POINT('Ctrl Pts',(13.5314532192717,2.04479255740346,0.961770751362896));
#84665=CARTESIAN_POINT('Ctrl Pts',(13.5895954402337,2.08654963985611,0.957230838392084));
#84666=CARTESIAN_POINT('Ctrl Pts',(13.6494442930343,2.12577054198976,0.95269092542127));
#84667=CARTESIAN_POINT('Ctrl Pts',(13.7107523710849,2.16232439780365,0.948151012450456));
#84668=CARTESIAN_POINT('Ctrl Pts',(13.7817562354166,2.20465919448186,0.942893118631136));
#84669=CARTESIAN_POINT('Ctrl Pts',(13.8549771790876,2.24357028609219,0.937635224811814));
#84670=CARTESIAN_POINT('Ctrl Pts',(13.9300515382914,2.27881911069908,0.932377330992491));
#84671=CARTESIAN_POINT('Ctrl Pts',(14.0050201766223,2.31401829736638,0.927126841420507));
#84672=CARTESIAN_POINT('Ctrl Pts',(14.0818366323,2.34556526698025,0.921876351848521));
#84673=CARTESIAN_POINT('Ctrl Pts',(14.1601105462379,2.37326609453285,0.916625862276535));
#84674=CARTESIAN_POINT('Ctrl Pts',(14.2386877550134,2.40107425692501,0.911355028169543));
#84675=CARTESIAN_POINT('Ctrl Pts',(14.3187333363833,2.42500616826725,0.906084194062551));
#84676=CARTESIAN_POINT('Ctrl Pts',(14.3998297718509,2.4449134846132,0.900813359955558));
#84677=CARTESIAN_POINT('Ctrl Pts',(14.4804704191395,2.46470891540691,0.895572149639866));
#84678=CARTESIAN_POINT('Ctrl Pts',(14.56214968765,2.48052475906152,0.890330939324172));
#84679=CARTESIAN_POINT('Ctrl Pts',(14.644441218443,2.49226487413712,0.885089729008479));
#84680=CARTESIAN_POINT('Ctrl Pts',(14.7267060638877,2.50400118214949,0.879850218302962));
#84681=CARTESIAN_POINT('Ctrl Pts',(14.8095823213893,2.51166432158278,0.874610707597444));
#84682=CARTESIAN_POINT('Ctrl Pts',(14.8926349439582,2.5152095329696,0.869371196891926));
#84683=CARTESIAN_POINT('Ctrl Pts',(14.9756856116639,2.51875466091049,0.864131809512157));
#84684=CARTESIAN_POINT('Ctrl Pts',(15.0589121756989,2.51818203495976,0.858892422132388));
#84685=CARTESIAN_POINT('Ctrl Pts',(15.1418773763537,2.5134989675906,0.853653034752618));
#84686=CARTESIAN_POINT('Ctrl Pts',(15.2257062951751,2.50876714664366,0.848359102165621));
#84687=CARTESIAN_POINT('Ctrl Pts',(15.3092678970014,2.49983881025923,0.843065169578624));
#84688=CARTESIAN_POINT('Ctrl Pts',(15.3921159728945,2.48677528413827,0.837771236991626));
#84689=CARTESIAN_POINT('Ctrl Pts',(15.4742277569492,2.47382785688336,0.832524352924652));
#84690=CARTESIAN_POINT('Ctrl Pts',(15.5556382037615,2.45681860473001,0.827277468857679));
#84691=CARTESIAN_POINT('Ctrl Pts',(15.6359245095989,2.43585842529721,0.822030584790705));
#84692=CARTESIAN_POINT('Ctrl Pts',(15.7172906997503,2.41461632270512,0.816713127943696));
#84693=CARTESIAN_POINT('Ctrl Pts',(15.7975018164948,2.38931636558638,0.811395671096688));
#84694=CARTESIAN_POINT('Ctrl Pts',(15.8761368135256,2.36012510981624,0.80607821424968));
#84695=CARTESIAN_POINT('Ctrl Pts',(15.9547718105564,2.33093385404611,0.800760757402672));
#84696=CARTESIAN_POINT('Ctrl Pts',(16.0318302665396,2.29785154969403,0.795443300555665));
#84697=CARTESIAN_POINT('Ctrl Pts',(16.1069168706898,2.2610929417833,0.790125843708659));
#84698=CARTESIAN_POINT('Ctrl Pts',(16.1810520127557,2.22480012163988,0.784875767170463));
#84699=CARTESIAN_POINT('Ctrl Pts',(16.2535384001907,2.1847898098043,0.779625690632268));
#84700=CARTESIAN_POINT('Ctrl Pts',(16.3239782521661,2.14123511968937,0.774375614094074));
#84701=CARTESIAN_POINT('Ctrl Pts',(16.394318339877,2.0977421162689,0.769132973261804));
#84702=CARTESIAN_POINT('Ctrl Pts',(16.462617259154,2.05071494621835,0.763890332429535));
#84703=CARTESIAN_POINT('Ctrl Pts',(16.5284999384715,2.0003735121453,0.758647691597266));
#84704=CARTESIAN_POINT('Ctrl Pts',(16.5947615229,1.94974255392328,0.753374899237668));
#84705=CARTESIAN_POINT('Ctrl Pts',(16.6585785565492,1.89575929024698,0.74810210687807));
#84706=CARTESIAN_POINT('Ctrl Pts',(16.7195972934524,1.83869285046503,0.742829314518473));
#84707=CARTESIAN_POINT('Ctrl Pts',(16.7801594987239,1.78205337191156,0.737595972278981));
#84708=CARTESIAN_POINT('Ctrl Pts',(16.8379647960742,1.72237701765057,0.732362630039489));
#84709=CARTESIAN_POINT('Ctrl Pts',(16.8927002954464,1.65996742185417,0.727129287799997));
#84710=CARTESIAN_POINT('Ctrl Pts',(16.9474181233827,1.59757797508687,0.721897635152686));
#84711=CARTESIAN_POINT('Ctrl Pts',(16.9990678169288,1.5324573866207,0.716665982505374));
#84712=CARTESIAN_POINT('Ctrl Pts',(17.0473747558102,1.46494466082204,0.711434329858064));
#84713=CARTESIAN_POINT('Ctrl Pts',(17.095680745222,1.39743326198149,0.706202780038535));
#84714=CARTESIAN_POINT('Ctrl Pts',(17.1406438424178,1.32753019598549,0.700971230219008));
#84715=CARTESIAN_POINT('Ctrl Pts',(17.1820318275012,1.25560477610262,0.69573968039948));
#84716=CARTESIAN_POINT('Ctrl Pts',(17.2239870526643,1.18269358750389,0.690436429946769));
#84717=CARTESIAN_POINT('Ctrl Pts',(17.2622681664442,1.10770460373393,0.685133179494059));
#84718=CARTESIAN_POINT('Ctrl Pts',(17.2966815251688,1.03104811815365,0.679829929041348));
#84719=CARTESIAN_POINT('Ctrl Pts',(17.33067909875,0.955317802788523,0.674590752914191));
#84720=CARTESIAN_POINT('Ctrl Pts',(17.3609017606068,0.87796052028999,0.669351576787034));
#84721=CARTESIAN_POINT('Ctrl Pts',(17.3872121270175,0.799390086641513,0.664112400659877));
#84722=CARTESIAN_POINT('Ctrl Pts',(17.4140051510851,0.719378296349657,0.658777113044389));
#84723=CARTESIAN_POINT('Ctrl Pts',(17.4367407694382,0.638108884838129,0.653441825428902));
#84724=CARTESIAN_POINT('Ctrl Pts',(17.4553280524873,0.556030938589552,0.648106537813414));
#84725=CARTESIAN_POINT('Ctrl Pts',(17.4739153355365,0.473952992340981,0.642771250197926));
#84726=CARTESIAN_POINT('Ctrl Pts',(17.4883542636022,0.391067014483707,0.637435962582438));
#84727=CARTESIAN_POINT('Ctrl Pts',(17.4986093954603,0.307826800194012,0.63210067496695));
#84728=CARTESIAN_POINT('Ctrl Pts',(17.5087318015308,0.225663912178923,0.62683443865773));
#84729=CARTESIAN_POINT('Ctrl Pts',(17.5148155050885,0.142852881066483,0.62156820234851));
#84730=CARTESIAN_POINT('Ctrl Pts',(17.5167890973848,0.0598238187100271,
0.616301966039289));
#84731=CARTESIAN_POINT('Ctrl Pts',(17.5187598990122,-0.0230878401543792,
0.611043176213446));
#84732=CARTESIAN_POINT('Ctrl Pts',(17.5166321236805,-0.106216462358676,
0.605784386387601));
#84733=CARTESIAN_POINT('Ctrl Pts',(17.5103859807718,-0.189125560262059,
0.600525596561758));
#84734=CARTESIAN_POINT('Ctrl Pts',(17.5041280031666,-0.272191747753212,
0.595256842797735));
#84735=CARTESIAN_POINT('Ctrl Pts',(17.4937359923408,-0.355037115582707,
0.589988089033713));
#84736=CARTESIAN_POINT('Ctrl Pts',(17.4792425788845,-0.43722132272559,0.58471933526969));
#84737=CARTESIAN_POINT('Ctrl Pts',(17.4648025487528,-0.519102822282364,
0.579469987809983));
#84738=CARTESIAN_POINT('Ctrl Pts',(17.4462913438407,-0.600327566507047,
0.574220640350275));
#84739=CARTESIAN_POINT('Ctrl Pts',(17.4237930655656,-0.68046559451328,0.568971292890567));
#84740=CARTESIAN_POINT('Ctrl Pts',(17.4013024125812,-0.76057646151839,0.563723724580357));
#84741=CARTESIAN_POINT('Ctrl Pts',(17.3748274944993,-0.839600902075373,
0.558476156270146));
#84742=CARTESIAN_POINT('Ctrl Pts',(17.3445029388326,-0.917121703922343,
0.553228587959936));
#84743=CARTESIAN_POINT('Ctrl Pts',(17.314179617978,-0.994639349132042,0.547981233330045));
#84744=CARTESIAN_POINT('Ctrl Pts',(17.2800071394821,-1.07065305001508,0.542733878700155));
#84745=CARTESIAN_POINT('Ctrl Pts',(17.2421686879526,-1.14476452808648,0.537486524070264));
#84746=CARTESIAN_POINT('Ctrl Pts',(17.2040641747517,-1.21939712218985,0.532202272583175));
#84747=CARTESIAN_POINT('Ctrl Pts',(17.1622421292968,-1.2921002088261,0.526918021096086));
#84748=CARTESIAN_POINT('Ctrl Pts',(17.1169363851008,-1.36249278582903,0.521633769608997));
#84749=CARTESIAN_POINT('Ctrl Pts',(17.0718852968847,-1.43248969797793,0.516379220012112));
#84750=CARTESIAN_POINT('Ctrl Pts',(17.0233898863071,-1.50020166271471,0.511124670415227));
#84751=CARTESIAN_POINT('Ctrl Pts',(16.9717222308726,-1.56528517985794,0.505870120818341));
#84752=CARTESIAN_POINT('Ctrl Pts',(16.9196164902129,-1.63092053406481,0.500571018386151));
#84753=CARTESIAN_POINT('Ctrl Pts',(16.8642847681636,-1.69388229767138,0.495271915953962));
#84754=CARTESIAN_POINT('Ctrl Pts',(16.8060446762978,-1.75385543224533,0.489972813521772));
#84755=CARTESIAN_POINT('Ctrl Pts',(16.747804584432,-1.81382856681928,0.484673711089583));
#84756=CARTESIAN_POINT('Ctrl Pts',(16.6866565091649,-1.87081279348982,0.479374608657392));
#84757=CARTESIAN_POINT('Ctrl Pts',(16.6229513048051,-1.92453508989352,0.474075506225203));
#84758=CARTESIAN_POINT('Ctrl Pts',(16.5596871988428,-1.97788541011264,0.468813095074594));
#84759=CARTESIAN_POINT('Ctrl Pts',(16.4936766262849,-2.02820830944165,0.463550683923985));
#84760=CARTESIAN_POINT('Ctrl Pts',(16.4252409185095,-2.0752095253748,0.458288272773376));
#84761=CARTESIAN_POINT('Ctrl Pts',(16.3569002284007,-2.122145483769,0.453033168072055));
#84762=CARTESIAN_POINT('Ctrl Pts',(16.2861414678863,-2.1657686620384,0.447778063370734));
#84763=CARTESIAN_POINT('Ctrl Pts',(16.2133194579239,-2.20582459479969,0.442522958669413));
#84764=CARTESIAN_POINT('Ctrl Pts',(16.1402952985317,-2.24599172037171,0.437253266119998));
#84765=CARTESIAN_POINT('Ctrl Pts',(16.0651967800906,-2.28257147155383,0.431983573570583));
#84766=CARTESIAN_POINT('Ctrl Pts',(15.9884115291994,-2.31535070754857,0.426713881021168));
#84767=CARTESIAN_POINT('Ctrl Pts',(15.911971140087,-2.34798272379082,0.421467855979837));
#84768=CARTESIAN_POINT('Ctrl Pts',(15.8338595608591,-2.3768481031062,0.416221830938508));
#84769=CARTESIAN_POINT('Ctrl Pts',(15.7544828038383,-2.40178307694768,0.410975805897177));
#84770=CARTESIAN_POINT('Ctrl Pts',(15.6751308057191,-2.42671027316528,0.405731417176377));
#84771=CARTESIAN_POINT('Ctrl Pts',(15.5945148520336,-2.44770936130754,0.400487028455576));
#84772=CARTESIAN_POINT('Ctrl Pts',(15.5130577907785,-2.46466589080985,0.395242639734777));
#84773=CARTESIAN_POINT('Ctrl Pts',(15.4316017771907,-2.48162220222423,0.389998318465158));
#84774=CARTESIAN_POINT('Ctrl Pts',(15.3493051279597,-2.49453596581245,0.38475399719554));
#84775=CARTESIAN_POINT('Ctrl Pts',(15.2666012599693,-2.50334376748036,0.379509675925921));
#84776=CARTESIAN_POINT('Ctrl Pts',(15.1832041834066,-2.51222539451785,0.374221397722384));
#84777=CARTESIAN_POINT('Ctrl Pts',(15.0993934998851,-2.51693183770499,0.368933119518846));
#84778=CARTESIAN_POINT('Ctrl Pts',(15.0156174689234,-2.51745155756063,0.363644841315309));
#84779=CARTESIAN_POINT('Ctrl Pts',(14.9324177135075,-2.51796770238603,0.358392939929495));
#84780=CARTESIAN_POINT('Ctrl Pts',(14.8492525967313,-2.51435462410235,0.353141038543681));
#84781=CARTESIAN_POINT('Ctrl Pts',(14.7665580024741,-2.50665336330956,0.347889137157867));
#84782=CARTESIAN_POINT('Ctrl Pts',(14.6830042433276,-2.49887208939213,0.342582670545468));
#84783=CARTESIAN_POINT('Ctrl Pts',(14.5999313168712,-2.48691725938727,0.337276203933069));
#84784=CARTESIAN_POINT('Ctrl Pts',(14.5177784320523,-2.47088417563553,0.33196973732067));
#84785=CARTESIAN_POINT('Ctrl Pts',(14.4356255472334,-2.45485109188379,0.326663270708271));
#84786=CARTESIAN_POINT('Ctrl Pts',(14.3543931525699,-2.43473992962642,0.321356804095871));
#84787=CARTESIAN_POINT('Ctrl Pts',(14.2745031108374,-2.41069710121685,0.316050337483472));
#84788=CARTESIAN_POINT('Ctrl Pts',(14.1961598457118,-2.38711977368503,0.310846611065516));
#84789=CARTESIAN_POINT('Ctrl Pts',(14.1188068158017,-2.35967105367289,0.305642884647561));
#84790=CARTESIAN_POINT('Ctrl Pts',(14.0428593314625,-2.32845184417279,0.300439158229605));
#84791=CARTESIAN_POINT('Ctrl Pts',(13.9670205221751,-2.29727730697799,0.295242877946866));
#84792=CARTESIAN_POINT('Ctrl Pts',(13.892583697609,-2.26234316820717,0.290046597664128));
#84793=CARTESIAN_POINT('Ctrl Pts',(13.819949844129,-2.22380032368664,0.284850317381388));
#84794=CARTESIAN_POINT('Ctrl Pts',(13.7460845119215,-2.18460400023237,0.27956593618807));
#84795=CARTESIAN_POINT('Ctrl Pts',(13.6740843350892,-2.14167559289604,0.274281554994751));
#84796=CARTESIAN_POINT('Ctrl Pts',(13.6043504961369,-2.09522521757605,0.268997173801433));
#84797=CARTESIAN_POINT('Ctrl Pts',(13.5358982830545,-2.04962854547354,0.263809913313728));
#84798=CARTESIAN_POINT('Ctrl Pts',(13.4696302129777,-2.00063854734632,0.258622652826023));
#84799=CARTESIAN_POINT('Ctrl Pts',(13.4058998011075,-1.94849962943049,0.253435392338318));
#84800=CARTESIAN_POINT('Ctrl Pts',(13.3421877949375,-1.89637576952653,0.24824962996053));
#84801=CARTESIAN_POINT('Ctrl Pts',(13.2810123569752,-1.84110509297578,0.24306386758274));
#84802=CARTESIAN_POINT('Ctrl Pts',(13.2226950380091,-1.78297316919876,0.237878105204951));
#84803=CARTESIAN_POINT('Ctrl Pts',(13.1643761279054,-1.7248396593424,0.232692201338114));
#84804=CARTESIAN_POINT('Ctrl Pts',(13.1089158246076,-1.6638450808606,0.227506297471279));
#84805=CARTESIAN_POINT('Ctrl Pts',(13.0565987251675,-1.60031176180751,0.222320393604442));
#84806=CARTESIAN_POINT('Ctrl Pts',(13.0025461151334,-1.53467085748167,0.216962458199217));
#84807=CARTESIAN_POINT('Ctrl Pts',(12.951849267774,-1.46632022224946,0.211604522793991));
#84808=CARTESIAN_POINT('Ctrl Pts',(12.9047754075953,-1.39565044240401,0.206246587388766));
#84809=CARTESIAN_POINT('Ctrl Pts',(12.859136809538,-1.32713535430808,0.201052013171835));
#84810=CARTESIAN_POINT('Ctrl Pts',(12.8169036271155,-1.2564409598805,0.195857438954905));
#84811=CARTESIAN_POINT('Ctrl Pts',(12.778272975014,-1.18394901767212,0.190662864737975));
#84812=CARTESIAN_POINT('Ctrl Pts',(12.737820013046,-1.10803743912983,0.185223248738602));
#84813=CARTESIAN_POINT('Ctrl Pts',(12.7013180887242,-1.03015508091847,0.179783632739229));
#84814=CARTESIAN_POINT('Ctrl Pts',(12.6689364767625,-0.950762378637098,
0.174344016739856));
#84815=CARTESIAN_POINT('Ctrl Pts',(12.6365548648009,-0.871369676355722,
0.168904400740483));
#84816=CARTESIAN_POINT('Ctrl Pts',(12.6082936708023,-0.790467209915332,
0.163464784741111));
#84817=CARTESIAN_POINT('Ctrl Pts',(12.5842615716475,-0.708529530634442,
0.158025168741738));
#84818=CARTESIAN_POINT('Ctrl Pts',(12.5533439584859,-0.603115623382605,
0.151027030870664));
#84819=CARTESIAN_POINT('Ctrl Pts',(12.5293259598537,-0.495662097745632,
0.144028892999589));
#84820=CARTESIAN_POINT('Ctrl Pts',(12.5124152219306,-0.386947311552094,
0.137030755128515));
#84821=CARTESIAN_POINT('Ctrl Pts',(12.4959203534034,-0.280906042781049,
0.130204715682857));
#84822=CARTESIAN_POINT('Ctrl Pts',(12.4861873976345,-0.173664393537871,
0.1233786762372));
#84823=CARTESIAN_POINT('Ctrl Pts',(12.4833644063538,-0.0659661943196923,
0.116552636791542));
#84824=CARTESIAN_POINT('Ctrl Pts',(12.4828174506086,-0.0450996230298626,
0.115230088784667));
#84825=CARTESIAN_POINT('Ctrl Pts',(12.482529752956,-0.0242159895210024,
0.113907540777792));
#84826=CARTESIAN_POINT('Ctrl Pts',(12.4825021902374,-0.00332081924700182,
0.112584992770917));
#84827=CARTESIAN_POINT('Ctrl Pts',(12.4825022739887,-0.00338371508027381,
0.111635339680572));
#84828=CARTESIAN_POINT('Ctrl Pts',(12.4823675913716,0.0968206975641423,
0.104704442175761));
#84829=CARTESIAN_POINT('Ctrl Pts',(12.4882156443794,0.196951503677597,0.0978501008475581));
#84830=CARTESIAN_POINT('Ctrl Pts',(12.5069280030255,0.354740533776522,0.0872189342832773));
#84831=CARTESIAN_POINT('Ctrl Pts',(12.5158729127969,0.41274968462613,0.0833463613678871));
#84832=CARTESIAN_POINT('Ctrl Pts',(12.5352006621777,0.514367388117053,0.0766211706808165));
#84833=CARTESIAN_POINT('Ctrl Pts',(12.5447353595632,0.558108879288796,0.0737456119838154));
#84834=CARTESIAN_POINT('Ctrl Pts',(12.5648857957226,0.639992447749824,0.068391451530109));
#84835=CARTESIAN_POINT('Ctrl Pts',(12.575244442901,0.67818306066525,0.0659062655892474));
#84836=CARTESIAN_POINT('Ctrl Pts',(12.601878361662,0.76794651483863,0.0600832067456229));
#84837=CARTESIAN_POINT('Ctrl Pts',(12.6189236479036,0.819271141012264,0.0567683063242814));
#84838=CARTESIAN_POINT('Ctrl Pts',(12.6379294358328,0.870878727335478,0.053434295920754));
#84839=CARTESIAN_POINT('Ctrl Pts',(12.6382499872001,0.871747661199217,0.0533781597321072));
#84840=CARTESIAN_POINT('Ctrl Pts',(12.6385710118969,0.872616401488192,0.0533220355972284));
#84841=CARTESIAN_POINT('Ctrl Pts',(12.6385711154041,0.872616681594026,0.329758541657824));
#84842=CARTESIAN_POINT('Ctrl Pts',(12.604742168923,0.781070584618255,0.336428593169256));
#84843=CARTESIAN_POINT('Ctrl Pts',(12.5762486803767,0.687589650928952,0.343201336130416));
#84844=CARTESIAN_POINT('Ctrl Pts',(12.5304438206718,0.49848259594701,0.356611734577644));
#84845=CARTESIAN_POINT('Ctrl Pts',(12.5130895120278,0.403077620634501,0.363235540803975));
#84846=CARTESIAN_POINT('Ctrl Pts',(12.4927843145818,0.237758076097962,0.374383878584141));
#84847=CARTESIAN_POINT('Ctrl Pts',(12.4871647804762,0.168285650935039,0.3789716204258));
#84848=CARTESIAN_POINT('Ctrl Pts',(12.4829009703236,0.0595741557933482,
0.38599867336799));
#84849=CARTESIAN_POINT('Ctrl Pts',(12.4822790884716,0.0204523564103614,
0.38849716768747));
#84850=CARTESIAN_POINT('Ctrl Pts',(12.4828363091139,-0.0546826133986007,
0.393241445280683));
#84851=CARTESIAN_POINT('Ctrl Pts',(12.4838761255024,-0.0906868069017626,
0.395490986094705));
#84852=CARTESIAN_POINT('Ctrl Pts',(12.4882219026152,-0.176955756085008,
0.400830467162363));
#84853=CARTESIAN_POINT('Ctrl Pts',(12.4922644730078,-0.227168665815338,
0.403896861580725));
#84854=CARTESIAN_POINT('Ctrl Pts',(12.5189888492276,-0.468374960492772,
0.418480888627921));
#84855=CARTESIAN_POINT('Ctrl Pts',(12.5619977837427,-0.656460864068143,
0.429352037481086));
#84856=CARTESIAN_POINT('Ctrl Pts',(12.6498945262017,-0.905518527406008,
0.444598126285946));
#84857=CARTESIAN_POINT('Ctrl Pts',(12.676668289437,-0.972156439160653,0.448774464393134));
#84858=CARTESIAN_POINT('Ctrl Pts',(12.7259518357056,-1.08110880071214,0.455901856630064));
#84859=CARTESIAN_POINT('Ctrl Pts',(12.7468880072878,-1.1240894107314,0.458794903871633));
#84860=CARTESIAN_POINT('Ctrl Pts',(12.7799106944797,-1.18724928464749,0.463207055548019));
#84861=CARTESIAN_POINT('Ctrl Pts',(12.7910780798627,-1.2078995154515,0.464676033404665));
#84862=CARTESIAN_POINT('Ctrl Pts',(12.8126780674132,-1.24653976343559,0.467480689348058));
#84863=CARTESIAN_POINT('Ctrl Pts',(12.8230477174689,-1.26456208154167,0.468812668418927));
#84864=CARTESIAN_POINT('Ctrl Pts',(12.8507318399904,-1.3113270067994,0.472328119495822));
#84865=CARTESIAN_POINT('Ctrl Pts',(12.8683995321564,-1.33985496631125,0.474531859886888));
#84866=CARTESIAN_POINT('Ctrl Pts',(12.9436419208379,-1.45609228270961,0.48373188173108));
#84867=CARTESIAN_POINT('Ctrl Pts',(13.006098355106,-1.54050839470345,0.4909391503102));
#84868=CARTESIAN_POINT('Ctrl Pts',(13.1555257252679,-1.71810983826825,0.50695408024129));
#84869=CARTESIAN_POINT('Ctrl Pts',(13.2446846144548,-1.80910448024971,0.515748458881631));
#84870=CARTESIAN_POINT('Ctrl Pts',(13.3836516743425,-1.93094317007374,0.528209632277172));
#84871=CARTESIAN_POINT('Ctrl Pts',(13.4282514391545,-1.96741726238998,0.53204723959394));
#84872=CARTESIAN_POINT('Ctrl Pts',(13.5134539725199,-2.03234829268834,0.539080395520705));
#84873=CARTESIAN_POINT('Ctrl Pts',(13.5537211831046,-2.06119790882775,0.542289072819348));
#84874=CARTESIAN_POINT('Ctrl Pts',(13.624823211575,-2.10902892129922,0.547763646985517));
#84875=CARTESIAN_POINT('Ctrl Pts',(13.6552634107837,-2.12856710377433,0.550049780318644));
#84876=CARTESIAN_POINT('Ctrl Pts',(13.7202664698996,-2.16833835850625,0.554816634319897));
#84877=CARTESIAN_POINT('Ctrl Pts',(13.7549125412612,-2.18841646998942,0.557291296145527));
#84878=CARTESIAN_POINT('Ctrl Pts',(13.8549960906644,-2.24327030812304,0.564267624468481));
#84879=CARTESIAN_POINT('Ctrl Pts',(13.9215116740373,-2.27599648112374,0.568698738434944));
#84880=CARTESIAN_POINT('Ctrl Pts',(14.1464490997509,-2.37458792540086,0.58316495893481));
#84881=CARTESIAN_POINT('Ctrl Pts',(14.310136774633,-2.42720093368182,0.592842289956259));
#84882=CARTESIAN_POINT('Ctrl Pts',(14.5335679095169,-2.47456774938233,0.606150784004289));
#84883=CARTESIAN_POINT('Ctrl Pts',(14.5896170245296,-2.48447772146856,0.609500801979481));
#84884=CARTESIAN_POINT('Ctrl Pts',(14.6866139918683,-2.49825586132311,0.615388697619319));
#84885=CARTESIAN_POINT('Ctrl Pts',(14.727410285451,-2.50303566919724,0.617892425804689));
#84886=CARTESIAN_POINT('Ctrl Pts',(14.7906346651955,-2.50887930949783,0.621839634283163));
#84887=CARTESIAN_POINT('Ctrl Pts',(14.8129923700133,-2.51064479590491,0.623248372960291));
#84888=CARTESIAN_POINT('Ctrl Pts',(14.8572913051837,-2.51354791076056,0.626070380636404));
#84889=CARTESIAN_POINT('Ctrl Pts',(14.8792296089908,-2.51469745299752,0.627482973797375));
#84890=CARTESIAN_POINT('Ctrl Pts',(14.9399378175018,-2.51708230927156,0.631428394811506));
#84891=CARTESIAN_POINT('Ctrl Pts',(14.9787243377328,-2.51770883705923,0.633990149912726));
#84892=CARTESIAN_POINT('Ctrl Pts',(15.1890960338925,-2.51624582516177,0.648054101231258));
#84893=CARTESIAN_POINT('Ctrl Pts',(15.3601070881016,-2.49751301650272,0.660062135035727));
#84894=CARTESIAN_POINT('Ctrl Pts',(15.6445667064522,-2.43651022208841,0.679997661878572));
#84895=CARTESIAN_POINT('Ctrl Pts',(15.7593388291444,-2.40321855648549,0.688038260867876));
#84896=CARTESIAN_POINT('Ctrl Pts',(15.913635752508,-2.34629695965286,0.698772286654597));
#84897=CARTESIAN_POINT('Ctrl Pts',(15.955517676486,-2.32955491627493,0.701679248999914));
#84898=CARTESIAN_POINT('Ctrl Pts',(16.0297211530866,-2.2975543236392,0.706821549061802));
#84899=CARTESIAN_POINT('Ctrl Pts',(16.0622094237457,-2.28271611763231,0.709070190562082));
#84900=CARTESIAN_POINT('Ctrl Pts',(16.1326496108087,-2.24871466226891,0.713944562186402));
#84901=CARTESIAN_POINT('Ctrl Pts',(16.1704543985394,-2.22927109277121,0.716559855515438));
#84902=CARTESIAN_POINT('Ctrl Pts',(16.2886176974978,-2.16466284075243,0.724750554638095));
#84903=CARTESIAN_POINT('Ctrl Pts',(16.3670003538676,-2.1160371565166,0.730205426687023));
#84904=CARTESIAN_POINT('Ctrl Pts',(16.5803356849875,-1.96687891523612,0.745378402081721));
#84905=CARTESIAN_POINT('Ctrl Pts',(16.7081202263537,-1.85698519904677,0.754846285568924));
#84906=CARTESIAN_POINT('Ctrl Pts',(16.8681809198738,-1.68873220738179,0.768504443517352));
#84907=CARTESIAN_POINT('Ctrl Pts',(16.9105750877766,-1.64061510531638,0.772334718895013));
#84908=CARTESIAN_POINT('Ctrl Pts',(16.9677402874505,-1.57050920308719,0.777897461646474));
#84909=CARTESIAN_POINT('Ctrl Pts',(16.9840746337631,-1.54982215423057,0.779536892014463));
#84910=CARTESIAN_POINT('Ctrl Pts',(17.0124992674903,-1.51263714107904,0.782487836536395));
#84911=CARTESIAN_POINT('Ctrl Pts',(17.0247183876664,-1.4962418862075,0.78379079890158));
#84912=CARTESIAN_POINT('Ctrl Pts',(17.0536569346944,-1.45640934590498,0.786960386040286));
#84913=CARTESIAN_POINT('Ctrl Pts',(17.0701758237359,-1.43283176793966,0.788839073800151));
#84914=CARTESIAN_POINT('Ctrl Pts',(17.1400700340562,-1.32933876117576,0.797078676662087));
#84915=CARTESIAN_POINT('Ctrl Pts',(17.1892454009603,-1.24669264688285,0.803638388431322));
#84916=CARTESIAN_POINT('Ctrl Pts',(17.3291773256558,-0.977590286218625,
0.824520220170332));
#84917=CARTESIAN_POINT('Ctrl Pts',(17.4017334207819,-0.78259477751762,0.838889351353303));
#84918=CARTESIAN_POINT('Ctrl Pts',(17.4595214645086,-0.538908338722196,
0.855299759443689));
#84919=CARTESIAN_POINT('Ctrl Pts',(17.4683970460975,-0.49667336057499,0.858094428341065));
#84920=CARTESIAN_POINT('Ctrl Pts',(17.4827343463794,-0.418515013268738,
0.863178213122588));
#84921=CARTESIAN_POINT('Ctrl Pts',(17.4885125151201,-0.382662169774976,
0.865476654945772));
#84922=CARTESIAN_POINT('Ctrl Pts',(17.4989021121014,-0.307937768290788,
0.87020202856891));
#84923=CARTESIAN_POINT('Ctrl Pts',(17.503386770235,-0.269058318328164,0.872624413454042));
#84924=CARTESIAN_POINT('Ctrl Pts',(17.5132544936217,-0.161543007546097,
0.879235048842481));
#84925=CARTESIAN_POINT('Ctrl Pts',(17.5167320423799,-0.0927647962934042,
0.883364556165057));
#84926=CARTESIAN_POINT('Ctrl Pts',(17.5182872636156,0.0708697245805634,
0.893035066516843));
#84927=CARTESIAN_POINT('Ctrl Pts',(17.5138330712852,0.165644200625899,0.898511535287157));
#84928=CARTESIAN_POINT('Ctrl Pts',(17.4872184688903,0.422022059387645,0.913342091520537));
#84929=CARTESIAN_POINT('Ctrl Pts',(17.4546991609139,0.582063159446605,0.92260663816126));
#84930=CARTESIAN_POINT('Ctrl Pts',(17.3980007661231,0.767027995927043,0.934405086453369));
#84931=CARTESIAN_POINT('Ctrl Pts',(17.3885164728805,0.796070651897628,0.936291480449378));
#84932=CARTESIAN_POINT('Ctrl Pts',(17.3717559080207,0.84439598649696,0.939498500985057));
#84933=CARTESIAN_POINT('Ctrl Pts',(17.3647673133553,0.863774386117301,0.940803399676279));
#84934=CARTESIAN_POINT('Ctrl Pts',(17.3487097700778,0.906643567050734,0.943734874261015));
#84935=CARTESIAN_POINT('Ctrl Pts',(17.3395255523565,0.93008613090563,0.945367338722355));
#84936=CARTESIAN_POINT('Ctrl Pts',(17.3079519772803,1.00724918952326,0.950829516955083));
#84937=CARTESIAN_POINT('Ctrl Pts',(17.2840526845121,1.06032803391536,0.954730699734162));
#84938=CARTESIAN_POINT('Ctrl Pts',(17.2142483121891,1.20202517595606,0.96545559880941));
#84939=CARTESIAN_POINT('Ctrl Pts',(17.1648787842151,1.28882069783537,0.972363724015122));
#84940=CARTESIAN_POINT('Ctrl Pts',(17.0305639094022,1.49536326497365,0.989362248487098));
#84941=CARTESIAN_POINT('Ctrl Pts',(16.9400430366759,1.61106945679474,0.999377773926579));
#84942=CARTESIAN_POINT('Ctrl Pts',(16.8050749328937,1.75559736152835,1.01238635017896));
#84943=CARTESIAN_POINT('Ctrl Pts',(16.7690661105209,1.79187703851152,1.01570290337216));
#84944=CARTESIAN_POINT('Ctrl Pts',(16.7056223531936,1.85201977267528,1.02129471491247));
#84945=CARTESIAN_POINT('Ctrl Pts',(16.6787306126256,1.87642974904936,1.02359290561397));
#84946=CARTESIAN_POINT('Ctrl Pts',(16.6216645485043,1.92602019926174,1.0283274503941));
#84947=CARTESIAN_POINT('Ctrl Pts',(16.5914097477963,1.95109328277504,1.03075903632243));
#84948=CARTESIAN_POINT('Ctrl Pts',(16.5059489382381,2.01860621182805,1.0374259745998));
#84949=CARTESIAN_POINT('Ctrl Pts',(16.4495491216316,2.05948095589878,1.04160094114627));
#84950=CARTESIAN_POINT('Ctrl Pts',(16.3110329376754,2.15135487339746,1.0514192140602));
#84951=CARTESIAN_POINT('Ctrl Pts',(16.2275336786949,2.20006765597637,1.05699500218606));
#84952=CARTESIAN_POINT('Ctrl Pts',(16.0000357708245,2.31579438345819,1.07168057128616));
#84953=CARTESIAN_POINT('Ctrl Pts',(15.8521664388527,2.37418947103169,1.08071639932309));
#84954=CARTESIAN_POINT('Ctrl Pts',(15.6700216152687,2.42689901065738,1.09227268039386));
#84955=CARTESIAN_POINT('Ctrl Pts',(15.6400801596817,2.43496713687307,1.09418616400736));
#84956=CARTESIAN_POINT('Ctrl Pts',(15.5899448238934,2.44748822419849,1.09742476684954));
#84957=CARTESIAN_POINT('Ctrl Pts',(15.5698318104211,2.45224900477874,1.09873341705746));
#84958=CARTESIAN_POINT('Ctrl Pts',(15.5253055319549,2.46221104603106,1.10165409204259));
#84959=CARTESIAN_POINT('Ctrl Pts',(15.5008714141582,2.46729747813692,1.10327157696218));
#84960=CARTESIAN_POINT('Ctrl Pts',(15.4207418694658,2.48273872448992,1.10861519571037));
#84961=CARTESIAN_POINT('Ctrl Pts',(15.3647749790611,2.49157651365271,1.1124088341832));
#84962=CARTESIAN_POINT('Ctrl Pts',(15.2142058107458,2.51017151938912,1.12270002374003));
#84963=CARTESIAN_POINT('Ctrl Pts',(15.1192682563172,2.51646956154645,1.12927538876171));
#84964=CARTESIAN_POINT('Ctrl Pts',(14.8705182732249,2.5188613990881,1.1464457567487));
#84965=CARTESIAN_POINT('Ctrl Pts',(14.716998759213,2.50626229996753,1.15696458653425));
#84966=CARTESIAN_POINT('Ctrl Pts',(14.5153664340098,2.47093796125292,1.1704286939267));
#84967=CARTESIAN_POINT('Ctrl Pts',(14.4654379187208,2.46061945326338,1.17373625719563));
#84968=CARTESIAN_POINT('Ctrl Pts',(14.3805596809748,2.44037220863774,1.17931731211773));
#84969=CARTESIAN_POINT('Ctrl Pts',(14.3454500820677,2.43119054226346,1.18161353750134));
#84970=CARTESIAN_POINT('Ctrl Pts',(14.272739853022,2.41048634656855,1.18634756077971));
#84971=CARTESIAN_POINT('Ctrl Pts',(14.2351858625547,2.3988354157261,1.18878051434161));
#84972=CARTESIAN_POINT('Ctrl Pts',(14.1317285603217,2.36406155072531,1.19546108494195));
#84973=CARTESIAN_POINT('Ctrl Pts',(14.0664893755381,2.33906850123898,1.199647805954));
#84974=CARTESIAN_POINT('Ctrl Pts',(13.9132596500795,2.27293234662019,1.20950408643882));
#84975=CARTESIAN_POINT('Ctrl Pts',(13.8264452391703,2.22934894972906,1.21510525830822));
#84976=CARTESIAN_POINT('Ctrl Pts',(13.6056551196452,2.10202570493024,1.22976722969446));
#84977=CARTESIAN_POINT('Ctrl Pts',(13.4766802936759,2.01052109272765,1.23875710519235));
#84978=CARTESIAN_POINT('Ctrl Pts',(13.3335645145612,1.88726430825271,1.25026581253358));
#84979=CARTESIAN_POINT('Ctrl Pts',(13.3103747679457,1.86653158702515,1.25218494018752));
#84980=CARTESIAN_POINT('Ctrl Pts',(13.2724220956371,1.83131325492163,1.25542943166501));
#84981=CARTESIAN_POINT('Ctrl Pts',(13.2574431634037,1.81706612314704,1.25673814211022));
#84982=CARTESIAN_POINT('Ctrl Pts',(13.2248234303855,1.78526567765905,1.25965390177186));
#84983=CARTESIAN_POINT('Ctrl Pts',(13.2072657831394,1.76763381495852,1.26126629411108));
#84984=CARTESIAN_POINT('Ctrl Pts',(13.1509453397864,1.70937304890351,1.26657172570376));
#84985=CARTESIAN_POINT('Ctrl Pts',(13.1132820308486,1.667709116314,1.27033104088656));
#84986=CARTESIAN_POINT('Ctrl Pts',(13.0166235947319,1.55331539048402,1.28048698565395));
#84987=CARTESIAN_POINT('Ctrl Pts',(12.9602391315948,1.47849418169828,1.28695941847178));
#84988=CARTESIAN_POINT('Ctrl Pts',(12.8213037578709,1.27100558895069,1.30419718779099));
#84989=CARTESIAN_POINT('Ctrl Pts',(12.7466933591226,1.13348771233836,1.31488680045159));
#84990=CARTESIAN_POINT('Ctrl Pts',(12.6687435921548,0.951221329104753,1.32792405305236));
#84991=CARTESIAN_POINT('Ctrl Pts',(12.6531633245514,0.912105356742518,1.33066211520459));
#84992=CARTESIAN_POINT('Ctrl Pts',(12.6385710124998,0.872616403119952,1.33336808075876));
#84993=CARTESIAN_POINT('Origin',(15.,0.,3.));
#84994=CARTESIAN_POINT('',(12.6385710877721,0.872616606817863,2.33071866803842));
#84995=CARTESIAN_POINT('',(12.6385710119932,0.872616401748851,2.05625948175199));
#84996=CARTESIAN_POINT('',(12.6385710119932,0.872616401748847,3.));
#84997=CARTESIAN_POINT('',(12.482500077493,0.000624641887345871,1.11258330254392));
#84998=CARTESIAN_POINT('Ctrl Pts',(12.6385710119932,0.872616401748851,2.05625948175199));
#84999=CARTESIAN_POINT('Ctrl Pts',(12.6420817776151,0.882117052542451,2.05561538571552));
#85000=CARTESIAN_POINT('Ctrl Pts',(12.6456495005229,0.891595491259146,2.05497128967904));
#85001=CARTESIAN_POINT('Ctrl Pts',(12.6492738991091,0.901051079900762,2.05432719364257));
#85002=CARTESIAN_POINT('Ctrl Pts',(12.6788539027848,0.978221495935984,2.04907049720776));
#85003=CARTESIAN_POINT('Ctrl Pts',(12.7122922497419,1.05407532159594,2.04381380077295));
#85004=CARTESIAN_POINT('Ctrl Pts',(12.7494510805673,1.12820025316438,2.03855710433814));
#85005=CARTESIAN_POINT('Ctrl Pts',(12.7865574588937,1.20222055178812,2.03330782812775));
#85006=CARTESIAN_POINT('Ctrl Pts',(12.8273736844179,1.27451639508405,2.02805855191736));
#85007=CARTESIAN_POINT('Ctrl Pts',(12.8717132992482,1.34469400586271,2.02280927570697));
#85008=CARTESIAN_POINT('Ctrl Pts',(12.9162375548247,1.41516385297371,2.01753814025671));
#85009=CARTESIAN_POINT('Ctrl Pts',(12.9643144432659,1.48349734572078,2.01226700480646));
#85010=CARTESIAN_POINT('Ctrl Pts',(13.0157077482685,1.54931936982614,2.0069958693562));
#85011=CARTESIAN_POINT('Ctrl Pts',(13.0667971665732,1.61475219075496,2.0017559019335));
#85012=CARTESIAN_POINT('Ctrl Pts',(13.1211636033577,1.67770279408537,1.9965159345108));
#85013=CARTESIAN_POINT('Ctrl Pts',(13.1785317860396,1.73783192384415,1.9912759670881));
#85014=CARTESIAN_POINT('Ctrl Pts',(13.2358812709124,1.79794145592808,1.98603770750948));
#85015=CARTESIAN_POINT('Ctrl Pts',(13.296230240507,1.85523100749621,1.98079944793085));
#85016=CARTESIAN_POINT('Ctrl Pts',(13.3592647967259,1.90939630321658,1.97556118835222));
#85017=CARTESIAN_POINT('Ctrl Pts',(13.4222977911159,1.96356025686479,1.97032305856375));
#85018=CARTESIAN_POINT('Ctrl Pts',(13.4880158893933,2.01459980887977,1.96508492877528));
#85019=CARTESIAN_POINT('Ctrl Pts',(13.5560712294798,2.06225021655082,1.95984679898681));
#85020=CARTESIAN_POINT('Ctrl Pts',(13.6248706131303,2.11042158229963,1.95455140114631));
#85021=CARTESIAN_POINT('Ctrl Pts',(13.6960582729743,2.15512895369361,1.94925600330581));
#85022=CARTESIAN_POINT('Ctrl Pts',(13.7692452867183,2.19614414047322,1.94396060546531));
#85023=CARTESIAN_POINT('Ctrl Pts',(13.8417443785649,2.23677380468988,1.93871498175746));
#85024=CARTESIAN_POINT('Ctrl Pts',(13.9162049509551,2.27378025032919,1.93346935804961));
#85025=CARTESIAN_POINT('Ctrl Pts',(13.9922263886963,2.30698907634168,1.92822373434176));
#85026=CARTESIAN_POINT('Ctrl Pts',(14.0693298429917,2.34067056507355,1.92290344943494));
#85027=CARTESIAN_POINT('Ctrl Pts',(14.1480384835152,2.37044530737412,1.91758316452811));
#85028=CARTESIAN_POINT('Ctrl Pts',(14.2279176382871,2.39618343970819,1.91226287962129));
#85029=CARTESIAN_POINT('Ctrl Pts',(14.307796793059,2.42192157204227,1.90694259471447));
#85030=CARTESIAN_POINT('Ctrl Pts',(14.3888459741961,2.4436230300173,1.90162230980764));
#85031=CARTESIAN_POINT('Ctrl Pts',(14.470620895541,2.46121189940286,1.89630202490082));
#85032=CARTESIAN_POINT('Ctrl Pts',(14.5514188943887,2.47859064370457,1.8910452986735));
#85033=CARTESIAN_POINT('Ctrl Pts',(14.6332217605528,2.49201832667614,1.88578857244619));
#85034=CARTESIAN_POINT('Ctrl Pts',(14.7156088295062,2.50138519867396,1.88053184621887));
#85035=CARTESIAN_POINT('Ctrl Pts',(14.7978796096309,2.51073884939097,1.8752825398275));
#85036=CARTESIAN_POINT('Ctrl Pts',(14.8807325002353,2.51604302277806,1.87003323343612));
#85037=CARTESIAN_POINT('Ctrl Pts',(14.9637358079743,2.5172387964547,1.86478392704475));
#85038=CARTESIAN_POINT('Ctrl Pts',(15.0470841635553,2.51843954100706,1.85951279909118));
#85039=CARTESIAN_POINT('Ctrl Pts',(15.1305837295089,2.51549755083754,1.85424167113761));
#85040=CARTESIAN_POINT('Ctrl Pts',(15.2137912737799,2.50840577683427,1.84897054318404));
#85041=CARTESIAN_POINT('Ctrl Pts',(15.2965074202738,2.50135588463405,1.8437305448664));
#85042=CARTESIAN_POINT('Ctrl Pts',(15.3789345204306,2.49020512748366,1.83849054654875));
#85043=CARTESIAN_POINT('Ctrl Pts',(15.4606380334944,2.47499875799936,1.83325054823111));
#85044=CARTESIAN_POINT('Ctrl Pts',(15.5423149204558,2.45979734407129,1.82801225756014));
#85045=CARTESIAN_POINT('Ctrl Pts',(15.6232682356974,2.44054302711176,1.82277396688917));
#85046=CARTESIAN_POINT('Ctrl Pts',(15.7030716394199,2.4173325215707,1.81753567621821));
#85047=CARTESIAN_POINT('Ctrl Pts',(15.7828730681785,2.39412259044014,1.81229751518376));
#85048=CARTESIAN_POINT('Ctrl Pts',(15.8615241995453,2.36695679520795,1.80705935414931));
#85049=CARTESIAN_POINT('Ctrl Pts',(15.9386132538092,2.33598189414508,1.80182119311486));
#85050=CARTESIAN_POINT('Ctrl Pts',(16.0165441155426,2.30466874917293,1.79652583170188));
#85051=CARTESIAN_POINT('Ctrl Pts',(16.0928781233521,2.26946296278871,1.7912304702889));
#85052=CARTESIAN_POINT('Ctrl Pts',(16.1672117001879,2.23056564506508,1.78593510887592));
#85053=CARTESIAN_POINT('Ctrl Pts',(16.2408475238947,2.19203344800837,1.78068945386955));
#85054=CARTESIAN_POINT('Ctrl Pts',(16.3125199438519,2.14987902217788,1.77544379886318));
#85055=CARTESIAN_POINT('Ctrl Pts',(16.381864034631,2.10434266216157,1.7701981438568));
#85056=CARTESIAN_POINT('Ctrl Pts',(16.4521937541547,2.05815906681708,1.76487792924052));
#85057=CARTESIAN_POINT('Ctrl Pts',(16.5201280402855,2.00849693418549,1.75955771462424));
#85058=CARTESIAN_POINT('Ctrl Pts',(16.5853206882403,1.95564939737096,1.75423750000795));
#85059=CARTESIAN_POINT('Ctrl Pts',(16.650513336195,1.90280186055643,1.74891728539167));
#85060=CARTESIAN_POINT('Ctrl Pts',(16.7129640255581,1.84676929299895,1.74359707077538));
#85061=CARTESIAN_POINT('Ctrl Pts',(16.7723664851078,1.78788234860868,1.7382768561591));
#85062=CARTESIAN_POINT('Ctrl Pts',(16.831058252292,1.72969992894892,1.73302029271045));
#85063=CARTESIAN_POINT('Ctrl Pts',(16.8869896882907,1.66851764379647,1.7277637292618));
#85064=CARTESIAN_POINT('Ctrl Pts',(16.9398390787621,1.60462786916696,1.72250716581314));
#85065=CARTESIAN_POINT('Ctrl Pts',(16.992613866375,1.54082828214002,1.71725802259501));
#85066=CARTESIAN_POINT('Ctrl Pts',(17.0423149588083,1.47432914965126,1.71200887937687));
#85067=CARTESIAN_POINT('Ctrl Pts',(17.0886571892918,1.40545985201274,1.70675973615873));
#85068=CARTESIAN_POINT('Ctrl Pts',(17.135193872432,1.33630157782419,1.70148856746117));
#85069=CARTESIAN_POINT('Ctrl Pts',(17.1783431060488,1.26475353319337,1.69621739876362));
#85070=CARTESIAN_POINT('Ctrl Pts',(17.2178568409913,1.19118314413369,1.69094623006606));
#85071=CARTESIAN_POINT('Ctrl Pts',(17.2571356951225,1.11805007826535,1.68570639468543));
#85072=CARTESIAN_POINT('Ctrl Pts',(17.2928219309709,1.04291905461402,1.6804665593048));
#85073=CARTESIAN_POINT('Ctrl Pts',(17.3247160849578,0.966178748647717,1.67522672392417));
#85074=CARTESIAN_POINT('Ctrl Pts',(17.3565998474769,0.889463445521055,1.6699885957398));
#85075=CARTESIAN_POINT('Ctrl Pts',(17.384693805145,0.811140326937861,1.66475046755544));
#85076=CARTESIAN_POINT('Ctrl Pts',(17.4088460792308,0.731619311236649,1.65951233937107));
#85077=CARTESIAN_POINT('Ctrl Pts',(17.4329977586653,0.652100253416509,1.65427434015428));
#85078=CARTESIAN_POINT('Ctrl Pts',(17.4532078144991,0.571383798667101,1.64903634093748));
#85079=CARTESIAN_POINT('Ctrl Pts',(17.4693742390353,0.489895006699017,1.64379834172068));
#85080=CARTESIAN_POINT('Ctrl Pts',(17.4857183007786,0.407510813192036,1.63850278719541));
#85081=CARTESIAN_POINT('Ctrl Pts',(17.4979292111129,0.324337673737048,1.63320723267013));
#85082=CARTESIAN_POINT('Ctrl Pts',(17.5059549605607,0.24082355707255,1.62791167814485));
#85083=CARTESIAN_POINT('Ctrl Pts',(17.5139048438455,0.158098886382231,1.62266618167404));
#85084=CARTESIAN_POINT('Ctrl Pts',(17.5177483960051,0.0750401264698005,
1.61742068520324));
#85085=CARTESIAN_POINT('Ctrl Pts',(17.51748755506,-0.0079158144197794,1.61217518873243));
#85086=CARTESIAN_POINT('Ctrl Pts',(17.5172229802862,-0.0920592348065238,
1.60685460517992));
#85087=CARTESIAN_POINT('Ctrl Pts',(17.5127356050044,-0.176096377978873,
1.6015340216274));
#85088=CARTESIAN_POINT('Ctrl Pts',(17.5040818716157,-0.259577021798146,
1.59621343807489));
#85089=CARTESIAN_POINT('Ctrl Pts',(17.495428138227,-0.343057665617419,1.59089285452238));
#85090=CARTESIAN_POINT('Ctrl Pts',(17.4826081846109,-0.425981337446218,
1.58557227096986));
#85091=CARTESIAN_POINT('Ctrl Pts',(17.4657317156099,-0.507910776254469,
1.58025168741735));
#85092=CARTESIAN_POINT('Ctrl Pts',(17.4490575726161,-0.588857992050123,
1.57499489045586));
#85093=CARTESIAN_POINT('Ctrl Pts',(17.4283625190827,-0.669131702942927,
1.56973809349437));
#85094=CARTESIAN_POINT('Ctrl Pts',(17.4037157334411,-0.748302694641591,
1.56448129653287));
#85095=CARTESIAN_POINT('Ctrl Pts',(17.3791037409477,-0.827361922960895,
1.5592319204383));
#85096=CARTESIAN_POINT('Ctrl Pts',(17.3505512331481,-0.905321087546031,
1.55398254434372));
#85097=CARTESIAN_POINT('Ctrl Pts',(17.3181783479629,-0.981761374793338,
1.54873316824914));
#85098=CARTESIAN_POINT('Ctrl Pts',(17.2856714273941,-1.05851815231214,1.54346205785025));
#85099=CARTESIAN_POINT('Ctrl Pts',(17.2493125166114,-1.13374298531113,1.53819094745135));
#85100=CARTESIAN_POINT('Ctrl Pts',(17.2092738670235,-1.20702743568121,1.53291983705245));
#85101=CARTESIAN_POINT('Ctrl Pts',(17.1694710338388,-1.27988026121685,1.52767977201368));
#85102=CARTESIAN_POINT('Ctrl Pts',(17.1260319110588,-1.35081508884042,1.52243970697491));
#85103=CARTESIAN_POINT('Ctrl Pts',(17.0791731159878,-1.41945250140804,1.51719964193614));
#85104=CARTESIAN_POINT('Ctrl Pts',(17.0323296026566,-1.48806752972353,1.5119612858041));
#85105=CARTESIAN_POINT('Ctrl Pts',(16.9820688918041,-1.5543862505504,1.50672292967207));
#85106=CARTESIAN_POINT('Ctrl Pts',(16.9286513878899,-1.6180575002114,1.50148457354004));
#85107=CARTESIAN_POINT('Ctrl Pts',(16.8752352196017,-1.68172715786649,1.4962463483854));
#85108=CARTESIAN_POINT('Ctrl Pts',(16.8186627123708,-1.74274912342548,1.49100812323075));
#85109=CARTESIAN_POINT('Ctrl Pts',(16.7592341963719,-1.80080573419667,1.48576989807611));
#85110=CARTESIAN_POINT('Ctrl Pts',(16.6991583655349,-1.85949471656551,1.4804746164594));
#85111=CARTESIAN_POINT('Ctrl Pts',(16.636164261308,-1.91515300259753,1.4751793348427));
#85112=CARTESIAN_POINT('Ctrl Pts',(16.570598616877,-1.9674923721997,1.46988405322599));
#85113=CARTESIAN_POINT('Ctrl Pts',(16.5056466986456,-2.01934181994305,1.46463833801087));
#85114=CARTESIAN_POINT('Ctrl Pts',(16.4381715953401,-2.06793400260606,1.45939262279575));
#85115=CARTESIAN_POINT('Ctrl Pts',(16.3685403427349,-2.11303184554967,1.45414690758064));
#85116=CARTESIAN_POINT('Ctrl Pts',(16.2979221787682,-2.15876887810874,1.44882684276313));
#85117=CARTESIAN_POINT('Ctrl Pts',(16.2250866927709,-2.20091149619349,1.44350677794563));
#85118=CARTESIAN_POINT('Ctrl Pts',(16.1504416786233,-2.23926108216223,1.43818671312813));
#85119=CARTESIAN_POINT('Ctrl Pts',(16.0757966644757,-2.27761066813096,1.43286664831063));
#85120=CARTESIAN_POINT('Ctrl Pts',(15.9993425929955,-2.31216707934187,1.42754658349313));
#85121=CARTESIAN_POINT('Ctrl Pts',(15.9215054922675,-2.34278336124381,1.42222651867563));
#85122=CARTESIAN_POINT('Ctrl Pts',(15.8445922768582,-2.37303624403277,1.41696960022064));
#85123=CARTESIAN_POINT('Ctrl Pts',(15.766046716246,-2.39955299249558,1.41171268176565));
#85124=CARTESIAN_POINT('Ctrl Pts',(15.6862661453634,-2.42215710219798,1.40645576331066));
#85125=CARTESIAN_POINT('Ctrl Pts',(15.6065981524194,-2.44472931536157,1.4012062628653));
#85126=CARTESIAN_POINT('Ctrl Pts',(15.5256990507878,-2.46339973191149,1.39595676241995));
#85127=CARTESIAN_POINT('Ctrl Pts',(15.4439852976864,-2.47804021465317,1.39070726197459));
#85128=CARTESIAN_POINT('Ctrl Pts',(15.3619356422798,-2.4927408803104,1.38543618230623));
#85129=CARTESIAN_POINT('Ctrl Pts',(15.2790650606302,-2.50337823301684,1.38016510263786));
#85130=CARTESIAN_POINT('Ctrl Pts',(15.1958097448168,-2.5098734617177,1.3748940229695));
#85131=CARTESIAN_POINT('Ctrl Pts',(15.1130422387048,-2.51633063356245,1.36965382762095));
#85132=CARTESIAN_POINT('Ctrl Pts',(15.0298949590122,-2.51869405103694,1.3644136322724));
#85133=CARTESIAN_POINT('Ctrl Pts',(14.9468040613674,-2.51693790986448,1.35917343692384));
#85134=CARTESIAN_POINT('Ctrl Pts',(14.8637402302972,-2.51518234074898,1.35393494855093));
#85135=CARTESIAN_POINT('Ctrl Pts',(14.7807332054025,-2.50930988796735,1.34869646017802));
#85136=CARTESIAN_POINT('Ctrl Pts',(14.6982193938658,-2.49934685783331,1.3434579718051));
#85137=CARTESIAN_POINT('Ctrl Pts',(14.6157076180462,-2.48938407349948,1.33821961267214));
#85138=CARTESIAN_POINT('Ctrl Pts',(14.5336894890003,-2.47533096881395,1.33298125353917));
#85139=CARTESIAN_POINT('Ctrl Pts',(14.4525951610934,-2.45726559255235,1.3277428944062));
#85140=CARTESIAN_POINT('Ctrl Pts',(14.3706219911186,-2.43900443672095,1.32244776570018));
#85141=CARTESIAN_POINT('Ctrl Pts',(14.2895932397855,-2.41664360508234,1.31715263699415));
#85142=CARTESIAN_POINT('Ctrl Pts',(14.2099396769268,-2.39031607447748,1.31185750828812));
#85143=CARTESIAN_POINT('Ctrl Pts',(14.1310273731703,-2.3642335488793,1.30661165625234));
#85144=CARTESIAN_POINT('Ctrl Pts',(14.0534651817788,-2.33425807187132,1.30136580421656));
#85145=CARTESIAN_POINT('Ctrl Pts',(13.977652192976,-2.300567584635,1.29611995218078));
#85146=CARTESIAN_POINT('Ctrl Pts',(13.900770985429,-2.26640239233115,1.29080018513963));
#85147=CARTESIAN_POINT('Ctrl Pts',(13.8256890957265,-2.22841690655591,1.28548041809848));
#85148=CARTESIAN_POINT('Ctrl Pts',(13.7527955721518,-2.18684415657719,1.28016065105733));
#85149=CARTESIAN_POINT('Ctrl Pts',(13.6799020485771,-2.14527140659847,1.27484088401618));
#85150=CARTESIAN_POINT('Ctrl Pts',(13.6091972676224,-2.10011170871136,1.26952111697503));
#85151=CARTESIAN_POINT('Ctrl Pts',(13.5410369757164,-2.05164157292967,1.26420134993388));
#85152=CARTESIAN_POINT('Ctrl Pts',(13.4741232279713,-2.00405787943052,1.25897887303567));
#85153=CARTESIAN_POINT('Ctrl Pts',(13.4094090849756,-1.95310411137364,1.25375639613746));
#85154=CARTESIAN_POINT('Ctrl Pts',(13.347256781384,-1.89901187550754,1.24853391923926));
#85155=CARTESIAN_POINT('Ctrl Pts',(13.2851924765386,-1.84499622648807,1.24331883661919));
#85156=CARTESIAN_POINT('Ctrl Pts',(13.2256831586008,-1.78785123762157,1.23810375399912));
#85157=CARTESIAN_POINT('Ctrl Pts',(13.1690612555907,-1.72785114064289,1.23288867137906));
#85158=CARTESIAN_POINT('Ctrl Pts',(13.1125034378521,-1.66791895241148,1.22767949124491));
#85159=CARTESIAN_POINT('Ctrl Pts',(13.0588268608299,-1.60513841555441,1.22247031111076));
#85160=CARTESIAN_POINT('Ctrl Pts',(13.0083289359024,-1.53982226975597,1.21726113097661));
#85161=CARTESIAN_POINT('Ctrl Pts',(12.957861901448,-1.47454607899821,1.21205513739001));
#85162=CARTESIAN_POINT('Ctrl Pts',(12.9105699454521,-1.40673772684094,1.20684914380342));
#85163=CARTESIAN_POINT('Ctrl Pts',(12.8667110190326,-1.33674394469659,1.20164315021682));
#85164=CARTESIAN_POINT('Ctrl Pts',(12.8228652630735,-1.26677118108634,1.19643871994556));
#85165=CARTESIAN_POINT('Ctrl Pts',(12.7824507378214,-1.19461468686452,1.19123428967431));
#85166=CARTESIAN_POINT('Ctrl Pts',(12.7456819263984,-1.12064993331245,1.18602985940305));
#85167=CARTESIAN_POINT('Ctrl Pts',(12.7089127056805,-1.04668435641591,1.18082537119827));
#85168=CARTESIAN_POINT('Ctrl Pts',(12.675789485934,-0.970910900012858,1.17562088299349));
#85169=CARTESIAN_POINT('Ctrl Pts',(12.6464799915257,-0.893728045722679,
1.17041639478872));
#85170=CARTESIAN_POINT('Ctrl Pts',(12.6171422653402,-0.816470846610217,
1.16520689346601));
#85171=CARTESIAN_POINT('Ctrl Pts',(12.591625765819,-0.737801977180131,1.1599973921433));
#85172=CARTESIAN_POINT('Ctrl Pts',(12.570049153169,-0.658137623894178,1.15478789082059));
#85173=CARTESIAN_POINT('Ctrl Pts',(12.5484616479362,-0.578433053426348,
1.14957575957052));
#85174=CARTESIAN_POINT('Ctrl Pts',(12.5308180891762,-0.497732455885842,
1.14436362832046));
#85175=CARTESIAN_POINT('Ctrl Pts',(12.5171860071357,-0.416462395466049,
1.13915149707039));
#85176=CARTESIAN_POINT('Ctrl Pts',(12.5035311990925,-0.335056849974474,
1.13393067669209));
#85177=CARTESIAN_POINT('Ctrl Pts',(12.493901276518,-0.253080410737266,1.12870985631379));
#85178=CARTESIAN_POINT('Ctrl Pts',(12.4883118481157,-0.17096455095729,1.12348903593549));
#85179=CARTESIAN_POINT('Ctrl Pts',(12.4844199427861,-0.113787478575951,
1.11985379147163));
#85180=CARTESIAN_POINT('Ctrl Pts',(12.4824858930936,-0.0565428733787466,
1.11621854700778));
#85181=CARTESIAN_POINT('Ctrl Pts',(12.482500077493,0.000624641887355624,
1.11258330254392));
#85182=CARTESIAN_POINT('Ctrl Pts',(12.4825000774932,0.000624642704131756,
1.11258330249198));
#85183=CARTESIAN_POINT('Ctrl Pts',(12.4825084108427,0.0342105732934546,
1.11044759539204));
#85184=CARTESIAN_POINT('Ctrl Pts',(12.483188820319,0.0677874220149789,1.10831188829209));
#85185=CARTESIAN_POINT('Ctrl Pts',(12.4845403861397,0.101336967774151,1.10617618119214));
#85186=CARTESIAN_POINT('Ctrl Pts',(12.487867196913,0.183917474445178,1.10091924639843));
#85187=CARTESIAN_POINT('Ctrl Pts',(12.4952709795173,0.266485193006332,1.09566231160471));
#85188=CARTESIAN_POINT('Ctrl Pts',(12.5067530227982,0.348605451297277,1.090405376811));
#85189=CARTESIAN_POINT('Ctrl Pts',(12.5182208248965,0.430623855801245,1.08515496219548));
#85190=CARTESIAN_POINT('Ctrl Pts',(12.5337567860609,0.512195448942675,1.07990454757996));
#85191=CARTESIAN_POINT('Ctrl Pts',(12.5533102255289,0.592887339634366,1.07465413296444));
#85192=CARTESIAN_POINT('Ctrl Pts',(12.5728415567011,0.67348799521644,1.06940965478378));
#85193=CARTESIAN_POINT('Ctrl Pts',(12.5963812299632,0.753210479528745,1.06416517660313));
#85194=CARTESIAN_POINT('Ctrl Pts',(12.6238272147944,0.831630413614315,1.05892069842248));
#85195=CARTESIAN_POINT('Ctrl Pts',(12.6286229091916,0.845332892896281,1.05800431976885));
#85196=CARTESIAN_POINT('Ctrl Pts',(12.6335377426765,0.858995630875053,1.05708794111522));
#85197=CARTESIAN_POINT('Ctrl Pts',(12.6385710119932,0.872616401748845,1.05617156246159));
#85198=CARTESIAN_POINT('',(12.4825009284562,-0.00216212305302416,1.38677784361821));
#85199=CARTESIAN_POINT('Ctrl Pts',(12.6385710124998,0.872616403119952,1.33336808075876));
#85200=CARTESIAN_POINT('Ctrl Pts',(12.6355305680993,0.8643885110971,1.33393189393573));
#85201=CARTESIAN_POINT('Ctrl Pts',(12.6325330147833,0.856144426973078,1.33449432094504));
#85202=CARTESIAN_POINT('Ctrl Pts',(12.6173637559732,0.813735893510851,1.33737482604954));
#85203=CARTESIAN_POINT('Ctrl Pts',(12.6058878915727,0.779325997287395,1.33966980309984));
#85204=CARTESIAN_POINT('Ctrl Pts',(12.5835218975054,0.707097983881072,1.344404214739));
#85205=CARTESIAN_POINT('Ctrl Pts',(12.5727667838583,0.669248206453787,1.34683874017852));
#85206=CARTESIAN_POINT('Ctrl Pts',(12.5453463927905,0.563369916881544,1.35353261847241));
#85207=CARTESIAN_POINT('Ctrl Pts',(12.5306251909079,0.494873000545777,1.35773061810491));
#85208=CARTESIAN_POINT('Ctrl Pts',(12.4945139350419,0.28446855221848,1.37033632056842));
#85209=CARTESIAN_POINT('Ctrl Pts',(12.482377734934,0.141280026253996,1.3785060527829));
#85210=CARTESIAN_POINT('Ctrl Pts',(12.4825009284562,-0.00216212305302416,
1.38677784361821));
#85211=CARTESIAN_POINT('Ctrl Pts',(12.4825009299462,-0.00216385721130979,
1.38677794362086));
#85212=CARTESIAN_POINT('Ctrl Pts',(12.4825892483069,-0.104916196833896,
1.39270330065558));
#85213=CARTESIAN_POINT('Ctrl Pts',(12.4889682976042,-0.207560627536312,
1.3986735855389));
#85214=CARTESIAN_POINT('Ctrl Pts',(12.5048507408771,-0.335761172816142,
1.40649340025748));
#85215=CARTESIAN_POINT('Ctrl Pts',(12.5085147022134,-0.361947903654483,
1.40811012268778));
#85216=CARTESIAN_POINT('Ctrl Pts',(12.5162476916813,-0.411513873520081,
1.41121534118018));
#85217=CARTESIAN_POINT('Ctrl Pts',(12.520236180417,-0.434902856207706,1.41269981151196));
#85218=CARTESIAN_POINT('Ctrl Pts',(12.5283404218897,-0.478683422575586,
1.41552050337111));
#85219=CARTESIAN_POINT('Ctrl Pts',(12.5323793961633,-0.499086486809031,
1.41685272620698));
#85220=CARTESIAN_POINT('Ctrl Pts',(12.5435701409766,-0.552156532842023,
1.42036090508382));
#85221=CARTESIAN_POINT('Ctrl Pts',(12.5511207110053,-0.584734522784112,
1.42255687870184));
#85222=CARTESIAN_POINT('Ctrl Pts',(12.5898208418566,-0.737784271775964,
1.43304460782569));
#85223=CARTESIAN_POINT('Ctrl Pts',(12.6292237528481,-0.855981706468816,
1.44163978898629));
#85224=CARTESIAN_POINT('Ctrl Pts',(12.7213243261735,-1.07635404331246,1.45812984796642));
#85225=CARTESIAN_POINT('Ctrl Pts',(12.7726008054748,-1.17881185003668,1.46600707315879));
#85226=CARTESIAN_POINT('Ctrl Pts',(12.8696346885768,-1.34359419022276,1.47886567489774));
#85227=CARTESIAN_POINT('Ctrl Pts',(12.9116047242935,-1.40794490190253,1.48394247053915));
#85228=CARTESIAN_POINT('Ctrl Pts',(12.98004715759,-1.50307306120157,1.49152961640535));
#85229=CARTESIAN_POINT('Ctrl Pts',(13.0044264765366,-1.53529304490731,1.49411517126841));
#85230=CARTESIAN_POINT('Ctrl Pts',(13.0519589120643,-1.59506610975866,1.49894622858357));
#85231=CARTESIAN_POINT('Ctrl Pts',(13.0749475629069,-1.62273636235345,1.50119737576193));
#85232=CARTESIAN_POINT('Ctrl Pts',(13.13024775295,-1.6864685397244,1.50642393084478));
#85233=CARTESIAN_POINT('Ctrl Pts',(13.1630226564683,-1.72211042331781,1.50937939223633));
#85234=CARTESIAN_POINT('Ctrl Pts',(13.3242278965214,-1.88757397845849,1.52330546163752));
#85235=CARTESIAN_POINT('Ctrl Pts',(13.4654987813836,-2.00411064473487,1.5336958325686));
#85236=CARTESIAN_POINT('Ctrl Pts',(13.6850933788845,-2.14831148067518,1.54883717387851));
#85237=CARTESIAN_POINT('Ctrl Pts',(13.7541011920106,-2.18905376466235,1.55347870452628));
#85238=CARTESIAN_POINT('Ctrl Pts',(13.8702200028078,-2.25033909973641,1.56128444311747));
#85239=CARTESIAN_POINT('Ctrl Pts',(13.916226581866,-2.2728535651194,1.56437634709942));
#85240=CARTESIAN_POINT('Ctrl Pts',(13.9848749127448,-2.30389013378527,1.56903456425697));
#85241=CARTESIAN_POINT('Ctrl Pts',(14.0070064947898,-2.31351517900331,1.57054299525911));
#85242=CARTESIAN_POINT('Ctrl Pts',(14.0483277918833,-2.33078373093992,1.57337777282385));
#85243=CARTESIAN_POINT('Ctrl Pts',(14.0674791081453,-2.33851180385144,1.57469933416925));
#85244=CARTESIAN_POINT('Ctrl Pts',(14.1169631171702,-2.35777547884206,1.57813098772628));
#85245=CARTESIAN_POINT('Ctrl Pts',(14.1474270361532,-2.36896147095265,1.5802594486682));
#85246=CARTESIAN_POINT('Ctrl Pts',(14.3148833064831,-2.42680120916045,1.59201338086093));
#85247=CARTESIAN_POINT('Ctrl Pts',(14.4554793639651,-2.4621618230667,1.60206073063141));
#85248=CARTESIAN_POINT('Ctrl Pts',(14.7001148641056,-2.50170090304566,1.61915343978747));
#85249=CARTESIAN_POINT('Ctrl Pts',(14.8028283632692,-2.51188473217001,1.62622000138453));
#85250=CARTESIAN_POINT('Ctrl Pts',(14.9782121176192,-2.51844599464298,1.63798655529033));
#85251=CARTESIAN_POINT('Ctrl Pts',(15.0506284814945,-2.51803164444162,1.64276002376625));
#85252=CARTESIAN_POINT('Ctrl Pts',(15.1626026507913,-2.51255728619015,1.65000757925224));
#85253=CARTESIAN_POINT('Ctrl Pts',(15.2022231379348,-2.50967922932441,1.65254636893324));
#85254=CARTESIAN_POINT('Ctrl Pts',(15.2777386914124,-2.50239363856914,1.65734025358771));
#85255=CARTESIAN_POINT('Ctrl Pts',(15.3136389826725,-2.49814801535511,1.65959975926562));
#85256=CARTESIAN_POINT('Ctrl Pts',(15.3988644029457,-2.48620282888378,1.66492380853644));
#85257=CARTESIAN_POINT('Ctrl Pts',(15.4480772062119,-2.47780641812479,1.6679659463003));
#85258=CARTESIAN_POINT('Ctrl Pts',(15.6114402148443,-2.44490742603661,1.67799269507686));
#85259=CARTESIAN_POINT('Ctrl Pts',(15.7241337920546,-2.41393149915663,1.68478407736683));
#85260=CARTESIAN_POINT('Ctrl Pts',(15.9505326720198,-2.33441127903611,1.69861748860469));
#85261=CARTESIAN_POINT('Ctrl Pts',(16.0636257656841,-2.28510085937189,1.70563446276486));
#85262=CARTESIAN_POINT('Ctrl Pts',(16.2301373500441,-2.19745058220073,1.71670126144634));
#85263=CARTESIAN_POINT('Ctrl Pts',(16.2864285066132,-2.16497743004938,1.72058322386198));
#85264=CARTESIAN_POINT('Ctrl Pts',(16.363449672329,-2.1164806704514,1.7261840735252));
#85265=CARTESIAN_POINT('Ctrl Pts',(16.3852852783155,-2.10225355397403,1.72780599617266));
#85266=CARTESIAN_POINT('Ctrl Pts',(16.4238841942221,-2.07624173984677,1.73074196355354));
#85267=CARTESIAN_POINT('Ctrl Pts',(16.4407311235664,-2.06458705151344,1.73204799773991));
#85268=CARTESIAN_POINT('Ctrl Pts',(16.4812585302018,-2.03581265527393,1.73524924518821));
#85269=CARTESIAN_POINT('Ctrl Pts',(16.5047857137513,-2.01848452501289,1.73715721951164));
#85270=CARTESIAN_POINT('Ctrl Pts',(16.6069693764728,-1.94044530022182,1.74564598920864));
#85271=CARTESIAN_POINT('Ctrl Pts',(16.6822878264905,-1.87552198042389,1.75243769924464));
#85272=CARTESIAN_POINT('Ctrl Pts',(16.8518608558646,-1.71090184000058,1.76871839540953));
#85273=CARTESIAN_POINT('Ctrl Pts',(16.9422097971594,-1.60760679634545,1.77821819657449));
#85274=CARTESIAN_POINT('Ctrl Pts',(17.0738212460485,-1.42974460685774,1.79316314695867));
#85275=CARTESIAN_POINT('Ctrl Pts',(17.1205075522731,-1.35954200723028,1.79875588217141));
#85276=CARTESIAN_POINT('Ctrl Pts',(17.184790037352,-1.25148639879039,1.80691307446885));
#85277=CARTESIAN_POINT('Ctrl Pts',(17.2051078310174,-1.21532937950084,1.80957213251245));
#85278=CARTESIAN_POINT('Ctrl Pts',(17.2412782557656,-1.14706518937248,1.81446706412267));
#85279=CARTESIAN_POINT('Ctrl Pts',(17.25735692092,-1.11509044926652,1.81671043248044));
#85280=CARTESIAN_POINT('Ctrl Pts',(17.2924073181679,-1.04152002741431,1.82176677462674));
#85281=CARTESIAN_POINT('Ctrl Pts',(17.3109390574179,-0.999728140014245,
1.82456423269701));
#85282=CARTESIAN_POINT('Ctrl Pts',(17.4042153827483,-0.772899745720214,
1.83939365813419));
#85283=CARTESIAN_POINT('Ctrl Pts',(17.4578958067133,-0.579982247226776,
1.85069374923668));
#85284=CARTESIAN_POINT('Ctrl Pts',(17.4993450584043,-0.310516115700269,
1.86644054002961));
#85285=CARTESIAN_POINT('Ctrl Pts',(17.5073040946449,-0.237846517424953,
1.87069213030698));
#85286=CARTESIAN_POINT('Ctrl Pts',(17.5152606123427,-0.116664778559043,
1.87793122705907));
#85287=CARTESIAN_POINT('Ctrl Pts',(17.5170377935756,-0.0683133356656833,
1.88085910329622));
#85288=CARTESIAN_POINT('Ctrl Pts',(17.517608524097,0.0037259544731554,1.88531917079733));
#85289=CARTESIAN_POINT('Ctrl Pts',(17.5174621925834,0.0273965498554707,
1.88680038766788));
#85290=CARTESIAN_POINT('Ctrl Pts',(17.5165597759672,0.0718803955753969,
1.88961945263629));
#85291=CARTESIAN_POINT('Ctrl Pts',(17.5158791451036,0.0926925086391416,
1.89095341406106));
#85292=CARTESIAN_POINT('Ctrl Pts',(17.5134260278189,0.147052398414725,1.89447359008228));
#85293=CARTESIAN_POINT('Ctrl Pts',(17.5112400549014,0.180576670410615,1.89668007933511));
#85294=CARTESIAN_POINT('Ctrl Pts',(17.4988012058636,0.326346885681827,1.90640136823097));
#85295=CARTESIAN_POINT('Ctrl Pts',(17.4816880976136,0.43786993804315,1.91416191140293));
#85296=CARTESIAN_POINT('Ctrl Pts',(17.4306564751432,0.666747111005294,1.93034945422796));
#85297=CARTESIAN_POINT('Ctrl Pts',(17.3955541265528,0.783560543061855,1.93875597559673));
#85298=CARTESIAN_POINT('Ctrl Pts',(17.3238259030189,0.971568041452843,1.95230904323382));
#85299=CARTESIAN_POINT('Ctrl Pts',(17.2920255170955,1.0443813841952,1.95756681384005));
#85300=CARTESIAN_POINT('Ctrl Pts',(17.2387610699576,1.15213644022985,1.96535494368297));
#85301=CARTESIAN_POINT('Ctrl Pts',(17.219802414759,1.18825378687309,1.96796709407843));
#85302=CARTESIAN_POINT('Ctrl Pts',(17.1825262863821,1.25525823529334,1.97282047676086));
#85303=CARTESIAN_POINT('Ctrl Pts',(17.1644096465376,1.28624465844413,1.97506803624026));
#85304=CARTESIAN_POINT('Ctrl Pts',(17.1211458153943,1.35673827949321,1.98019454043744));
#85305=CARTESIAN_POINT('Ctrl Pts',(17.0955462649591,1.3959529392483,1.98305622246118));
#85306=CARTESIAN_POINT('Ctrl Pts',(16.9599922186528,1.59146103927357,1.99741846958626));
#85307=CARTESIAN_POINT('Ctrl Pts',(16.8335965174715,1.73558270055007,2.00826530212706));
#85308=CARTESIAN_POINT('Ctrl Pts',(16.6354761722271,1.91543031199457,2.02370243437099));
#85309=CARTESIAN_POINT('Ctrl Pts',(16.5765374994451,1.96422600629548,2.02814336314053));
#85310=CARTESIAN_POINT('Ctrl Pts',(16.475725445798,2.04022508747897,2.0356588733976));
#85311=CARTESIAN_POINT('Ctrl Pts',(16.4351005888672,2.0690020774596,2.03866779232439));
#85312=CARTESIAN_POINT('Ctrl Pts',(16.3737471440655,2.10978585218213,2.04322584831046));
#85313=CARTESIAN_POINT('Ctrl Pts',(16.353655179001,2.12273293430859,2.04472064667779));
#85314=CARTESIAN_POINT('Ctrl Pts',(16.315796830307,2.14637247547994,2.0475471671789));
#85315=CARTESIAN_POINT('Ctrl Pts',(16.2980773879768,2.15713492253999,2.04887454940363));
#85316=CARTESIAN_POINT('Ctrl Pts',(16.2518140099119,2.18445803425106,2.05234853733703));
#85317=CARTESIAN_POINT('Ctrl Pts',(16.2230743446823,2.20067810460126,2.05451442449593));
#85318=CARTESIAN_POINT('Ctrl Pts',(16.0765527714209,2.27961523632146,2.06556467230243));
#85319=CARTESIAN_POINT('Ctrl Pts',(15.9542423588839,2.33345838445376,2.07480287282561));
#85320=CARTESIAN_POINT('Ctrl Pts',(15.7250141946449,2.41331977972933,2.09155788131163));
#85321=CARTESIAN_POINT('Ctrl Pts',(15.6195359333951,2.44252667976103,2.09906899473149));
#85322=CARTESIAN_POINT('Ctrl Pts',(15.4599903239398,2.47569991955132,2.11001272623214));
#85323=CARTESIAN_POINT('Ctrl Pts',(15.4071565630592,2.48493568833214,2.11357175830024));
#85324=CARTESIAN_POINT('Ctrl Pts',(15.3074572408588,2.49909832027411,2.12016291192237));
#85325=CARTESIAN_POINT('Ctrl Pts',(15.260670592234,2.50441084814274,2.12320507377839));
#85326=CARTESIAN_POINT('Ctrl Pts',(15.1780557861838,2.51145105875922,2.12849144563821));
#85327=CARTESIAN_POINT('Ctrl Pts',(15.1422895026663,2.51373113006754,2.13075211386224));
#85328=CARTESIAN_POINT('Ctrl Pts',(15.0654104952545,2.51698587026842,2.13555631238731));
#85329=CARTESIAN_POINT('Ctrl Pts',(15.0242976787143,2.51771847698641,2.13809171566911));
#85330=CARTESIAN_POINT('Ctrl Pts',(14.9014902289023,2.51689812121091,2.14557988627));
#85331=CARTESIAN_POINT('Ctrl Pts',(14.8198674198282,2.51237624622363,2.150442400473));
#85332=CARTESIAN_POINT('Ctrl Pts',(14.6935232123984,2.49918637817835,2.15788702321381));
#85333=CARTESIAN_POINT('Ctrl Pts',(14.6485778876443,2.49326357614882,2.16051953685836));
#85334=CARTESIAN_POINT('Ctrl Pts',(14.471537435022,2.46505081649111,2.17088193332234));
#85335=CARTESIAN_POINT('Ctrl Pts',(14.3411584247098,2.43344881236856,2.17848704099896));
#85336=CARTESIAN_POINT('Ctrl Pts',(14.1496998141575,2.37052006330617,2.19031949517956));
#85337=CARTESIAN_POINT('Ctrl Pts',(14.086362808083,2.34683645070651,2.19435154665354));
#85338=CARTESIAN_POINT('Ctrl Pts',(13.9997490364697,2.31041119111617,2.2001294707858));
#85339=CARTESIAN_POINT('Ctrl Pts',(13.9756003579974,2.29980588345927,2.20176985699335));
#85340=CARTESIAN_POINT('Ctrl Pts',(13.9330227528557,2.28030357624855,2.20472239058758));
#85341=CARTESIAN_POINT('Ctrl Pts',(13.9145281735862,2.27155798263263,2.20602597528365));
#85342=CARTESIAN_POINT('Ctrl Pts',(13.8702549237056,2.24995821636688,2.20919716297465));
#85343=CARTESIAN_POINT('Ctrl Pts',(13.8445875979461,2.23688576417375,2.21107683855228));
#85344=CARTESIAN_POINT('Ctrl Pts',(13.7395842249338,2.1811178516321,2.21892096953529));
#85345=CARTESIAN_POINT('Ctrl Pts',(13.6623493878982,2.13462197723981,2.22505812695252));
#85346=CARTESIAN_POINT('Ctrl Pts',(13.4856177280682,2.01486526181441,2.23973865984903));
#85347=CARTESIAN_POINT('Ctrl Pts',(13.3886793635801,1.9382166314849,2.24830699285757));
#85348=CARTESIAN_POINT('Ctrl Pts',(13.2230053353671,1.78616609995838,2.26362234613225));
#85349=CARTESIAN_POINT('Ctrl Pts',(13.1524667552495,1.71310377161154,2.270410727781));
#85350=CARTESIAN_POINT('Ctrl Pts',(13.0582340114413,1.60288683694009,2.2798525055689));
#85351=CARTESIAN_POINT('Ctrl Pts',(13.0308061955652,1.56906899529796,2.28265296446426));
#85352=CARTESIAN_POINT('Ctrl Pts',(12.9825291142042,1.5062832854388,2.28768436759806));
#85353=CARTESIAN_POINT('Ctrl Pts',(12.9613928204058,1.4775517207062,2.28992617231733));
#85354=CARTESIAN_POINT('Ctrl Pts',(12.9156291945434,1.4124906611709,2.29487491189316));
#85355=CARTESIAN_POINT('Ctrl Pts',(12.8913266425681,1.37594642151091,2.29756915648175));
#85356=CARTESIAN_POINT('Ctrl Pts',(12.8175004395359,1.25837840057791,2.3059926533752));
#85357=CARTESIAN_POINT('Ctrl Pts',(12.7715964034195,1.17517678895927,2.31159524001484));
#85358=CARTESIAN_POINT('Ctrl Pts',(12.6964686834177,1.01869138548658,2.32169059877296));
#85359=CARTESIAN_POINT('Ctrl Pts',(12.6657962272505,0.946291839447466,2.32620136657629));
#85360=CARTESIAN_POINT('Ctrl Pts',(12.6385710877721,0.872616606817863,2.33071866803842));
#85361=CARTESIAN_POINT('Origin',(15.,0.,3.));
#85362=CARTESIAN_POINT('',(12.6385710144774,0.87261640847139,3.32953357812844));
#85363=CARTESIAN_POINT('',(12.6408521577454,0.871797393741481,3.05636274128509));
#85364=CARTESIAN_POINT('',(12.6385710119932,0.872616401748847,3.));
#85365=CARTESIAN_POINT('',(12.4849790795627,0.00159552663997447,2.11258330249198));
#85366=CARTESIAN_POINT('Ctrl Pts',(12.6408521577454,0.87179739374149,3.05636274128509));
#85367=CARTESIAN_POINT('Ctrl Pts',(12.7375264301118,1.13962417266692,3.03840122955439));
#85368=CARTESIAN_POINT('Ctrl Pts',(13.2888950829206,2.12729580985852,2.96776466157644));
#85369=CARTESIAN_POINT('Ctrl Pts',(15.3377008476539,2.95164299596017,2.84445303735124));
#85370=CARTESIAN_POINT('Ctrl Pts',(17.6568119242111,1.32950708964651,2.6864278686095));
#85371=CARTESIAN_POINT('Ctrl Pts',(17.5649293736244,-1.49912516962393,2.52840269986778));
#85372=CARTESIAN_POINT('Ctrl Pts',(15.1454344282297,-2.96733641764902,2.37037753112603));
#85373=CARTESIAN_POINT('Ctrl Pts',(12.9074954366079,-1.89324175649192,2.23177106533412));
#85374=CARTESIAN_POINT('Ctrl Pts',(12.4885048299379,-0.525856856019931,
2.14583965578942));
#85375=CARTESIAN_POINT('Ctrl Pts',(12.4854125712649,0.00159525163329232,
2.11258330249198));
#85376=CARTESIAN_POINT('Ctrl Pts',(12.4825005065989,0.00159709904406843,
2.11258330249198));
#85377=CARTESIAN_POINT('Ctrl Pts',(12.4825600916737,0.0955207640184819,
2.10666815249281));
#85378=CARTESIAN_POINT('Ctrl Pts',(12.4878799426804,0.189246299602191,2.10075300249363));
#85379=CARTESIAN_POINT('Ctrl Pts',(12.498369487036,0.282225134612964,2.09483785249446));
#85380=CARTESIAN_POINT('Ctrl Pts',(12.5089078977187,0.375637118482618,2.08889514632649));
#85381=CARTESIAN_POINT('Ctrl Pts',(12.5246641526241,0.468295217851566,2.08295244015852));
#85382=CARTESIAN_POINT('Ctrl Pts',(12.5454968432786,0.559661061397646,2.07700973399055));
#85383=CARTESIAN_POINT('Ctrl Pts',(12.5664420987786,0.651520580111855,2.07103491772155));
#85384=CARTESIAN_POINT('Ctrl Pts',(12.592518678278,0.742073636519814,2.06506010145255));
#85385=CARTESIAN_POINT('Ctrl Pts',(12.6235347394388,0.83079426776169,2.05908528518355));
#85386=CARTESIAN_POINT('Ctrl Pts',(12.6284244458395,0.844781144954579,2.05814335070637));
#85387=CARTESIAN_POINT('Ctrl Pts',(12.6334368223796,0.858722525631891,2.05720141622918));
#85388=CARTESIAN_POINT('Ctrl Pts',(12.6385710119932,0.872616401748851,2.05625948175199));
#85389=CARTESIAN_POINT('Ctrl Pts',(12.6385710877721,0.872616606817863,2.33071866803842));
#85390=CARTESIAN_POINT('Ctrl Pts',(12.6130828119274,0.803641582697994,2.33494778230365));
#85391=CARTESIAN_POINT('Ctrl Pts',(12.5906160635846,0.733548458146182,2.33918298169588));
#85392=CARTESIAN_POINT('Ctrl Pts',(12.5524234413054,0.593540129543784,2.34768324219969));
#85393=CARTESIAN_POINT('Ctrl Pts',(12.5365523828507,0.523779504389352,2.35193820193661));
#85394=CARTESIAN_POINT('Ctrl Pts',(12.5188442919751,0.427073034483106,2.35797802765619));
#85395=CARTESIAN_POINT('Ctrl Pts',(12.5144371661924,0.400627362594168,2.35964408622218));
#85396=CARTESIAN_POINT('Ctrl Pts',(12.507416771345,0.353910509147975,2.36262047332756));
#85397=CARTESIAN_POINT('Ctrl Pts',(12.5046265882995,0.333669376866167,2.36392147830763));
#85398=CARTESIAN_POINT('Ctrl Pts',(12.4985634376397,0.285343195659269,2.36705479121824));
#85399=CARTESIAN_POINT('Ctrl Pts',(12.4955168157114,0.257234194162914,2.36889828846849));
#85400=CARTESIAN_POINT('Ctrl Pts',(12.4860363282071,0.153480172861711,2.37576578528259));
#85401=CARTESIAN_POINT('Ctrl Pts',(12.4825520719847,0.0776112608302906,
2.38090946543098));
#85402=CARTESIAN_POINT('Ctrl Pts',(12.4823712472628,-0.188935106255942,
2.39917119488424));
#85403=CARTESIAN_POINT('Ctrl Pts',(12.5038986407159,-0.379004630001638,
2.41247744373233));
#85404=CARTESIAN_POINT('Ctrl Pts',(12.561621777294,-0.62972438427405,2.4296525467515));
#85405=CARTESIAN_POINT('Ctrl Pts',(12.5791332370533,-0.69400762931579,2.43402857148568));
#85406=CARTESIAN_POINT('Ctrl Pts',(12.6108458804789,-0.794514453660138,
2.44082697973957));
#85407=CARTESIAN_POINT('Ctrl Pts',(12.6233705584292,-0.831230048995139,
2.44330128017505));
#85408=CARTESIAN_POINT('Ctrl Pts',(12.6493220850701,-0.901916037334384,
2.44805104517824));
#85409=CARTESIAN_POINT('Ctrl Pts',(12.6626494599651,-0.935912320495879,
2.45032908331539));
#85410=CARTESIAN_POINT('Ctrl Pts',(12.6969570928146,-1.01811718436349,2.45582918360601));
#85411=CARTESIAN_POINT('Ctrl Pts',(12.7187172560145,-1.06598258021218,2.45902438756089));
#85412=CARTESIAN_POINT('Ctrl Pts',(12.7697381517989,-1.1694805662318,2.46594578407214));
#85413=CARTESIAN_POINT('Ctrl Pts',(12.7996153607669,-1.22476972659078,2.46965127771572));
#85414=CARTESIAN_POINT('Ctrl Pts',(12.9115164949221,-1.41450838567484,2.48250609407803));
#85415=CARTESIAN_POINT('Ctrl Pts',(13.0040449393849,-1.54232234967238,2.49139891274401));
#85416=CARTESIAN_POINT('Ctrl Pts',(13.1569229405479,-1.71650687108799,2.50494199649724));
#85417=CARTESIAN_POINT('Ctrl Pts',(13.208388994884,-1.77015733273108,2.50935071471145));
#85418=CARTESIAN_POINT('Ctrl Pts',(13.2803226749894,-1.83878960470903,2.51544573372024));
#85419=CARTESIAN_POINT('Ctrl Pts',(13.2987557962732,-1.85585704180918,2.51700216684152));
#85420=CARTESIAN_POINT('Ctrl Pts',(13.3327264208623,-1.88637943135215,2.5198675830547));
#85421=CARTESIAN_POINT('Ctrl Pts',(13.3481784054611,-1.89992471664867,2.52117017057166));
#85422=CARTESIAN_POINT('Ctrl Pts',(13.3832170828368,-1.92988919622541,2.52412446271687));
#85423=CARTESIAN_POINT('Ctrl Pts',(13.4028895777065,-1.9462007821441,2.52578271121433));
#85424=CARTESIAN_POINT('Ctrl Pts',(13.4703418359251,-2.0004178826431,2.53145717917954));
#85425=CARTESIAN_POINT('Ctrl Pts',(13.5192468228761,-2.03688356324417,2.53555225558514));
#85426=CARTESIAN_POINT('Ctrl Pts',(13.6589586137463,-2.13336683449742,2.54709888821033));
#85427=CARTESIAN_POINT('Ctrl Pts',(13.7524063522685,-2.18932756366017,2.55464758714719));
#85428=CARTESIAN_POINT('Ctrl Pts',(13.968793545032,-2.30054489448085,2.57141144763015));
#85429=CARTESIAN_POINT('Ctrl Pts',(14.0931555196742,-2.35234673683755,2.58056594074289));
#85430=CARTESIAN_POINT('Ctrl Pts',(14.2693340079656,-2.40966987317855,2.59274870356547));
#85431=CARTESIAN_POINT('Ctrl Pts',(14.3180589205194,-2.42390978730885,2.59604124906964));
#85432=CARTESIAN_POINT('Ctrl Pts',(14.4022742725217,-2.44578097548938,2.60160536773693));
#85433=CARTESIAN_POINT('Ctrl Pts',(14.4375586730536,-2.45413540800816,2.60389931376189));
#85434=CARTESIAN_POINT('Ctrl Pts',(14.5115320331716,-2.46997105733845,2.60863569393038));
#85435=CARTESIAN_POINT('Ctrl Pts',(14.5502410776344,-2.47731208371283,2.61107312739481));
#85436=CARTESIAN_POINT('Ctrl Pts',(14.6584923043308,-2.49522036063281,2.61778778958015));
#85437=CARTESIAN_POINT('Ctrl Pts',(14.728330640856,-2.50378696515588,2.62200299266667));
#85438=CARTESIAN_POINT('Ctrl Pts',(14.896343800069,-2.51728195899517,2.63195379493515));
#85439=CARTESIAN_POINT('Ctrl Pts',(14.9946267218981,-2.51940978863386,2.63761894385376));
#85440=CARTESIAN_POINT('Ctrl Pts',(15.2478670917557,-2.51006993620561,2.65219537605792));
#85441=CARTESIAN_POINT('Ctrl Pts',(15.4020694883506,-2.49002372021481,2.66104420567355));
#85442=CARTESIAN_POINT('Ctrl Pts',(15.5840392331565,-2.44901801812302,2.67240481473275));
#85443=CARTESIAN_POINT('Ctrl Pts',(15.6145202497099,-2.4415478145329,2.6743402209903));
#85444=CARTESIAN_POINT('Ctrl Pts',(15.6648707888756,-2.42820550531402,2.67760334491258));
#85445=CARTESIAN_POINT('Ctrl Pts',(15.6848213586035,-2.42265449900531,2.67891393963998));
#85446=CARTESIAN_POINT('Ctrl Pts',(15.7284563377012,-2.40993149874373,2.68182229987095));
#85447=CARTESIAN_POINT('Ctrl Pts',(15.7521056541362,-2.40265591258142,2.6834251502501));
#85448=CARTESIAN_POINT('Ctrl Pts',(15.8281476360055,-2.37802936055742,2.68865666441717));
#85449=CARTESIAN_POINT('Ctrl Pts',(15.8800753365586,-2.35930469086154,2.69234920354004));
#85450=CARTESIAN_POINT('Ctrl Pts',(16.015735118432,-2.30528523044506,2.70224519428313));
#85451=CARTESIAN_POINT('Ctrl Pts',(16.0982447167614,-2.2671380950189,2.70852057197804));
#85452=CARTESIAN_POINT('Ctrl Pts',(16.320671280704,-2.149305839092,2.72589844658641));
#85453=CARTESIAN_POINT('Ctrl Pts',(16.4553064853032,-2.06053028658965,2.73692750398818));
#85454=CARTESIAN_POINT('Ctrl Pts',(16.619939130365,-1.92773522883161,2.75083350506466));
#85455=CARTESIAN_POINT('Ctrl Pts',(16.658353873918,-1.89478994227332,2.7541154273558));
#85456=CARTESIAN_POINT('Ctrl Pts',(16.7225325009139,-1.83630087459142,2.75966760613806));
#85457=CARTESIAN_POINT('Ctrl Pts',(16.7487840597598,-1.81131820848578,2.76195997955683));
#85458=CARTESIAN_POINT('Ctrl Pts',(16.802472068631,-1.75796956885561,2.76669819636012));
#85459=CARTESIAN_POINT('Ctrl Pts',(16.8297994785494,-1.72950764734889,2.76913892611866));
#85460=CARTESIAN_POINT('Ctrl Pts',(16.9041951128387,-1.64828529421477,2.77587849233801));
#85461=CARTESIAN_POINT('Ctrl Pts',(16.9497281181776,-1.59416591792567,2.78011447275607));
#85462=CARTESIAN_POINT('Ctrl Pts',(17.0534578394276,-1.45977122291452,2.79013440968192));
#85463=CARTESIAN_POINT('Ctrl Pts',(17.1093099128012,-1.37783682148057,2.79584638422875));
#85464=CARTESIAN_POINT('Ctrl Pts',(17.2389235182868,-1.16126401172449,2.81036317370143));
#85465=CARTESIAN_POINT('Ctrl Pts',(17.3054659665301,-1.02280423164037,2.81911118867626));
#85466=CARTESIAN_POINT('Ctrl Pts',(17.3700250243665,-0.849579321335824,
2.83036641633348));
#85467=CARTESIAN_POINT('Ctrl Pts',(17.3804956210495,-0.819782912112732,
2.83231355926413));
#85468=CARTESIAN_POINT('Ctrl Pts',(17.3969076442725,-0.770110354874441,
2.83559011838298));
#85469=CARTESIAN_POINT('Ctrl Pts',(17.4031687656677,-0.750343968663925,
2.83690207018901));
#85470=CARTESIAN_POINT('Ctrl Pts',(17.4163358327527,-0.706919114294123,
2.83980509790709));
#85471=CARTESIAN_POINT('Ctrl Pts',(17.4231392968821,-0.683234458002295,
2.84140107421867));
#85472=CARTESIAN_POINT('Ctrl Pts',(17.4438732357607,-0.606845538499601,
2.84658048117067));
#85473=CARTESIAN_POINT('Ctrl Pts',(17.4564392045818,-0.553790066614681,
2.85022612797859));
#85474=CARTESIAN_POINT('Ctrl Pts',(17.4849478752528,-0.413217588018961,
2.85994264232883));
#85475=CARTESIAN_POINT('Ctrl Pts',(17.4979921456865,-0.325190309535636,
2.86608279581412));
#85476=CARTESIAN_POINT('Ctrl Pts',(17.5218021037186,-0.0730320571787507,
2.88356974141117));
#85477=CARTESIAN_POINT('Ctrl Pts',(17.5211937633259,0.0917399181762342,
2.89484575169084));
#85478=CARTESIAN_POINT('Ctrl Pts',(17.4994180485582,0.3053669965451,2.90895903658735));
#85479=CARTESIAN_POINT('Ctrl Pts',(17.4928131991141,0.35527809862235,2.91222318375574));
#85480=CARTESIAN_POINT('Ctrl Pts',(17.4788929623976,0.440688453307653,2.91775540713375));
#85481=CARTESIAN_POINT('Ctrl Pts',(17.472299877668,0.476287903941779,2.92004517318884));
#85482=CARTESIAN_POINT('Ctrl Pts',(17.4569016892818,0.550458471127815,2.92478662970764));
#85483=CARTESIAN_POINT('Ctrl Pts',(17.4479506260041,0.588989341534187,2.92723301440188));
#85484=CARTESIAN_POINT('Ctrl Pts',(17.4203246556744,0.696362639868777,2.93401544195895));
#85485=CARTESIAN_POINT('Ctrl Pts',(17.3996265525521,0.76464767828463,2.93828718784357));
#85486=CARTESIAN_POINT('Ctrl Pts',(17.342825289282,0.926869305729871,2.94842705298447));
#85487=CARTESIAN_POINT('Ctrl Pts',(17.3039381821449,1.01969966267607,2.95422048736621));
#85488=CARTESIAN_POINT('Ctrl Pts',(17.1934216397223,1.24468417293609,2.96863602741457));
#85489=CARTESIAN_POINT('Ctrl Pts',(17.1153323408748,1.37320649594988,2.97721026736162));
#85490=CARTESIAN_POINT('Ctrl Pts',(17.0073312115788,1.51968636251021,2.98828432077836));
#85491=CARTESIAN_POINT('Ctrl Pts',(16.9879016592406,1.54501521219778,2.99025146605093));
#85492=CARTESIAN_POINT('Ctrl Pts',(16.9550372473264,1.58621167316143,2.99355103380811));
#85493=CARTESIAN_POINT('Ctrl Pts',(16.9418782426142,1.60229428519577,2.9948654084667));
#85494=CARTESIAN_POINT('Ctrl Pts',(16.9127871596869,1.63696385526219,2.99775989330806));
#85495=CARTESIAN_POINT('Ctrl Pts',(16.8967816829363,1.65548316719344,2.99934459960838));
#85496=CARTESIAN_POINT('Ctrl Pts',(16.844992187807,1.71366972343203,3.0044397920781));
#85497=CARTESIAN_POINT('Ctrl Pts',(16.8082162523907,1.75243066238104,3.00800985827858));
#85498=CARTESIAN_POINT('Ctrl Pts',(16.7091447474894,1.8504089865478,3.01744199859366));
#85499=CARTESIAN_POINT('Ctrl Pts',(16.6450004613352,1.90765863392137,3.02336923184861));
#85500=CARTESIAN_POINT('Ctrl Pts',(16.4454745230108,2.06817925568255,3.04104935564278));
#85501=CARTESIAN_POINT('Ctrl Pts',(16.3023985038526,2.16114238104892,3.05273767550511));
#85502=CARTESIAN_POINT('Ctrl Pts',(16.1067230811676,2.26173627178208,3.06718909568718));
#85503=CARTESIAN_POINT('Ctrl Pts',(16.061758768532,2.28318983665751,3.07041740641836));
#85504=CARTESIAN_POINT('Ctrl Pts',(15.9831272891693,2.31788103496291,3.07590949396312));
#85505=CARTESIAN_POINT('Ctrl Pts',(15.9497583212086,2.33175279769755,3.07819410377899));
#85506=CARTESIAN_POINT('Ctrl Pts',(15.8790662600272,2.35937060683458,3.08294276886838));
#85507=CARTESIAN_POINT('Ctrl Pts',(15.8416926153348,2.37296038055608,3.08540111823881));
#85508=CARTESIAN_POINT('Ctrl Pts',(15.7351636844384,2.4088625810652,3.09227483770303));
#85509=CARTESIAN_POINT('Ctrl Pts',(15.6653404518237,2.42907554873721,3.09662279191374));
#85510=CARTESIAN_POINT('Ctrl Pts',(15.493891193051,2.47075868189329,3.10702225593738));
#85511=CARTESIAN_POINT('Ctrl Pts',(15.391623489351,2.48901778442396,3.11299302852617));
#85512=CARTESIAN_POINT('Ctrl Pts',(15.146065686656,2.51734657695677,3.12720674622698));
#85513=CARTESIAN_POINT('Ctrl Pts',(15.0024850399308,2.52157764254631,3.13541741038279));
#85514=CARTESIAN_POINT('Ctrl Pts',(14.8268331670838,2.51174833795092,3.14611140176326));
#85515=CARTESIAN_POINT('Ctrl Pts',(14.7943632052678,2.50929865528764,3.14811614536501));
#85516=CARTESIAN_POINT('Ctrl Pts',(14.7413773863779,2.50426590346203,3.15144647134996));
#85517=CARTESIAN_POINT('Ctrl Pts',(14.7208286087857,2.50205848914436,3.15275271131997));
#85518=CARTESIAN_POINT('Ctrl Pts',(14.6763964592994,2.49673127055157,3.15561252389852));
#85519=CARTESIAN_POINT('Ctrl Pts',(14.6525271857858,2.49352137043495,3.15717037702822));
#85520=CARTESIAN_POINT('Ctrl Pts',(14.5783602095451,2.48246197961092,3.16207056797737));
#85521=CARTESIAN_POINT('Ctrl Pts',(14.5282544826983,2.47342940167856,3.16546659467556));
#85522=CARTESIAN_POINT('Ctrl Pts',(14.4008692382386,2.44645437464517,3.17426536022568));
#85523=CARTESIAN_POINT('Ctrl Pts',(14.3241008378071,2.42636680393794,3.17972434738033));
#85524=CARTESIAN_POINT('Ctrl Pts',(14.0724453984637,2.34764626657905,3.19792228713017));
#85525=CARTESIAN_POINT('Ctrl Pts',(13.9030286189375,2.27342801338589,3.21062075383624));
#85526=CARTESIAN_POINT('Ctrl Pts',(13.7014713474306,2.15730188918366,3.22586865793446));
#85527=CARTESIAN_POINT('Ctrl Pts',(13.660416700625,2.13205187680984,3.22898647946852));
#85528=CARTESIAN_POINT('Ctrl Pts',(13.5900472659546,2.08593657995908,3.2343558114026));
#85529=CARTESIAN_POINT('Ctrl Pts',(13.5604089664217,2.06559337708123,3.23662554462106));
#85530=CARTESIAN_POINT('Ctrl Pts',(13.4983193755591,2.02099038091255,3.24140302932744));
#85531=CARTESIAN_POINT('Ctrl Pts',(13.4659973156161,1.99656777307702,3.24390371683415));
#85532=CARTESIAN_POINT('Ctrl Pts',(13.3735808157404,1.92316791501497,3.25110849738315));
#85533=CARTESIAN_POINT('Ctrl Pts',(13.3151397883925,1.87218104358476,3.25573327928046));
#85534=CARTESIAN_POINT('Ctrl Pts',(13.1750323971919,1.73806103147935,3.26712843159783));
#85535=CARTESIAN_POINT('Ctrl Pts',(13.09660867849,1.6518068151793,3.27379219278394));
#85536=CARTESIAN_POINT('Ctrl Pts',(12.9494462482203,1.46549394149441,3.28745594219608));
#85537=CARTESIAN_POINT('Ctrl Pts',(12.8814051859582,1.36528142804665,3.29444293075157));
#85538=CARTESIAN_POINT('Ctrl Pts',(12.8040119871058,1.23149179491109,3.30382294321753));
#85539=CARTESIAN_POINT('Ctrl Pts',(12.7877711928948,1.20207272920697,3.30588890254683));
#85540=CARTESIAN_POINT('Ctrl Pts',(12.7624275389304,1.15391047610687,3.30929091677925));
#85541=CARTESIAN_POINT('Ctrl Pts',(12.7529594182019,1.13536271968924,3.31060581369784));
#85542=CARTESIAN_POINT('Ctrl Pts',(12.7332240052087,1.09548756703211,3.31344662332477));
#85543=CARTESIAN_POINT('Ctrl Pts',(12.7230256448046,1.07412946294541,3.3149760349355));
#85544=CARTESIAN_POINT('Ctrl Pts',(12.6929105177186,1.00870357358768,3.31967760203572));
#85545=CARTESIAN_POINT('Ctrl Pts',(12.6739619501597,0.964204908918892,3.32289774862161));
#85546=CARTESIAN_POINT('Ctrl Pts',(12.6502414493595,0.903723990875261,3.32727933563373));
#85547=CARTESIAN_POINT('Ctrl Pts',(12.6443289208352,0.888198154170151,3.32840455789558));
#85548=CARTESIAN_POINT('Ctrl Pts',(12.6385710144774,0.872616408471391,3.32953357812844));
#85549=CARTESIAN_POINT('Origin',(15.,0.,3.));
#85550=CARTESIAN_POINT('',(12.6421214752944,0.871321765791503,4.3311309048973));
#85551=CARTESIAN_POINT('',(12.6385710119932,0.872616401748849,4.05617650648277));
#85552=CARTESIAN_POINT('',(12.6385710119932,0.872616401748847,3.));
#85553=CARTESIAN_POINT('',(12.4825008631916,-0.00208474671008541,3.11258330249198));
#85554=CARTESIAN_POINT('Ctrl Pts',(12.6385710119932,0.872616401748848,4.05617650648277));
#85555=CARTESIAN_POINT('Ctrl Pts',(12.6673543993352,0.950508503142112,4.05093727502692));
#85556=CARTESIAN_POINT('Ctrl Pts',(12.7000132622957,1.02702225238975,4.04569804357108));
#85557=CARTESIAN_POINT('Ctrl Pts',(12.7363857616833,1.10175170981944,4.04045881211524));
#85558=CARTESIAN_POINT('Ctrl Pts',(12.7727499931487,1.1764641803124,4.03522077160199));
#85559=CARTESIAN_POINT('Ctrl Pts',(12.8128259822694,1.24939275031694,4.02998273108873));
#85560=CARTESIAN_POINT('Ctrl Pts',(12.8564046387866,1.32015346736063,4.02474469057549));
#85561=CARTESIAN_POINT('Ctrl Pts',(12.8999865129388,1.3909194090299,4.01950626331092));
#85562=CARTESIAN_POINT('Ctrl Pts',(12.9470713250003,1.45951678803023,4.01426783604636));
#85563=CARTESIAN_POINT('Ctrl Pts',(12.99740584606,1.52558936303496,4.00902940878179));
#85564=CARTESIAN_POINT('Ctrl Pts',(13.0477923412206,1.59173016284064,4.00378557245519));
#85565=CARTESIAN_POINT('Ctrl Pts',(13.1014349655593,1.65534058553694,3.99854173612859));
#85566=CARTESIAN_POINT('Ctrl Pts',(13.1580395801034,1.71609675179873,3.99329789980198));
#85567=CARTESIAN_POINT('Ctrl Pts',(13.2146748413793,1.77688581251547,3.98805122437034));
#85568=CARTESIAN_POINT('Ctrl Pts',(13.2742749555559,1.83481721791559,3.9828045489387));
#85569=CARTESIAN_POINT('Ctrl Pts',(13.3365099735538,1.88960503331095,3.97755787350706));
#85570=CARTESIAN_POINT('Ctrl Pts',(13.3988511407322,1.94448629580235,3.97230224925022));
#85571=CARTESIAN_POINT('Ctrl Pts',(13.4638358265541,1.99621297218007,3.96704662499338));
#85572=CARTESIAN_POINT('Ctrl Pts',(13.5311024033621,2.04454055978144,3.96179100073653));
#85573=CARTESIAN_POINT('Ctrl Pts',(13.5787221749002,2.07875292481873,3.95807040667218));
#85574=CARTESIAN_POINT('Ctrl Pts',(13.6274848972943,2.11126270130169,3.95434981260783));
#85575=CARTESIAN_POINT('Ctrl Pts',(13.6772548532223,2.14199708839114,3.95062921854348));
#85576=CARTESIAN_POINT('Ctrl Pts',(13.7475729445644,2.18542054333301,3.94537253168521));
#85577=CARTESIAN_POINT('Ctrl Pts',(13.8201605534495,2.22545734514497,3.94011584482692));
#85578=CARTESIAN_POINT('Ctrl Pts',(13.8946580326627,2.26186325520417,3.93485915796864));
#85579=CARTESIAN_POINT('Ctrl Pts',(13.9690503549056,2.29821777647488,3.92960989119047));
#85580=CARTESIAN_POINT('Ctrl Pts',(14.0453467816793,2.33095138554809,3.9243606244123));
#85581=CARTESIAN_POINT('Ctrl Pts',(14.1231602579543,2.35986404624701,3.91911135763412));
#85582=CARTESIAN_POINT('Ctrl Pts',(14.2012979437543,2.38889717142634,3.91384021980777));
#85583=CARTESIAN_POINT('Ctrl Pts',(14.2809649492097,2.41407718758061,3.90856908198142));
#85584=CARTESIAN_POINT('Ctrl Pts',(14.3617459691189,2.43524907187419,3.90329794415507));
#85585=CARTESIAN_POINT('Ctrl Pts',(14.4420491594968,2.45629572190405,3.89805798574834));
#85586=CARTESIAN_POINT('Ctrl Pts',(14.5234527709189,2.47338140800351,3.89281802734161));
#85587=CARTESIAN_POINT('Ctrl Pts',(14.6055321909212,2.48640330549984,3.88757806893488));
#85588=CARTESIAN_POINT('Ctrl Pts',(14.687584861771,2.49942095924395,3.88233981819673));
#85589=CARTESIAN_POINT('Ctrl Pts',(14.7703124487109,2.50837738253097,3.87710156745857));
#85590=CARTESIAN_POINT('Ctrl Pts',(14.8532808396168,2.51322098868692,3.87186331672041));
#85591=CARTESIAN_POINT('Ctrl Pts',(14.9362471777384,2.5180644750035,3.86662519558582));
#85592=CARTESIAN_POINT('Ctrl Pts',(15.0194538475891,2.51879532071958,3.86138707445122));
#85593=CARTESIAN_POINT('Ctrl Pts',(15.102463704417,2.51541396976266,3.85614895331663));
#85594=CARTESIAN_POINT('Ctrl Pts',(15.1863814109029,2.51199563815757,3.85085354469038));
#85595=CARTESIAN_POINT('Ctrl Pts',(15.2700974917501,2.5043746142835,3.84555813606413));
#85596=CARTESIAN_POINT('Ctrl Pts',(15.3531643149952,2.49260530702595,3.84026272743787));
#85597=CARTESIAN_POINT('Ctrl Pts',(15.435450056159,2.48094666723647,3.83501711184125));
#85598=CARTESIAN_POINT('Ctrl Pts',(15.517098252225,2.46521757867526,3.82977149624463));
#85599=CARTESIAN_POINT('Ctrl Pts',(15.5976845977134,2.44552231060283,3.82452588064801));
#85600=CARTESIAN_POINT('Ctrl Pts',(15.6794183695281,2.42554661203124,3.81920557550695));
#85601=CARTESIAN_POINT('Ctrl Pts',(15.7600593435452,2.40149104209609,3.81388527036588));
#85602=CARTESIAN_POINT('Ctrl Pts',(15.8391831363984,2.37351593918905,3.80856496522481));
#85603=CARTESIAN_POINT('Ctrl Pts',(15.9183069292517,2.34554083628201,3.80324466008374));
#85604=CARTESIAN_POINT('Ctrl Pts',(15.9959131139442,2.31364644507584,3.79792435494268));
#85605=CARTESIAN_POINT('Ctrl Pts',(16.0716023793666,2.27804183248152,3.79260404980161));
#85606=CARTESIAN_POINT('Ctrl Pts',(16.1463865469486,2.24286298248101,3.78734736526337));
#85607=CARTESIAN_POINT('Ctrl Pts',(16.2195737593306,2.2039331554168,3.78209068072513));
#85608=CARTESIAN_POINT('Ctrl Pts',(16.2907629773018,2.16142017812991,3.7768339961869));
#85609=CARTESIAN_POINT('Ctrl Pts',(16.3618517072413,2.11896721056818,3.77158473178751));
#85610=CARTESIAN_POINT('Ctrl Pts',(16.4309476521906,2.07294137382628,3.76633546738813));
#85611=CARTESIAN_POINT('Ctrl Pts',(16.4976718256376,2.02355759806615,3.76108620298875));
#85612=CARTESIAN_POINT('Ctrl Pts',(16.5646740429046,1.97396803701193,3.75581506457504));
#85613=CARTESIAN_POINT('Ctrl Pts',(16.6292842504876,1.92099268733259,3.75054392616134));
#85614=CARTESIAN_POINT('Ctrl Pts',(16.6911457330465,1.86489473150598,3.74527278774764));
#85615=CARTESIAN_POINT('Ctrl Pts',(16.7526412611842,1.80912863476358,3.74003283184569));
#85616=CARTESIAN_POINT('Ctrl Pts',(16.8114201504743,1.75027708761682,3.73479287594374));
#85617=CARTESIAN_POINT('Ctrl Pts',(16.8671643238952,1.68863958190404,3.72955292004179));
#85618=CARTESIAN_POINT('Ctrl Pts',(16.9228903301959,1.62702216395834,3.72431467185031));
#85619=CARTESIAN_POINT('Ctrl Pts',(16.9755832758802,1.56262093247153,3.71907642365883));
#85620=CARTESIAN_POINT('Ctrl Pts',(17.0249628122788,1.49577132573392,3.71383817546735));
#85621=CARTESIAN_POINT('Ctrl Pts',(17.0743411265767,1.42892337346617,3.70860005691797));
#85622=CARTESIAN_POINT('Ctrl Pts',(17.1204059215362,1.35962753796808,3.70336193836859));
#85623=CARTESIAN_POINT('Ctrl Pts',(17.1629187734376,1.28825022007032,3.69812381981922));
#85624=CARTESIAN_POINT('Ctrl Pts',(17.2058966185215,1.21609219787433,3.69282840825595));
#85625=CARTESIAN_POINT('Ctrl Pts',(17.2452440836424,1.14180728564829,3.68753299669267));
#85626=CARTESIAN_POINT('Ctrl Pts',(17.2807622175225,1.06580014877178,3.6822375851294));
#85627=CARTESIAN_POINT('Ctrl Pts',(17.315946335045,0.990507791199236,3.67699197218698));
#85628=CARTESIAN_POINT('Ctrl Pts',(17.3473727228792,0.913525920142375,3.67174635924456));
#85629=CARTESIAN_POINT('Ctrl Pts',(17.3748969365347,0.835266897966168,3.66650074630214));
#85630=CARTESIAN_POINT('Ctrl Pts',(17.4028130971071,0.755893461302154,3.66118043542845));
#85631=CARTESIAN_POINT('Ctrl Pts',(17.4267149356507,0.675206685676165,3.65586012455475));
#85632=CARTESIAN_POINT('Ctrl Pts',(17.446504929017,0.593649629239103,3.65053981368105));
#85633=CARTESIAN_POINT('Ctrl Pts',(17.4662949223832,0.512092572802039,3.64521950280735));
#85634=CARTESIAN_POINT('Ctrl Pts',(17.4819730422611,0.42966572687241,3.63989919193365));
#85635=CARTESIAN_POINT('Ctrl Pts',(17.4934962775776,0.346817767288341,3.63457888105995));
#85636=CARTESIAN_POINT('Ctrl Pts',(17.5048817109381,0.26496055470899,3.62932219374546));
#85637=CARTESIAN_POINT('Ctrl Pts',(17.5122529109554,0.182391959997753,3.62406550643097));
#85638=CARTESIAN_POINT('Ctrl Pts',(17.5155313797586,0.0995395773032683,
3.61880881911649));
#85639=CARTESIAN_POINT('Ctrl Pts',(17.5188052208284,0.0168041451609522,
3.61355955189619));
#85640=CARTESIAN_POINT('Ctrl Pts',(17.51799778788,-0.0662138223184987,3.6083102846759));
#85641=CARTESIAN_POINT('Ctrl Pts',(17.5130820840236,-0.149079471959533,
3.60306101745561));
#85642=CARTESIAN_POINT('Ctrl Pts',(17.5081458994284,-0.232290372203708,
3.59778987974155));
#85643=CARTESIAN_POINT('Ctrl Pts',(17.4990670668675,-0.315347216186424,
3.59251874202749));
#85644=CARTESIAN_POINT('Ctrl Pts',(17.4858711721179,-0.397807447936076,
3.58724760431343));
#85645=CARTESIAN_POINT('Ctrl Pts',(17.4727533313952,-0.479779925480137,
3.58200764550263));
#85646=CARTESIAN_POINT('Ctrl Pts',(17.4555670725052,-0.561162369073261,
3.57676768669183));
#85647=CARTESIAN_POINT('Ctrl Pts',(17.4343895011345,-0.641524751483474,
3.57152772788102));
#85648=CARTESIAN_POINT('Ctrl Pts',(17.4132188314588,-0.721860944079876,
3.56628947675411));
#85649=CARTESIAN_POINT('Ctrl Pts',(17.3880595501687,-0.801177290203249,
3.56105122562719));
#85650=CARTESIAN_POINT('Ctrl Pts',(17.3590394817709,-0.879055728293861,
3.55581297450028));
#85651=CARTESIAN_POINT('Ctrl Pts',(17.3300201314689,-0.956932239297852,
3.55057485299286));
#85652=CARTESIAN_POINT('Ctrl Pts',(17.2971403460322,-1.03337048130383,3.54533673148544));
#85653=CARTESIAN_POINT('Ctrl Pts',(17.2605767866301,-1.10797059606703,3.54009860997801));
#85654=CARTESIAN_POINT('Ctrl Pts',(17.2236133504537,-1.18338657377524,3.53480320183969));
#85655=CARTESIAN_POINT('Ctrl Pts',(17.1828852681956,-1.25692353330891,3.52950779370137));
#85656=CARTESIAN_POINT('Ctrl Pts',(17.1386228133881,-1.328193778052,3.52421238556305));
#85657=CARTESIAN_POINT('Ctrl Pts',(17.0947765541762,-1.39879387555417,3.51896676963698));
#85658=CARTESIAN_POINT('Ctrl Pts',(17.0474624264169,-1.46716935843424,3.51372115371091));
#85659=CARTESIAN_POINT('Ctrl Pts',(16.9969469265273,-1.53297397976387,3.50847553778484));
#85660=CARTESIAN_POINT('Ctrl Pts',(16.9457121750204,-1.59971554283263,3.5031552335404));
#85661=CARTESIAN_POINT('Ctrl Pts',(16.8911844897076,-1.66381208525609,3.49783492929595));
#85662=CARTESIAN_POINT('Ctrl Pts',(16.8336817078274,-1.72493989587443,3.49251462505151));
#85663=CARTESIAN_POINT('Ctrl Pts',(16.7761789259471,-1.78606770649277,3.48719432080706));
#85664=CARTESIAN_POINT('Ctrl Pts',(16.7157014435654,-1.84422649320658,3.48187401656262));
#85665=CARTESIAN_POINT('Ctrl Pts',(16.6526015810124,-1.89913513590667,3.47655371231817));
#85666=CARTESIAN_POINT('Ctrl Pts',(16.5902562391359,-1.95338720497005,3.47129702595489));
#85667=CARTESIAN_POINT('Ctrl Pts',(16.5251222113034,-2.00466549670962,3.46604033959161));
#85668=CARTESIAN_POINT('Ctrl Pts',(16.4575147759546,-2.05267068178846,3.46078365322833));
#85669=CARTESIAN_POINT('Ctrl Pts',(16.3900027722482,-2.10060810488778,3.45553438696921));
#85670=CARTESIAN_POINT('Ctrl Pts',(16.3200246688988,-2.14528133377571,3.4502851207101));
#85671=CARTESIAN_POINT('Ctrl Pts',(16.2479299576488,-2.18643021173846,3.44503585445098));
#85672=CARTESIAN_POINT('Ctrl Pts',(16.1755348551851,-2.22775054140939,3.43976471649788));
#85673=CARTESIAN_POINT('Ctrl Pts',(16.1010058210992,-2.26551677418808,3.43449357854477));
#85674=CARTESIAN_POINT('Ctrl Pts',(16.0247275232926,-2.29950858946136,3.42922244059167));
#85675=CARTESIAN_POINT('Ctrl Pts',(15.9489004310018,-2.33329933450914,3.42398248275908));
#85676=CARTESIAN_POINT('Ctrl Pts',(15.8713451381114,-2.36336000218641,3.41874252492649));
#85677=CARTESIAN_POINT('Ctrl Pts',(15.7924639613833,-2.38952026982586,3.41350256709391));
#85678=CARTESIAN_POINT('Ctrl Pts',(15.7136084918173,-2.41567201190487,3.4082643169494));
#85679=CARTESIAN_POINT('Ctrl Pts',(15.633428433952,-2.43792573352404,3.4030260668049));
#85680=CARTESIAN_POINT('Ctrl Pts',(15.5523437876966,-2.45616013121965,3.39778781666039));
#85681=CARTESIAN_POINT('Ctrl Pts',(15.4712611479092,-2.4743940776987,3.39254969613822));
#85682=CARTESIAN_POINT('Ctrl Pts',(15.3892744143518,-2.48860879789434,3.38731157561605));
#85683=CARTESIAN_POINT('Ctrl Pts',(15.3068150171882,-2.49873383841253,3.38207345509388));
#85684=CARTESIAN_POINT('Ctrl Pts',(15.2234537703064,-2.50896961542955,3.37677804580076));
#85685=CARTESIAN_POINT('Ctrl Pts',(15.1396099329018,-2.51502563259169,3.37148263650765));
#85686=CARTESIAN_POINT('Ctrl Pts',(15.0557340353218,-2.51688298641529,3.36618722721453));
#85687=CARTESIAN_POINT('Ctrl Pts',(14.9726468483965,-2.51872287497422,3.36094161227058));
#85688=CARTESIAN_POINT('Ctrl Pts',(14.889528666218,-2.51644280600452,3.35569599732663));
#85689=CARTESIAN_POINT('Ctrl Pts',(14.806815086913,-2.51007685925263,3.35045038238268));
#85690=CARTESIAN_POINT('Ctrl Pts',(14.7229237613685,-2.50362026874055,3.34513007591498));
#85691=CARTESIAN_POINT('Ctrl Pts',(14.63944913927,-2.49296059172656,3.33980976944728));
#85692=CARTESIAN_POINT('Ctrl Pts',(14.5568359887859,-2.47818722237942,3.33448946297957));
#85693=CARTESIAN_POINT('Ctrl Pts',(14.4742228383017,-2.46341385303227,3.32916915651187));
#85694=CARTESIAN_POINT('Ctrl Pts',(14.392471620456,-2.44452696354054,3.32384885004417));
#85695=CARTESIAN_POINT('Ctrl Pts',(14.3120102652849,-2.42166809759857,3.31852854357646));
#85696=CARTESIAN_POINT('Ctrl Pts',(14.2325110658525,-2.39908257764982,3.31327185725769));
#85697=CARTESIAN_POINT('Ctrl Pts',(14.1539793922194,-2.37253675295542,3.30801517093892));
#85698=CARTESIAN_POINT('Ctrl Pts',(14.0768381915538,-2.3421311930433,3.30275848462015));
#85699=CARTESIAN_POINT('Ctrl Pts',(13.9998058800514,-2.31176855229686,3.29750921841111));
#85700=CARTESIAN_POINT('Ctrl Pts',(13.9241605683303,-2.27755716605228,3.29225995220207));
#85701=CARTESIAN_POINT('Ctrl Pts',(13.8503110814322,-2.239647659906,3.28701068599304));
#85702=CARTESIAN_POINT('Ctrl Pts',(13.7761538909645,-2.20158019883205,3.28173954802811));
#85703=CARTESIAN_POINT('Ctrl Pts',(13.7038079777237,-2.15978385808111,3.27646841006318));
#85704=CARTESIAN_POINT('Ctrl Pts',(13.6336680148729,-2.11446048826138,3.27119727209825));
#85705=CARTESIAN_POINT('Ctrl Pts',(13.563942948726,-2.06940521833771,3.26595731432901));
#85706=CARTESIAN_POINT('Ctrl Pts',(13.4963981989511,-2.02086478354645,3.26071735655978));
#85707=CARTESIAN_POINT('Ctrl Pts',(13.4313962005976,-1.96908312940322,3.25547739879054));
#85708=CARTESIAN_POINT('Ctrl Pts',(13.3664153862802,-1.9173183508093,3.25023914871426));
#85709=CARTESIAN_POINT('Ctrl Pts',(13.3039760379141,-1.862314737904,3.24500089863797));
#85710=CARTESIAN_POINT('Ctrl Pts',(13.2444091909891,-1.80435782518783,3.23976264856169));
#85711=CARTESIAN_POINT('Ctrl Pts',(13.1848438181212,-1.74640234668875,3.23452452811252));
#85712=CARTESIAN_POINT('Ctrl Pts',(13.1281511350965,-1.68549403602229,3.22928640766336));
#85713=CARTESIAN_POINT('Ctrl Pts',(13.0746258285682,-1.6219557792934,3.22404828721419));
#85714=CARTESIAN_POINT('Ctrl Pts',(13.020515119927,-1.55772260959435,3.21875287784924));
#85715=CARTESIAN_POINT('Ctrl Pts',(12.9696418177184,-1.49080197138715,3.21345746848428));
#85716=CARTESIAN_POINT('Ctrl Pts',(12.9222678633734,-1.42156090915204,3.20816205911932));
#85717=CARTESIAN_POINT('Ctrl Pts',(12.8753393821638,-1.35297094378045,3.2029164442595));
#85718=CARTESIAN_POINT('Ctrl Pts',(12.8318449052164,-1.28210444049809,3.19767082939967));
#85719=CARTESIAN_POINT('Ctrl Pts',(12.7919938375189,-1.20934487903391,3.19242521453984));
#85720=CARTESIAN_POINT('Ctrl Pts',(12.7515753346643,-1.1355493018347,3.18710490792232));
#85721=CARTESIAN_POINT('Ctrl Pts',(12.7149050271858,-1.05980677523672,3.1817846013048));
#85722=CARTESIAN_POINT('Ctrl Pts',(12.6821509971805,-0.982538676149113,
3.17646429468728));
#85723=CARTESIAN_POINT('Ctrl Pts',(12.6493969671752,-0.905270577061505,
3.17114398806976));
#85724=CARTESIAN_POINT('Ctrl Pts',(12.6205593222554,-0.826477385704819,
3.16582368145224));
#85725=CARTESIAN_POINT('Ctrl Pts',(12.5957532652842,-0.746594862430913,
3.16050337483472));
#85726=CARTESIAN_POINT('Ctrl Pts',(12.5660861567849,-0.651058377615517,
3.15414048879223));
#85727=CARTESIAN_POINT('Ctrl Pts',(12.542095602325,-0.553681574571601,3.14777760274975));
#85728=CARTESIAN_POINT('Ctrl Pts',(12.5239729173674,-0.455078164791567,
3.14141471670727));
#85729=CARTESIAN_POINT('Ctrl Pts',(12.5060754715587,-0.357700254883325,
3.13513091227105));
#85730=CARTESIAN_POINT('Ctrl Pts',(12.4939009850906,-0.25912605532082,3.12884710783484));
#85731=CARTESIAN_POINT('Ctrl Pts',(12.4875874665127,-0.159967220317441,
3.12256330339863));
#85732=CARTESIAN_POINT('Ctrl Pts',(12.4842450687784,-0.107472203257753,
3.11923663642975));
#85733=CARTESIAN_POINT('Ctrl Pts',(12.4825445281381,-0.0548136775673956,
3.11590996946086));
#85734=CARTESIAN_POINT('Ctrl Pts',(12.4825008631916,-0.00208474671008541,
3.11258330249198));
#85735=CARTESIAN_POINT('Ctrl Pts',(12.4841498434241,-0.00208338118583777,
3.11258330249198));
#85736=CARTESIAN_POINT('Ctrl Pts',(12.4865054906647,0.294763270002047,3.09384311542301));
#85737=CARTESIAN_POINT('Ctrl Pts',(12.5399868199015,0.592359670770662,3.07510292835405));
#85738=CARTESIAN_POINT('Ctrl Pts',(12.6408521577454,0.87179739374149,3.05636274128509));
#85739=CARTESIAN_POINT('',(12.4862285524092,0.000445657771908455,3.38754588178119));
#85740=CARTESIAN_POINT('Ctrl Pts',(12.6385710144774,0.872616408471391,3.32953357812844));
#85741=CARTESIAN_POINT('Ctrl Pts',(12.619021003094,0.819711187918733,3.33336697815837));
#85742=CARTESIAN_POINT('Ctrl Pts',(12.6012535156701,0.766161406554403,3.33724378078027));
#85743=CARTESIAN_POINT('Ctrl Pts',(12.5333054375905,0.535738690251715,3.35380928062876));
#85744=CARTESIAN_POINT('Ctrl Pts',(12.5007720780434,0.354226854504134,3.36651667217454));
#85745=CARTESIAN_POINT('Ctrl Pts',(12.4860719888631,0.138021323217801,3.38079977453777));
#85746=CARTESIAN_POINT('Ctrl Pts',(12.4844858769325,0.105227315747329,3.38294529035555));
#85747=CARTESIAN_POINT('Ctrl Pts',(12.4828528391001,0.0484748116459329,
3.38662256013421));
#85748=CARTESIAN_POINT('Ctrl Pts',(12.4825056181578,0.0245301016561651,
3.38816309378582));
#85749=CARTESIAN_POINT('Ctrl Pts',(12.4825000676272,0.000583526462428343,
3.38969315734209));
#85750=CARTESIAN_POINT('Ctrl Pts',(12.4864528653038,0.000437363323397832,
3.38741669750802));
#85751=CARTESIAN_POINT('Ctrl Pts',(12.4871507384439,-0.445065060869901,
3.41547689838276));
#85752=CARTESIAN_POINT('Ctrl Pts',(12.811943456554,-1.72782232442595,3.49621215550473));
#85753=CARTESIAN_POINT('Ctrl Pts',(14.8545655179616,-2.96733750069494,3.62962246887397));
#85754=CARTESIAN_POINT('Ctrl Pts',(17.4060396764084,-1.74276220584388,3.78764763761569));
#85755=CARTESIAN_POINT('Ctrl Pts',(17.7740900564321,1.06333051391069,3.94567280635744));
#85756=CARTESIAN_POINT('Ctrl Pts',(15.6247197032598,2.9044718341732,4.10369797509916));
#85757=CARTESIAN_POINT('Ctrl Pts',(13.4161781540431,2.25841240405204,4.23218400794579));
#85758=CARTESIAN_POINT('Ctrl Pts',(12.7683211668134,1.21621823547935,4.30799498454517));
#85759=CARTESIAN_POINT('Ctrl Pts',(12.6421214752944,0.871321765791516,4.3311309048973));
#85760=CARTESIAN_POINT('Origin',(15.,0.,3.));
#85761=CARTESIAN_POINT('',(12.6385710119932,0.872616401748846,5.33098034507765));
#85762=CARTESIAN_POINT('',(12.6385710119932,0.872616401748849,5.05624489442998));
#85763=CARTESIAN_POINT('',(12.6385710119932,0.872616401748847,3.));
#85764=CARTESIAN_POINT('',(12.4825004940191,0.00157714490144886,5.38741669754798));
#85765=CARTESIAN_POINT('Ctrl Pts',(12.6385710119932,0.872616401748844,5.33098034507765));
#85766=CARTESIAN_POINT('Ctrl Pts',(12.6098178284995,0.794806036434478,5.33622205618864));
#85767=CARTESIAN_POINT('Ctrl Pts',(12.5849432520214,0.715650777905113,5.34146376729964));
#85768=CARTESIAN_POINT('Ctrl Pts',(12.5640499918729,0.635573605419081,5.34670547841063));
#85769=CARTESIAN_POINT('Ctrl Pts',(12.543122884809,0.555366708550572,5.35195568105193));
#85770=CARTESIAN_POINT('Ctrl Pts',(12.5261900580931,0.47423536920686,5.35720588369323));
#85771=CARTESIAN_POINT('Ctrl Pts',(12.5133028738199,0.392611325164924,5.36245608633453));
#85772=CARTESIAN_POINT('Ctrl Pts',(12.508849203175,0.364402943786497,5.36427049923404));
#85773=CARTESIAN_POINT('Ctrl Pts',(12.5048782541387,0.336135744403197,5.36608491213355));
#85774=CARTESIAN_POINT('Ctrl Pts',(12.5013907003247,0.307827577673285,5.36789932503306));
#85775=CARTESIAN_POINT('Ctrl Pts',(12.4888856659904,0.206325316840848,5.37440511585805));
#85776=CARTESIAN_POINT('Ctrl Pts',(12.4825646917813,0.104052047516512,5.38091090668304));
#85777=CARTESIAN_POINT('Ctrl Pts',(12.4825004940195,0.00157714553074645,
5.38741669750803));
#85778=CARTESIAN_POINT('',(16.9134659966651,1.63598720337493,6.));
#85779=CARTESIAN_POINT('Ctrl Pts',(12.4825004940191,0.00157714490144911,
5.38741669754798));
#85780=CARTESIAN_POINT('Ctrl Pts',(12.4824492998181,-0.0801410127544445,
5.39260471168613));
#85781=CARTESIAN_POINT('Ctrl Pts',(12.4863811899288,-0.162011329145106,
5.39779272582428));
#85782=CARTESIAN_POINT('Ctrl Pts',(12.49431418367,-0.243607963422187,5.40298073996243));
#85783=CARTESIAN_POINT('Ctrl Pts',(12.5022364492358,-0.32509425058011,5.40816173809533));
#85784=CARTESIAN_POINT('Ctrl Pts',(12.5141490234632,-0.40630712270579,5.41334273622823));
#85785=CARTESIAN_POINT('Ctrl Pts',(12.5300179018197,-0.48682099859071,5.41852373436114));
#85786=CARTESIAN_POINT('Ctrl Pts',(12.5458749086248,-0.567274641824679,
5.42370085657515));
#85787=CARTESIAN_POINT('Ctrl Pts',(12.5656822570989,-0.647029863143335,
5.42887797878917));
#85788=CARTESIAN_POINT('Ctrl Pts',(12.5893542961562,-0.725667651572945,
5.43405510100318));
#85789=CARTESIAN_POINT('Ctrl Pts',(12.6130161888524,-0.804271734101949,
5.43923000418777));
#85790=CARTESIAN_POINT('Ctrl Pts',(12.6405393482842,-0.881758881203542,
5.44440490737236));
#85791=CARTESIAN_POINT('Ctrl Pts',(12.671787708573,-0.957723225179621,5.44957981055694));
#85792=CARTESIAN_POINT('Ctrl Pts',(12.7030326574948,-1.03367927616822,5.45475414880007));
#85793=CARTESIAN_POINT('Ctrl Pts',(12.7380018182631,-1.1081124165419,5.4599284870432));
#85794=CARTESIAN_POINT('Ctrl Pts',(12.7765107980518,-1.18063627710643,5.46510282528633));
#85795=CARTESIAN_POINT('Ctrl Pts',(12.815052983583,-1.25322267395869,5.47028162528732));
#85796=CARTESIAN_POINT('Ctrl Pts',(12.8571408635482,-1.32389608247715,5.47546042528831));
#85797=CARTESIAN_POINT('Ctrl Pts',(12.9025441613878,-1.39229495979536,5.48063922528931));
#85798=CARTESIAN_POINT('Ctrl Pts',(12.9479661610744,-1.46072201095558,5.4858201584641));
#85799=CARTESIAN_POINT('Ctrl Pts',(12.9967060167826,-1.5268722833105,5.49100109163889));
#85800=CARTESIAN_POINT('Ctrl Pts',(13.0484916987446,-1.59041554322488,5.49618202481368));
#85801=CARTESIAN_POINT('Ctrl Pts',(13.1003655936019,-1.65406704415733,5.50137178330657));
#85802=CARTESIAN_POINT('Ctrl Pts',(13.1552953616705,-1.71510230855825,5.50656154179945));
#85803=CARTESIAN_POINT('Ctrl Pts',(13.2129707216408,-1.77322660940077,5.51175130029234));
#85804=CARTESIAN_POINT('Ctrl Pts',(13.2654743874119,-1.82613895994677,5.51647569811982));
#85805=CARTESIAN_POINT('Ctrl Pts',(13.3202526773605,-1.87663928457784,5.52120009594731));
#85806=CARTESIAN_POINT('Ctrl Pts',(13.3770488316674,-1.9245352049801,5.5259244937748));
#85807=CARTESIAN_POINT('Ctrl Pts',(13.4403118562222,-1.97788460557705,5.53118681653968));
#85808=CARTESIAN_POINT('Ctrl Pts',(13.506321281188,-2.02820671259872,5.53644913930457));
#85809=CARTESIAN_POINT('Ctrl Pts',(13.5747557907899,-2.07520726533838,5.54171146206945));
#85810=CARTESIAN_POINT('Ctrl Pts',(13.6430952773156,-2.12214255660204,5.54696647796387));
#85811=CARTESIAN_POINT('Ctrl Pts',(13.7138527833007,-2.1657651971615,5.55222149385829));
#85812=CARTESIAN_POINT('Ctrl Pts',(13.7866735024611,-2.20582072262684,5.55747650975271));
#85813=CARTESIAN_POINT('Ctrl Pts',(13.8596979084428,-2.24598828739571,5.5627462244512));
#85814=CARTESIAN_POINT('Ctrl Pts',(13.9347967246319,-2.28256845733183,5.56801593914969));
#85815=CARTESIAN_POINT('Ctrl Pts',(14.0115823135293,-2.31534807903085,5.57328565384819));
#85816=CARTESIAN_POINT('Ctrl Pts',(14.0880214188612,-2.34797978755551,5.57853158974178));
#85817=CARTESIAN_POINT('Ctrl Pts',(14.1661316832303,-2.37684498621441,5.58377752563537));
#85818=CARTESIAN_POINT('Ctrl Pts',(14.2455071070187,-2.40177990757704,5.58902346152897));
#85819=CARTESIAN_POINT('Ctrl Pts',(14.3248577730842,-2.42670705157173,5.59426776118024));
#85820=CARTESIAN_POINT('Ctrl Pts',(14.4054723763626,-2.44770621550424,5.59951206083151));
#85821=CARTESIAN_POINT('Ctrl Pts',(14.4869280811847,-2.46466294980128,5.60475636048278));
#85822=CARTESIAN_POINT('Ctrl Pts',(14.5683827415137,-2.48161946666491,5.61000059288727));
#85823=CARTESIAN_POINT('Ctrl Pts',(14.6506780315082,-2.49453356438589,5.61524482529175));
#85824=CARTESIAN_POINT('Ctrl Pts',(14.7333805464554,-2.50334182983299,5.62048905769623));
#85825=CARTESIAN_POINT('Ctrl Pts',(14.8167793360512,-2.51222425229856,5.62577744143126));
#85826=CARTESIAN_POINT('Ctrl Pts',(14.9005917694087,-2.51693131427674,5.63106582516628));
#85827=CARTESIAN_POINT('Ctrl Pts',(14.9843695500362,-2.51745147699691,5.63635420890131));
#85828=CARTESIAN_POINT('Ctrl Pts',(15.0675679975995,-2.51796804273158,5.64160602284979));
#85829=CARTESIAN_POINT('Ctrl Pts',(15.1507318088343,-2.51435551447981,5.64685783679827));
#85830=CARTESIAN_POINT('Ctrl Pts',(15.2334251125323,-2.50665493573393,5.65210965074675));
#85831=CARTESIAN_POINT('Ctrl Pts',(15.3169821396488,-2.49887392520094,5.65741631937505));
#85832=CARTESIAN_POINT('Ctrl Pts',(15.4000582965981,-2.48691903614563,5.66272298800334));
#85833=CARTESIAN_POINT('Ctrl Pts',(15.4822143167678,-2.47088559077594,5.66802965663164));
#85834=CARTESIAN_POINT('Ctrl Pts',(15.5643703369375,-2.45485214540624,5.67333632525993));
#85835=CARTESIAN_POINT('Ctrl Pts',(15.6456057716764,-2.43474031903382,5.67864299388823));
#85836=CARTESIAN_POINT('Ctrl Pts',(15.7254987058856,-2.41069655447515,5.68394966251653));
#85837=CARTESIAN_POINT('Ctrl Pts',(15.8038445324732,-2.38711839168426,5.68915356877214));
#85838=CARTESIAN_POINT('Ctrl Pts',(15.8811999880898,-2.35966860286573,5.69435747502775));
#85839=CARTESIAN_POINT('Ctrl Pts',(15.9571497439144,-2.3284481135994,5.69956138128336));
#85840=CARTESIAN_POINT('Ctrl Pts',(16.0329908326933,-2.29727229384249,5.70475784191768));
#85841=CARTESIAN_POINT('Ctrl Pts',(16.1074297825892,-2.26233666105182,5.70995430255201));
#85842=CARTESIAN_POINT('Ctrl Pts',(16.180065591005,-2.22379213302998,5.71515076318633));
#85843=CARTESIAN_POINT('Ctrl Pts',(16.2539297182706,-2.18459579192366,5.72043509935599));
#85844=CARTESIAN_POINT('Ctrl Pts',(16.3259286754122,-2.14166749400403,5.72571943552566));
#85845=CARTESIAN_POINT('Ctrl Pts',(16.3956613162591,-2.09521734917831,5.73100377169532));
#85846=CARTESIAN_POINT('Ctrl Pts',(16.4641153205206,-2.04961892678639,5.73619121284603));
#85847=CARTESIAN_POINT('Ctrl Pts',(16.5303850131159,-2.00062700045551,5.74137865399674));
#85848=CARTESIAN_POINT('Ctrl Pts',(16.5941168644065,-1.94848599497531,5.74656609514745));
#85849=CARTESIAN_POINT('Ctrl Pts',(16.6578303083121,-1.89636004914801,5.75175203803278));
#85850=CARTESIAN_POINT('Ctrl Pts',(16.7190070011472,-1.84108712751668,5.75693798091811));
#85851=CARTESIAN_POINT('Ctrl Pts',(16.77732537827,-1.78295281759144,5.76212392380345));
#85852=CARTESIAN_POINT('Ctrl Pts',(16.8356453429613,-1.72481692510858,5.76731000786278));
#85853=CARTESIAN_POINT('Ctrl Pts',(16.8911065044959,-1.66381982325704,5.77249609192212));
#85854=CARTESIAN_POINT('Ctrl Pts',(16.9434242521823,-1.60028385795444,5.77768217598146));
#85855=CARTESIAN_POINT('Ctrl Pts',(16.9974734936777,-1.53464512379362,5.78303989725453));
#85856=CARTESIAN_POINT('Ctrl Pts',(17.0481672504167,-1.46629693281038,5.7883976185276));
#85857=CARTESIAN_POINT('Ctrl Pts',(17.0952383407115,-1.39562980249503,5.79375533980066));
#85858=CARTESIAN_POINT('Ctrl Pts',(17.1408776398397,-1.32711219904057,5.79895009187237));
#85859=CARTESIAN_POINT('Ctrl Pts',(17.1831113188493,-1.25641515828611,5.80414484394408));
#85860=CARTESIAN_POINT('Ctrl Pts',(17.2217422455258,-1.18392045528663,5.80933959601579));
#85861=CARTESIAN_POINT('Ctrl Pts',(17.262191060096,-1.10801430828925,5.81477880188954));
#85862=CARTESIAN_POINT('Ctrl Pts',(17.2986894609775,-1.03013768849094,5.82021800776328));
#85863=CARTESIAN_POINT('Ctrl Pts',(17.3310682049762,-0.950750899946465,
5.82565721363703));
#85864=CARTESIAN_POINT('Ctrl Pts',(17.3634469489749,-0.871364111401987,
5.83109641951078));
#85865=CARTESIAN_POINT('Ctrl Pts',(17.3917059305147,-0.790467733661366,
5.83653562538452));
#85866=CARTESIAN_POINT('Ctrl Pts',(17.415736476975,-0.708536183841481,5.84197483125827));
#85867=CARTESIAN_POINT('Ctrl Pts',(17.4395912944092,-0.627203777760307,
5.84737426165907));
#85868=CARTESIAN_POINT('Ctrl Pts',(17.4593704891542,-0.54454292061888,5.85277369205987));
#85869=CARTESIAN_POINT('Ctrl Pts',(17.4749339320301,-0.46098620596046,5.85817312246068));
#85870=CARTESIAN_POINT('Ctrl Pts',(17.4904730039907,-0.377560333406624,
5.86356409785173));
#85871=CARTESIAN_POINT('Ctrl Pts',(17.501809375636,-0.293241813948646,5.86895507324279));
#85872=CARTESIAN_POINT('Ctrl Pts',(17.5088530313989,-0.208477137452827,
5.87434604863384));
#85873=CARTESIAN_POINT('Ctrl Pts',(17.5158856497004,-0.123845287840876,
5.87972857632602));
#85874=CARTESIAN_POINT('Ctrl Pts',(17.518638909606,-0.0387691001167128,
5.8851111040182));
#85875=CARTESIAN_POINT('Ctrl Pts',(17.5170742549287,0.0462973560269238,
5.89049363171038));
#85876=CARTESIAN_POINT('Ctrl Pts',(17.5155110459009,0.131285215735854,5.89587118626149));
#85877=CARTESIAN_POINT('Ctrl Pts',(17.5096378635764,0.216262932944203,5.90124874081261));
#85878=CARTESIAN_POINT('Ctrl Pts',(17.4994681446226,0.30077440718398,5.90662629536372));
#85879=CARTESIAN_POINT('Ctrl Pts',(17.4893053914714,0.3852279948445,5.91200016653053));
#85880=CARTESIAN_POINT('Ctrl Pts',(17.4748520068441,0.46921554822398,5.91737403769734));
#85881=CARTESIAN_POINT('Ctrl Pts',(17.4561733372392,0.552285059942274,5.92274790886415));
#85882=CARTESIAN_POINT('Ctrl Pts',(17.4375030019987,0.635317506301934,5.92811938222631));
#85883=CARTESIAN_POINT('Ctrl Pts',(17.4146112278296,0.717432306497981,5.93349085558846));
#85884=CARTESIAN_POINT('Ctrl Pts',(17.3876144534637,0.798187616798997,5.93886232895061));
#85885=CARTESIAN_POINT('Ctrl Pts',(17.3606154325272,0.878949647254824,5.94423424930668));
#85886=CARTESIAN_POINT('Ctrl Pts',(17.3295108558663,0.958351550047946,5.94960616966276));
#85887=CARTESIAN_POINT('Ctrl Pts',(17.2944668662793,1.03596720486042,5.95497809001883));
#85888=CARTESIAN_POINT('Ctrl Pts',(17.2594234455537,1.11358159975507,5.9603499231737));
#85889=CARTESIAN_POINT('Ctrl Pts',(17.2204409219351,1.18940941409572,5.96572175632857));
#85890=CARTESIAN_POINT('Ctrl Pts',(17.1777327734932,1.26304640344432,5.97109358948344));
#85891=CARTESIAN_POINT('Ctrl Pts',(17.1349938295841,1.33673649004879,5.97646929609379));
#85892=CARTESIAN_POINT('Ctrl Pts',(17.0885241134416,1.40823222428896,5.98184500270414));
#85893=CARTESIAN_POINT('Ctrl Pts',(17.038581909391,1.47715606782208,5.98722070931449));
#85894=CARTESIAN_POINT('Ctrl Pts',(16.9990072085316,1.53177200922393,5.99148047287632));
#85895=CARTESIAN_POINT('Ctrl Pts',(16.9572530041006,1.58477350827339,5.99574023643816));
#85896=CARTESIAN_POINT('Ctrl Pts',(16.9134659966651,1.63598720337492,6.));
#85897=CARTESIAN_POINT('',(13.0863257750576,1.63574362624191,5.99999801595942));
#85898=CARTESIAN_POINT('Origin',(15.,0.,6.));
#85899=CARTESIAN_POINT('',(12.4825005975625,0.00173456822324663,5.11258330243344));
#85900=CARTESIAN_POINT('Ctrl Pts',(13.0863257750576,1.63574362624191,5.99999801595942));
#85901=CARTESIAN_POINT('Ctrl Pts',(13.1398047889163,1.6983093050897,5.99476345326225));
#85902=CARTESIAN_POINT('Ctrl Pts',(13.1964569730435,1.75836839630831,5.98952889056507));
#85903=CARTESIAN_POINT('Ctrl Pts',(13.2560173944066,1.81558005094452,5.9842943278679));
#85904=CARTESIAN_POINT('Ctrl Pts',(13.3154940880969,1.87271127971086,5.97906712371088));
#85905=CARTESIAN_POINT('Ctrl Pts',(13.377870567159,1.92700270143622,5.97383991955386));
#85906=CARTESIAN_POINT('Ctrl Pts',(13.4428421932686,1.97814706605332,5.96861271539685));
#85907=CARTESIAN_POINT('Ctrl Pts',(13.5077407467043,2.0292339093231,5.96339139020281));
#85908=CARTESIAN_POINT('Ctrl Pts',(13.5752282830167,2.07718044289211,5.95817006500876));
#85909=CARTESIAN_POINT('Ctrl Pts',(13.644965012631,2.12171780239641,5.95294873981472));
#85910=CARTESIAN_POINT('Ctrl Pts',(13.7146592101118,2.16622799875545,5.94773059908461));
#85911=CARTESIAN_POINT('Ctrl Pts',(13.7865994867435,2.20733289832195,5.94251245835449));
#85912=CARTESIAN_POINT('Ctrl Pts',(13.8604157788461,2.2448060167634,5.93729431762437));
#85913=CARTESIAN_POINT('Ctrl Pts',(13.9342097789858,2.28226781860593,5.93207775273337));
#85914=CARTESIAN_POINT('Ctrl Pts',(14.0098782547165,2.31609980690116,5.92686118784237));
#85915=CARTESIAN_POINT('Ctrl Pts',(14.0870264325652,2.34612137690389,5.92164462295136));
#85916=CARTESIAN_POINT('Ctrl Pts',(14.16417506616,2.37614312425642,5.91642802724396));
#85917=CARTESIAN_POINT('Ctrl Pts',(14.242802984838,2.40235424144356,5.91121143153655));
#85918=CARTESIAN_POINT('Ctrl Pts',(14.3224966766949,2.42462275352488,5.90599483582915));
#85919=CARTESIAN_POINT('Ctrl Pts',(14.4022672076388,2.44691273646664,5.90077321038298));
#85920=CARTESIAN_POINT('Ctrl Pts',(14.4831051146794,2.46525239736934,5.89555158493682));
#85921=CARTESIAN_POINT('Ctrl Pts',(14.5645835897953,2.47956020288366,5.89032995949065));
#85922=CARTESIAN_POINT('Ctrl Pts',(14.6461022933234,2.49387507259865,5.88510575596849));
#85923=CARTESIAN_POINT('Ctrl Pts',(14.7282617325478,2.50415406503659,5.87988155244634));
#85924=CARTESIAN_POINT('Ctrl Pts',(14.810629266729,2.51036749807282,5.87465734892418));
#85925=CARTESIAN_POINT('Ctrl Pts',(14.8931361053126,2.51659143960108,5.86942430994813));
#85926=CARTESIAN_POINT('Ctrl Pts',(14.9758512759986,2.51873607618652,5.86419127097209));
#85927=CARTESIAN_POINT('Ctrl Pts',(15.0583417354306,2.51682388972827,5.85895823199605));
#85928=CARTESIAN_POINT('Ctrl Pts',(15.1215371250673,2.51535897646292,5.85494923581211));
#85929=CARTESIAN_POINT('Ctrl Pts',(15.1846006139742,2.51151419625709,5.85094023962817));
#85930=CARTESIAN_POINT('Ctrl Pts',(15.2473407751248,2.50532009750464,5.84693124344423));
#85931=CARTESIAN_POINT('Ctrl Pts',(15.3297418431585,2.49718495179657,5.84166594668308));
#85932=CARTESIAN_POINT('Ctrl Pts',(15.4118865717943,2.48496584586104,5.83640064992194));
#85933=CARTESIAN_POINT('Ctrl Pts',(15.493339607283,2.4686883727773,5.83113535316079));
#85934=CARTESIAN_POINT('Ctrl Pts',(15.5746805746141,2.4524332952545,5.82587730072276));
#85935=CARTESIAN_POINT('Ctrl Pts',(15.6553312924422,2.43213103240371,5.82061924828473));
#85936=CARTESIAN_POINT('Ctrl Pts',(15.7348616424701,2.40785892784982,5.81536119584669));
#85937=CARTESIAN_POINT('Ctrl Pts',(15.8145570252977,2.38353645644398,5.81009223246568));
#85938=CARTESIAN_POINT('Ctrl Pts',(15.8931269243526,2.35522770936555,5.80482326908468));
#85939=CARTESIAN_POINT('Ctrl Pts',(15.9701489144374,2.32306205982879,5.79955430570367));
#85940=CARTESIAN_POINT('Ctrl Pts',(16.0468806290134,2.29101763411754,5.79430519965204));
#85941=CARTESIAN_POINT('Ctrl Pts',(16.1220756512209,2.25514549385421,5.78905609360041));
#85942=CARTESIAN_POINT('Ctrl Pts',(16.1953332573609,2.21562285911819,5.78380698754878));
#85943=CARTESIAN_POINT('Ctrl Pts',(16.2685686428395,2.17611221247635,5.77855947366777));
#85944=CARTESIAN_POINT('Ctrl Pts',(16.3398673755929,2.13295348875128,5.77331195978675));
#85945=CARTESIAN_POINT('Ctrl Pts',(16.4088523767563,2.08637034835815,5.76806444590574));
#85946=CARTESIAN_POINT('Ctrl Pts',(16.4778370250932,2.03978744621633,5.76281695886335));
#85947=CARTESIAN_POINT('Ctrl Pts',(16.544507585392,1.98978042028937,5.75756947182095));
#85948=CARTESIAN_POINT('Ctrl Pts',(16.6085162169142,1.93661607705915,5.75232198477855));
#85949=CARTESIAN_POINT('Ctrl Pts',(16.6729782725596,1.88307512843776,5.74703732560555));
#85950=CARTESIAN_POINT('Ctrl Pts',(16.7347401635969,1.82633224283836,5.74175266643254));
#85951=CARTESIAN_POINT('Ctrl Pts',(16.793482116325,1.76669979012352,5.73646800725954));
#85952=CARTESIAN_POINT('Ctrl Pts',(16.8518959264495,1.70740045449759,5.73121286909732));
#85953=CARTESIAN_POINT('Ctrl Pts',(16.9073231858939,1.64524413625105,5.72595773093509));
#85954=CARTESIAN_POINT('Ctrl Pts',(16.9594891797343,1.58057217630327,5.72070259277287));
#85955=CARTESIAN_POINT('Ctrl Pts',(17.0120947413328,1.51535526922907,5.71540317309448));
#85956=CARTESIAN_POINT('Ctrl Pts',(17.0613835376696,1.44758051073455,5.71010375341608));
#85957=CARTESIAN_POINT('Ctrl Pts',(17.1071187672171,1.37762721766134,5.70480433373768));
#85958=CARTESIAN_POINT('Ctrl Pts',(17.1528539967647,1.30767392458814,5.69950491405929));
#85959=CARTESIAN_POINT('Ctrl Pts',(17.1950354743649,1.23554253582845,5.69420549438089));
#85960=CARTESIAN_POINT('Ctrl Pts',(17.2334747450077,1.16163540468297,5.68890607470249));
#85961=CARTESIAN_POINT('Ctrl Pts',(17.2715585648948,1.08841169820112,5.68365565914663));
#85962=CARTESIAN_POINT('Ctrl Pts',(17.3061091309926,1.01317570439733,5.67840524359078));
#85963=CARTESIAN_POINT('Ctrl Pts',(17.3369089490488,0.936302736221347,5.67315482803492));
#85964=CARTESIAN_POINT('Ctrl Pts',(17.3676647212905,0.859539701567974,5.66791192092697));
#85965=CARTESIAN_POINT('Ctrl Pts',(17.3946802284794,0.781144767706604,5.66266901381902));
#85966=CARTESIAN_POINT('Ctrl Pts',(17.4177840102534,0.701517447938976,5.65742610671107));
#85967=CARTESIAN_POINT('Ctrl Pts',(17.4410191531688,0.621437391225072,5.65215339001314));
#85968=CARTESIAN_POINT('Ctrl Pts',(17.4602977226381,0.540111307931608,5.64688067331521));
#85969=CARTESIAN_POINT('Ctrl Pts',(17.4754946440225,0.457965629077161,5.64160795661728));
#85970=CARTESIAN_POINT('Ctrl Pts',(17.4905783331584,0.376432017606484,5.63637452692701));
#85971=CARTESIAN_POINT('Ctrl Pts',(17.5016409083356,0.294091444263798,5.63114109723675));
#85972=CARTESIAN_POINT('Ctrl Pts',(17.5086106325315,0.211373944349393,5.62590766754648));
#85973=CARTESIAN_POINT('Ctrl Pts',(17.5155780170051,0.128684212532012,5.62067599470795));
#85974=CARTESIAN_POINT('Ctrl Pts',(17.5184552403201,0.04561826581733,5.61544432186942));
#85975=CARTESIAN_POINT('Ctrl Pts',(17.5172223543771,-0.0373880813133137,
5.61021264903089));
#85976=CARTESIAN_POINT('Ctrl Pts',(17.5159895085048,-0.12039173061044,5.60498114622975));
#85977=CARTESIAN_POINT('Ctrl Pts',(17.5106468268508,-0.203335321846842,
5.5997496434286));
#85978=CARTESIAN_POINT('Ctrl Pts',(17.5012264746769,-0.285783786060985,
5.59451814062746));
#85979=CARTESIAN_POINT('Ctrl Pts',(17.4916771924292,-0.369360667385267,
5.58921503773857));
#85980=CARTESIAN_POINT('Ctrl Pts',(17.4779378138276,-0.452428279455892,
5.58391193484967));
#85981=CARTESIAN_POINT('Ctrl Pts',(17.4600958703531,-0.534541447103558,
5.57860883196078));
#85982=CARTESIAN_POINT('Ctrl Pts',(17.4424697166931,-0.615661495070169,
5.57336986757732));
#85983=CARTESIAN_POINT('Ctrl Pts',(17.4208398793822,-0.69584962456979,5.56813090319387));
#85984=CARTESIAN_POINT('Ctrl Pts',(17.3953412717723,-0.774691191213783,
5.56289193881041));
#85985=CARTESIAN_POINT('Ctrl Pts',(17.3693744105736,-0.854980595602245,
5.5575567666688));
#85986=CARTESIAN_POINT('Ctrl Pts',(17.3393954443895,-0.933873015488072,
5.55222159452719));
#85987=CARTESIAN_POINT('Ctrl Pts',(17.3055976313624,-1.01095292286836,5.54688642238558));
#85988=CARTESIAN_POINT('Ctrl Pts',(17.2717998183353,-1.08803283024865,5.54155125024397));
#85989=CARTESIAN_POINT('Ctrl Pts',(17.2341834407507,-1.16329980809554,5.53621607810236));
#85990=CARTESIAN_POINT('Ctrl Pts',(17.1929892410661,-1.23636743671465,5.53088090596074));
#85991=CARTESIAN_POINT('Ctrl Pts',(17.1523913371662,-1.30837739412583,5.52562296169788));
#85992=CARTESIAN_POINT('Ctrl Pts',(17.1081686274721,-1.37851725625535,5.52036501743502));
#85993=CARTESIAN_POINT('Ctrl Pts',(17.0605182013148,-1.44639931970747,5.51510707317216));
#85994=CARTESIAN_POINT('Ctrl Pts',(17.0129349748039,-1.51418565157814,5.50985654399502));
#85995=CARTESIAN_POINT('Ctrl Pts',(16.9619338964915,-1.57972013542936,5.50460601481788));
#85996=CARTESIAN_POINT('Ctrl Pts',(16.9077573997971,-1.64264054300363,5.49935548564074));
#85997=CARTESIAN_POINT('Ctrl Pts',(16.8533715070376,-1.70580414248893,5.49408466278983));
#85998=CARTESIAN_POINT('Ctrl Pts',(16.7957858292548,-1.76633300679217,5.48881383993893));
#85999=CARTESIAN_POINT('Ctrl Pts',(16.7352890092242,-1.82389097932569,5.48354301708802));
#86000=CARTESIAN_POINT('Ctrl Pts',(16.6751319233483,-1.88112572149542,5.47830179378541));
#86001=CARTESIAN_POINT('Ctrl Pts',(16.6120966418765,-1.93542252986321,5.4730605704828));
#86002=CARTESIAN_POINT('Ctrl Pts',(16.5465054206629,-1.98648615244613,5.46781934718018));
#86003=CARTESIAN_POINT('Ctrl Pts',(16.4809355946334,-2.03753311859876,5.46257983351089));
#86004=CARTESIAN_POINT('Ctrl Pts',(16.4128118481274,-2.08534871074164,5.45734031984159));
#86005=CARTESIAN_POINT('Ctrl Pts',(16.3424895048318,-2.12967795204261,5.4521008061723));
#86006=CARTESIAN_POINT('Ctrl Pts',(16.2721689511846,-2.17400606519929,5.4468614258445));
#86007=CARTESIAN_POINT('Ctrl Pts',(16.1996503024337,-2.21484775908183,5.4416220455167));
#86008=CARTESIAN_POINT('Ctrl Pts',(16.125316673362,-2.25199214799997,5.4363826651889));
#86009=CARTESIAN_POINT('Ctrl Pts',(16.0502093959688,-2.28952312767786,5.43108875452475));
#86010=CARTESIAN_POINT('Ctrl Pts',(15.9732495593644,-2.32327916190359,5.42579484386059));
#86011=CARTESIAN_POINT('Ctrl Pts',(15.8948548793404,-2.35309179483517,5.42050093319643));
#86012=CARTESIAN_POINT('Ctrl Pts',(15.8171570581821,-2.3826394200193,5.41525408068187));
#86013=CARTESIAN_POINT('Ctrl Pts',(15.7380502635238,-2.40831338687226,5.41000722816731));
#86014=CARTESIAN_POINT('Ctrl Pts',(15.6579565276493,-2.4299998884205,5.40476037565274));
#86015=CARTESIAN_POINT('Ctrl Pts',(15.5767852706341,-2.45197814391967,5.39944293591379));
#86016=CARTESIAN_POINT('Ctrl Pts',(15.4946007979303,-2.46986074220205,5.39412549617483));
#86017=CARTESIAN_POINT('Ctrl Pts',(15.4118512759015,-2.48358305207181,5.38880805643588));
#86018=CARTESIAN_POINT('Ctrl Pts',(15.3291017538727,-2.49730536194156,5.38349061669692));
#86019=CARTESIAN_POINT('Ctrl Pts',(15.2457876724258,-2.50686739103449,5.37817317695797));
#86020=CARTESIAN_POINT('Ctrl Pts',(15.1623588078343,-2.51225911631715,5.37285573721902));
#86021=CARTESIAN_POINT('Ctrl Pts',(15.0798682633806,-2.5175902011436,5.3675981024506));
#86022=CARTESIAN_POINT('Ctrl Pts',(14.9969642259103,-2.51886382988772,5.36234046768219));
#86023=CARTESIAN_POINT('Ctrl Pts',(14.9140790773331,-2.5160333553131,5.35708283291378));
#86024=CARTESIAN_POINT('Ctrl Pts',(14.8313105765977,-2.51320686418733,5.35183259744137));
#86025=CARTESIAN_POINT('Ctrl Pts',(14.7485613688306,-2.50628775833595,5.34658236196896));
#86026=CARTESIAN_POINT('Ctrl Pts',(14.6662672594009,-2.49528128832246,5.34133212649656));
#86027=CARTESIAN_POINT('Ctrl Pts',(14.5836492740316,-2.4842315013469,5.33606122824575));
#86028=CARTESIAN_POINT('Ctrl Pts',(14.5014904461928,-2.46906207896666,5.33079032999495));
#86029=CARTESIAN_POINT('Ctrl Pts',(14.4202300646622,-2.44983123338698,5.32551943174415));
#86030=CARTESIAN_POINT('Ctrl Pts',(14.3394310705388,-2.43070957840935,5.3202784610673));
#86031=CARTESIAN_POINT('Ctrl Pts',(14.2595208004982,-2.40757260462149,5.31503749039045));
#86032=CARTESIAN_POINT('Ctrl Pts',(14.1809225467008,-2.3805290116898,5.3097965197136));
#86033=CARTESIAN_POINT('Ctrl Pts',(14.1023496903866,-2.35349415736448,5.30455724255358));
#86034=CARTESIAN_POINT('Ctrl Pts',(14.0250884437906,-2.32255534094759,5.29931796539356));
#86035=CARTESIAN_POINT('Ctrl Pts',(13.9495464172445,-2.28787095800358,5.29407868823354));
#86036=CARTESIAN_POINT('Ctrl Pts',(13.8740060750566,-2.25318734841612,5.28883952789351));
#86037=CARTESIAN_POINT('Ctrl Pts',(13.8001852951159,-2.21475853167456,5.28360036755348));
#86038=CARTESIAN_POINT('Ctrl Pts',(13.7284699269289,-2.17279026214585,5.27836120721345));
#86039=CARTESIAN_POINT('Ctrl Pts',(13.6560008852565,-2.13038093831074,5.27306698731877));
#86040=CARTESIAN_POINT('Ctrl Pts',(13.5856821914247,-2.08435755731284,5.26777276742409));
#86041=CARTESIAN_POINT('Ctrl Pts',(13.5178831491532,-2.03497810564045,5.26247854752941));
#86042=CARTESIAN_POINT('Ctrl Pts',(13.4506929680101,-1.98604210018288,5.25723187173846));
#86043=CARTESIAN_POINT('Ctrl Pts',(13.385977688935,-1.93381040068355,5.25198519594752));
#86044=CARTESIAN_POINT('Ctrl Pts',(13.3240630831332,-1.87857437986441,5.24673852015657));
#86045=CARTESIAN_POINT('Ctrl Pts',(13.2613068946155,-1.82258755590581,5.24142052821002));
#86046=CARTESIAN_POINT('Ctrl Pts',(13.2014284377852,-1.76351446736911,5.23610253626347));
#86047=CARTESIAN_POINT('Ctrl Pts',(13.1447266726257,-1.70169536954578,5.23078454431692));
#86048=CARTESIAN_POINT('Ctrl Pts',(13.0880249074662,-1.63987627172245,5.22546655237037));
#86049=CARTESIAN_POINT('Ctrl Pts',(13.034500095191,-1.57531157960346,5.22014856042382));
#86050=CARTESIAN_POINT('Ctrl Pts',(12.9844062983381,-1.50837272576141,5.21483056847728));
#86051=CARTESIAN_POINT('Ctrl Pts',(12.9347409969261,-1.44200645765842,5.20955806590161));
#86052=CARTESIAN_POINT('Ctrl Pts',(12.8882642141893,-1.37306074742762,5.20428556332595));
#86053=CARTESIAN_POINT('Ctrl Pts',(12.8452534888802,-1.30187315926588,5.19901306075028));
#86054=CARTESIAN_POINT('Ctrl Pts',(12.8023036373243,-1.23078632401286,5.19374802043011));
#86055=CARTESIAN_POINT('Ctrl Pts',(12.7628103357478,-1.15746429922706,5.18848298010994));
#86056=CARTESIAN_POINT('Ctrl Pts',(12.7270097454968,-1.08227609829163,5.18321793978977));
#86057=CARTESIAN_POINT('Ctrl Pts',(12.6912492744183,-1.00717215541974,5.17795879962542));
#86058=CARTESIAN_POINT('Ctrl Pts',(12.659173489575,-0.930206601019301,5.17269965946107));
#86059=CARTESIAN_POINT('Ctrl Pts',(12.6309735430406,-0.851774557160795,
5.16744051929673));
#86060=CARTESIAN_POINT('Ctrl Pts',(12.6027972054207,-0.77340817638473,5.16218578206946));
#86061=CARTESIAN_POINT('Ctrl Pts',(12.5784904108169,-0.69357817516063,5.1569310448422));
#86062=CARTESIAN_POINT('Ctrl Pts',(12.5581963739879,-0.612700009788105,
5.15167630761493));
#86063=CARTESIAN_POINT('Ctrl Pts',(12.5379122956235,-0.531861532051385,
5.14642414893401));
#86064=CARTESIAN_POINT('Ctrl Pts',(12.5216371714886,-0.449976355376292,
5.14117199025308));
#86065=CARTESIAN_POINT('Ctrl Pts',(12.5094641290169,-0.367474251270026,
5.13591983157216));
#86066=CARTESIAN_POINT('Ctrl Pts',(12.4972912357025,-0.284973158068802,
5.13066773724636));
#86067=CARTESIAN_POINT('Ctrl Pts',(12.4892203979113,-0.201855603551131,
5.12541564292057));
#86068=CARTESIAN_POINT('Ctrl Pts',(12.4852932836739,-0.118559608908535,
5.12016354859477));
#86069=CARTESIAN_POINT('Ctrl Pts',(12.4834039743466,-0.0784864431958992,
5.11763679989384));
#86070=CARTESIAN_POINT('Ctrl Pts',(12.4824729639348,-0.038372057539079,
5.11511005119291));
#86071=CARTESIAN_POINT('Ctrl Pts',(12.4825005975619,0.00173456729401744,
5.11258330249198));
#86072=CARTESIAN_POINT('Ctrl Pts',(12.4825005975625,0.00173456822324807,
5.11258330243344));
#86073=CARTESIAN_POINT('Ctrl Pts',(12.4825660917933,0.0967908966663681,
5.10659467947122));
#86074=CARTESIAN_POINT('Ctrl Pts',(12.4880193463078,0.191635955587718,5.10060605650901));
#86075=CARTESIAN_POINT('Ctrl Pts',(12.4987647943891,0.285707361144845,5.09461743354679));
#86076=CARTESIAN_POINT('Ctrl Pts',(12.5100725482397,0.384701492462413,5.08831542791158));
#86077=CARTESIAN_POINT('Ctrl Pts',(12.5272411438782,0.482838514846412,5.08201342227637));
#86078=CARTESIAN_POINT('Ctrl Pts',(12.5501013634223,0.579485047688556,5.07571141664117));
#86079=CARTESIAN_POINT('Ctrl Pts',(12.5729615829664,0.676131580530701,5.06940941100596));
#86080=CARTESIAN_POINT('Ctrl Pts',(12.6015132358442,0.771287443638239,5.06310740537075));
#86081=CARTESIAN_POINT('Ctrl Pts',(12.6355307871045,0.864344602151889,5.05680539973555));
#86082=CARTESIAN_POINT('Ctrl Pts',(12.6365393029679,0.867103460949512,5.05661856463369));
#86083=CARTESIAN_POINT('Ctrl Pts',(12.6375527128651,0.86986073376603,5.05643172953183));
#86084=CARTESIAN_POINT('Ctrl Pts',(12.6385710119932,0.872616401748855,5.05624489442998));
#86085=CARTESIAN_POINT('Origin',(15.,0.,3.));
#86086=CARTESIAN_POINT('',(12.4825000279491,0.000375131315902114,4.11258330252632));
#86087=CARTESIAN_POINT('Ctrl Pts',(12.6385710119932,0.872616401748855,5.05624489442998));
#86088=CARTESIAN_POINT('Ctrl Pts',(12.6672209705858,0.950147425220547,5.05098826817542));
#86089=CARTESIAN_POINT('Ctrl Pts',(12.6997453794103,1.02640706388388,5.04573164192086));
#86090=CARTESIAN_POINT('Ctrl Pts',(12.7360110065744,1.10098142021001,5.0404750156663));
#86091=CARTESIAN_POINT('Ctrl Pts',(12.7722258857873,1.17545142163892,5.03522574522036));
#86092=CARTESIAN_POINT('Ctrl Pts',(12.8121713842627,1.24824041385453,5.02997647477441));
#86093=CARTESIAN_POINT('Ctrl Pts',(12.8556654677086,1.31895248724981,5.02472720432846));
#86094=CARTESIAN_POINT('Ctrl Pts',(12.8991472891697,1.38964462528165,5.01947941377285));
#86095=CARTESIAN_POINT('Ctrl Pts',(12.9461755055359,1.45826059395244,5.01423162321724));
#86096=CARTESIAN_POINT('Ctrl Pts',(12.9965212968207,1.52442754367236,5.00898383266163));
#86097=CARTESIAN_POINT('Ctrl Pts',(13.0467934877305,1.59049776410885,5.00374371383673));
#86098=CARTESIAN_POINT('Ctrl Pts',(13.1003733045611,1.65412573716825,4.99850359501183));
#86099=CARTESIAN_POINT('Ctrl Pts',(13.1569894777469,1.71496893991238,4.99326347618692));
#86100=CARTESIAN_POINT('Ctrl Pts',(13.2135877355353,1.77579288967475,4.98802501552444));
#86101=CARTESIAN_POINT('Ctrl Pts',(13.27322012749,1.83383348204527,4.98278655486195));
#86102=CARTESIAN_POINT('Ctrl Pts',(13.3355763533395,1.88878272292961,4.97754809419947));
#86103=CARTESIAN_POINT('Ctrl Pts',(13.3979316213402,1.94373111974321,4.97230971400454));
#86104=CARTESIAN_POINT('Ctrl Pts',(13.463010293335,1.99558795555208,4.96707133380962));
#86105=CARTESIAN_POINT('Ctrl Pts',(13.5304676465996,2.04408437015443,4.9618329536147));
#86106=CARTESIAN_POINT('Ctrl Pts',(13.59813121221,2.09272903485747,4.95657856006296));
#86107=CARTESIAN_POINT('Ctrl Pts',(13.6681876489952,2.137992425348,4.95132416651121));
#86108=CARTESIAN_POINT('Ctrl Pts',(13.7402598195989,2.17964697322364,4.94606977295947));
#86109=CARTESIAN_POINT('Ctrl Pts',(13.8122158132601,2.22123437593118,4.94082384924251));
#86110=CARTESIAN_POINT('Ctrl Pts',(13.8861806201403,2.25922437893871,4.93557792552555));
#86111=CARTESIAN_POINT('Ctrl Pts',(13.9617558816988,2.29343746389843,4.93033200180859));
#86112=CARTESIAN_POINT('Ctrl Pts',(14.037514173934,2.32773340724282,4.92507337333946));
#86113=CARTESIAN_POINT('Ctrl Pts',(14.114890291854,2.35823396355735,4.91981474487033));
#86114=CARTESIAN_POINT('Ctrl Pts',(14.1934662938004,2.38480809097165,4.91455611640119));
#86115=CARTESIAN_POINT('Ctrl Pts',(14.2720422957467,2.41138221838595,4.90929748793206));
#86116=CARTESIAN_POINT('Ctrl Pts',(14.3518177225178,2.43402984975802,4.90403885946293));
#86117=CARTESIAN_POINT('Ctrl Pts',(14.4323647341015,2.45267128961635,4.8987802309938));
#86118=CARTESIAN_POINT('Ctrl Pts',(14.5128834668174,2.47130618474009,4.89352344875157));
#86119=CARTESIAN_POINT('Ctrl Pts',(14.5944684357902,2.48600602173817,4.88826666650934));
#86120=CARTESIAN_POINT('Ctrl Pts',(14.6767007227819,2.49665452703218,4.88300988426711));
#86121=CARTESIAN_POINT('Ctrl Pts',(14.7588169739909,2.50728800650491,4.87776051972983));
#86122=CARTESIAN_POINT('Ctrl Pts',(14.8415782753605,2.51388145090071,4.87251115519255));
#86123=CARTESIAN_POINT('Ctrl Pts',(14.9245538919164,2.51636923657381,4.86726179065528));
#86124=CARTESIAN_POINT('Ctrl Pts',(15.0078732927155,2.51886732963057,4.86199067697181));
#86125=CARTESIAN_POINT('Ctrl Pts',(15.0914083300651,2.51722555892271,4.85671956328834));
#86126=CARTESIAN_POINT('Ctrl Pts',(15.1747159447591,2.51142998880059,4.85144844960487));
#86127=CARTESIAN_POINT('Ctrl Pts',(15.2575327894807,2.50566856071698,4.84620838835673));
#86128=CARTESIAN_POINT('Ctrl Pts',(15.3401244188441,2.49580217124105,4.84096832710858));
#86129=CARTESIAN_POINT('Ctrl Pts',(15.4220556324454,2.48186931427122,4.83572826586043));
#86130=CARTESIAN_POINT('Ctrl Pts',(15.5039601720778,2.46794099335766,4.83048991059496));
#86131=CARTESIAN_POINT('Ctrl Pts',(15.5852042687661,2.44994891162134,4.82525155532949));
#86132=CARTESIAN_POINT('Ctrl Pts',(15.6653601224456,2.42798314604101,4.82001320006402));
#86133=CARTESIAN_POINT('Ctrl Pts',(15.7455140166557,2.40601791743013,4.81477497285404));
#86134=CARTESIAN_POINT('Ctrl Pts',(15.8245792763412,2.38007932102533,4.80953674564406));
#86135=CARTESIAN_POINT('Ctrl Pts',(15.9021418820164,2.35030769787955,4.80429851843407));
#86136=CARTESIAN_POINT('Ctrl Pts',(15.9805493889443,2.3202117679177,4.79900323041891));
#86137=CARTESIAN_POINT('Ctrl Pts',(16.0574208498021,2.2861989507252,4.79370794240374));
#86138=CARTESIAN_POINT('Ctrl Pts',(16.1323496339631,2.24846404384497,4.78841265438857));
#86139=CARTESIAN_POINT('Ctrl Pts',(16.2065770889589,2.21108233355049,4.78316692996856));
#86140=CARTESIAN_POINT('Ctrl Pts',(16.2788977069171,2.17004820348001,4.77792120554854));
#86141=CARTESIAN_POINT('Ctrl Pts',(16.3489428619747,2.12559624696874,4.77267548112852));
#86142=CARTESIAN_POINT('Ctrl Pts',(16.4199807368444,2.08051429202457,4.76735541131578));
#86143=CARTESIAN_POINT('Ctrl Pts',(16.4886777444177,2.03191715767091,4.76203534150304));
#86144=CARTESIAN_POINT('Ctrl Pts',(16.5546831971137,1.9800925247605,4.7567152716903));
#86145=CARTESIAN_POINT('Ctrl Pts',(16.6206886498097,1.92826789185008,4.75139520187756));
#86146=CARTESIAN_POINT('Ctrl Pts',(16.6840022215195,1.87321612871151,4.74607513206482));
#86147=CARTESIAN_POINT('Ctrl Pts',(16.7443125632853,1.81526304748511,4.74075506225207));
#86148=CARTESIAN_POINT('Ctrl Pts',(16.8039030619099,1.75800167396285,4.73549849093153));
#86149=CARTESIAN_POINT('Ctrl Pts',(16.8607803053939,1.69769780895363,4.73024191961099));
#86150=CARTESIAN_POINT('Ctrl Pts',(16.9146180609925,1.63463877677032,4.72498534829044));
#86151=CARTESIAN_POINT('Ctrl Pts',(16.968379801339,1.571668779655,4.71973619889137));
#86152=CARTESIAN_POINT('Ctrl Pts',(17.0191102812959,1.50595169023062,4.71448704949229));
#86153=CARTESIAN_POINT('Ctrl Pts',(17.0665192341682,1.4378124025104,4.70923790009322));
#86154=CARTESIAN_POINT('Ctrl Pts',(17.1141270437554,1.36938730474612,4.70396673315227));
#86155=CARTESIAN_POINT('Ctrl Pts',(17.1583850577259,1.29851996784166,4.69869556621131));
#86156=CARTESIAN_POINT('Ctrl Pts',(17.1990395300914,1.22557390437916,4.69342439927036));
#86157=CARTESIAN_POINT('Ctrl Pts',(17.2394523698836,1.15306140071972,4.68818456186238));
#86158=CARTESIAN_POINT('Ctrl Pts',(17.2763041580762,1.0784952191346,4.68294472445441));
#86159=CARTESIAN_POINT('Ctrl Pts',(17.309389396096,1.00226087781539,4.67770488704643));
#86160=CARTESIAN_POINT('Ctrl Pts',(17.3424638447102,0.926051397227946,4.67246675839844));
#86161=CARTESIAN_POINT('Ctrl Pts',(17.3717739992685,0.848175260046755,4.66722862975046));
#86162=CARTESIAN_POINT('Ctrl Pts',(17.3971616089557,0.769039966808437,4.66199050110247));
#86163=CARTESIAN_POINT('Ctrl Pts',(17.4225485860033,0.689906645560786,4.65675250298462));
#86164=CARTESIAN_POINT('Ctrl Pts',(17.4440130726898,0.609514670065358,4.65151450486677));
#86165=CARTESIAN_POINT('Ctrl Pts',(17.4614464470319,0.528287458108025,4.64627650674893));
#86166=CARTESIAN_POINT('Ctrl Pts',(17.4790713721756,0.446167754699549,4.64098095564571));
#86167=CARTESIAN_POINT('Ctrl Pts',(17.4925759379711,0.363194814282982,4.6356854045425));
#86168=CARTESIAN_POINT('Ctrl Pts',(17.5019011574019,0.279815740427992,4.63038985343928));
#86169=CARTESIAN_POINT('Ctrl Pts',(17.5111382242823,0.197224860143897,4.62514436189107));
#86170=CARTESIAN_POINT('Ctrl Pts',(17.5162746601712,0.114235961838988,4.61989887034286));
#86171=CARTESIAN_POINT('Ctrl Pts',(17.5173055914026,0.0312859312310394,
4.61465337879465));
#86172=CARTESIAN_POINT('Ctrl Pts',(17.5183512804384,-0.0528515309784231,
4.60933279791393));
#86173=CARTESIAN_POINT('Ctrl Pts',(17.5151730139759,-0.136948512252474,
4.60401221703321));
#86174=CARTESIAN_POINT('Ctrl Pts',(17.507820208695,-0.220553963602515,4.59869163615249));
#86175=CARTESIAN_POINT('Ctrl Pts',(17.5004674034141,-0.304159414952556,
4.59337105527178));
#86176=CARTESIAN_POINT('Ctrl Pts',(17.4889401897988,-0.387272861644603,
4.58805047439106));
#86177=CARTESIAN_POINT('Ctrl Pts',(17.4733414428944,-0.469455383248395,
4.58272989351034));
#86178=CARTESIAN_POINT('Ctrl Pts',(17.4579299050636,-0.55065158756479,4.57747316782412));
#86179=CARTESIAN_POINT('Ctrl Pts',(17.4384875391269,-0.631236991974626,
4.57221644213791));
#86180=CARTESIAN_POINT('Ctrl Pts',(17.4150768313274,-0.710781364967923,
4.56695971645169));
#86181=CARTESIAN_POINT('Ctrl Pts',(17.3916991670801,-0.790213463327384,
4.56171041048518));
#86182=CARTESIAN_POINT('Ctrl Pts',(17.364364415959,-0.868607010265535,4.55646110451866));
#86183=CARTESIAN_POINT('Ctrl Pts',(17.333186179455,-0.945541380374444,4.55121179855215));
#86184=CARTESIAN_POINT('Ctrl Pts',(17.3018783306093,-1.0227955775479,4.54594067047784));
#86185=CARTESIAN_POINT('Ctrl Pts',(17.2666950549121,-1.09857797552401,4.54066954240352));
#86186=CARTESIAN_POINT('Ctrl Pts',(17.2278022311034,-1.17247749193354,4.53539841432921));
#86187=CARTESIAN_POINT('Ctrl Pts',(17.1891390980827,-1.24594057723586,4.53015841615091));
#86188=CARTESIAN_POINT('Ctrl Pts',(17.146810328221,-1.3175425467998,4.52491841797262));
#86189=CARTESIAN_POINT('Ctrl Pts',(17.1010266047129,-1.38690066561695,4.51967841979432));
#86190=CARTESIAN_POINT('Ctrl Pts',(17.0552578005805,-1.45623618295573,4.51444012915521));
#86191=CARTESIAN_POINT('Ctrl Pts',(17.0060365327093,-1.52332891726462,4.50920183851609));
#86192=CARTESIAN_POINT('Ctrl Pts',(16.9536177056951,-1.58782370242873,4.50396354787698));
#86193=CARTESIAN_POINT('Ctrl Pts',(16.9012001748603,-1.65231689280697,4.49872538676698));
#86194=CARTESIAN_POINT('Ctrl Pts',(16.8455855337545,-1.7142119046275,4.49348722565697));
#86195=CARTESIAN_POINT('Ctrl Pts',(16.7870691289199,-1.77318644774361,4.48824906454696));
#86196=CARTESIAN_POINT('Ctrl Pts',(16.7279137269679,-1.83280499083126,4.48295370289877));
#86197=CARTESIAN_POINT('Ctrl Pts',(16.6657931261,-1.8894385389231,4.47765834125057));
#86198=CARTESIAN_POINT('Ctrl Pts',(16.6010495560704,-1.94279349623342,4.47236297960237));
#86199=CARTESIAN_POINT('Ctrl Pts',(16.5369137185718,-1.99564762321825,4.46711732425761));
#86200=CARTESIAN_POINT('Ctrl Pts',(16.4702043590405,-2.04528422344915,4.46187166891285));
#86201=CARTESIAN_POINT('Ctrl Pts',(16.4012847755172,-2.09146054897142,4.45662601356809));
#86202=CARTESIAN_POINT('Ctrl Pts',(16.3313855991194,-2.13829320462705,4.45130579876818));
#86203=CARTESIAN_POINT('Ctrl Pts',(16.2592132971079,-2.18156619514584,4.44598558396826));
#86204=CARTESIAN_POINT('Ctrl Pts',(16.1851725660572,-2.22107456846127,4.44066536916835));
#86205=CARTESIAN_POINT('Ctrl Pts',(16.1111318350065,-2.26058294177669,4.43534515436843));
#86206=CARTESIAN_POINT('Ctrl Pts',(16.035223143569,-2.29632654792773,4.43002493956852));
#86207=CARTESIAN_POINT('Ctrl Pts',(15.9578702252833,-2.32815181668116,4.4247047247686));
#86208=CARTESIAN_POINT('Ctrl Pts',(15.8814408538521,-2.35959711105865,4.41944803010151));
#86209=CARTESIAN_POINT('Ctrl Pts',(15.803321217137,-2.38733251975011,4.41419133543442));
#86210=CARTESIAN_POINT('Ctrl Pts',(15.7239058116032,-2.4111753619194,4.40893464076733));
#86211=CARTESIAN_POINT('Ctrl Pts',(15.6446025012189,-2.43498454982552,4.40368536594493));
#86212=CARTESIAN_POINT('Ctrl Pts',(15.5640074929885,-2.45491195338061,4.39843609112252));
#86213=CARTESIAN_POINT('Ctrl Pts',(15.4825351598875,-2.47082295389054,4.39318681630012));
#86214=CARTESIAN_POINT('Ctrl Pts',(15.4007235287782,-2.48680021702702,4.3879156804554));
#86215=CARTESIAN_POINT('Ctrl Pts',(15.318027683937,-2.49872736769975,4.38264454461068));
#86216=CARTESIAN_POINT('Ctrl Pts',(15.2348825720286,-2.50651878655582,4.37737340876596));
#86217=CARTESIAN_POINT('Ctrl Pts',(15.1522291074359,-2.51426413378989,4.37213344179851));
#86218=CARTESIAN_POINT('Ctrl Pts',(15.0691321382078,-2.5179224807289,4.36689347483107));
#86219=CARTESIAN_POINT('Ctrl Pts',(14.9860273324777,-2.51746122404344,4.36165350786362));
#86220=CARTESIAN_POINT('Ctrl Pts',(14.9029496072365,-2.51700011766285,4.35641524838908));
#86221=CARTESIAN_POINT('Ctrl Pts',(14.8198645113117,-2.51242207640567,4.35117698891454));
#86222=CARTESIAN_POINT('Ctrl Pts',(14.7372087773475,-2.50374659726116,4.34593872944));
#86223=CARTESIAN_POINT('Ctrl Pts',(14.654555085836,-2.49507133249082,4.34070059940472));
#86224=CARTESIAN_POINT('Ctrl Pts',(14.5723311936678,-2.48229888035421,4.33546246936944));
#86225=CARTESIAN_POINT('Ctrl Pts',(14.4909683880573,-2.46550057149518,4.33022433933416));
#86226=CARTESIAN_POINT('Ctrl Pts',(14.4087160413711,-2.44851860641116,4.32492894072522));
#86227=CARTESIAN_POINT('Ctrl Pts',(14.3273441995726,-2.42742229671369,4.31963354211628));
#86228=CARTESIAN_POINT('Ctrl Pts',(14.2472857420408,-2.40233792291278,4.31433814350734));
#86229=CARTESIAN_POINT('Ctrl Pts',(14.1679797893908,-2.37748932824535,4.30909251869404));
#86230=CARTESIAN_POINT('Ctrl Pts',(14.0899630506313,-2.34872754544044,4.30384689388075));
#86231=CARTESIAN_POINT('Ctrl Pts',(14.0136373062393,-2.31622427376046,4.29860126906745));
#86232=CARTESIAN_POINT('Ctrl Pts',(13.9362252216669,-2.28325838477748,4.29328098356069));
#86233=CARTESIAN_POINT('Ctrl Pts',(13.8605530875749,-2.24644388040261,4.28796069805392));
#86234=CARTESIAN_POINT('Ctrl Pts',(13.7870136622207,-2.20600779562559,4.28264041254716));
#86235=CARTESIAN_POINT('Ctrl Pts',(13.7134742368666,-2.16557171084856,4.2773201270404));
#86236=CARTESIAN_POINT('Ctrl Pts',(13.6420679019044,-2.12151435634008,4.27199984153363));
#86237=CARTESIAN_POINT('Ctrl Pts',(13.573154773638,-2.07410678365602,4.26667955602687));
#86238=CARTESIAN_POINT('Ctrl Pts',(13.505345422078,-2.02745853471412,4.26144448515717));
#86239=CARTESIAN_POINT('Ctrl Pts',(13.4396966081709,-1.97739226415211,4.25620941428747));
#86240=CARTESIAN_POINT('Ctrl Pts',(13.3765751239122,-1.9241356297567,4.25097434341777));
#86241=CARTESIAN_POINT('Ctrl Pts',(13.3135429179877,-1.87095432096019,4.24574667697483));
#86242=CARTESIAN_POINT('Ctrl Pts',(13.2530312955316,-1.81459190711496,4.24051901053188));
#86243=CARTESIAN_POINT('Ctrl Pts',(13.1953778145324,-1.75531906436353,4.23529134408894));
#86244=CARTESIAN_POINT('Ctrl Pts',(13.1377897754579,-1.69611350165912,4.23006961152107));
#86245=CARTESIAN_POINT('Ctrl Pts',(13.0830537535038,-1.63400440705708,4.2248478789532));
#86246=CARTESIAN_POINT('Ctrl Pts',(13.0314728318686,-1.56930144915777,4.21962614638532));
#86247=CARTESIAN_POINT('Ctrl Pts',(12.9799237606473,-1.50463844432485,4.21440763815579));
#86248=CARTESIAN_POINT('Ctrl Pts',(12.9315262120739,-1.43738511830809,4.20918912992626));
#86249=CARTESIAN_POINT('Ctrl Pts',(12.8865443118865,-1.36788570589086,4.20397062169673));
#86250=CARTESIAN_POINT('Ctrl Pts',(12.8415763400671,-1.29840781353819,4.1987537293461));
#86251=CARTESIAN_POINT('Ctrl Pts',(12.8000221690277,-1.22668560636456,4.19353683699547));
#86252=CARTESIAN_POINT('Ctrl Pts',(12.7621029009024,-1.15309272127195,4.18831994464484));
#86253=CARTESIAN_POINT('Ctrl Pts',(12.7241837012758,-1.07949996912034,4.18310306171821));
#86254=CARTESIAN_POINT('Ctrl Pts',(12.6898996032389,-1.00403696023441,4.17788617879157));
#86255=CARTESIAN_POINT('Ctrl Pts',(12.6594253212799,-0.927101085823097,
4.17266929586493));
#86256=CARTESIAN_POINT('Ctrl Pts',(12.628921471219,-0.850090563294519,4.16744735118406));
#86257=CARTESIAN_POINT('Ctrl Pts',(12.602234991766,-0.771604754724609,4.16222540650318));
#86258=CARTESIAN_POINT('Ctrl Pts',(12.5794918391932,-0.692059602539742,
4.15700346182231));
#86259=CARTESIAN_POINT('Ctrl Pts',(12.5567376281915,-0.612475773025612,
4.15177897806937));
#86260=CARTESIAN_POINT('Ctrl Pts',(12.53793066827,-0.531832027762312,4.14655449431642));
#86261=CARTESIAN_POINT('Ctrl Pts',(12.5231459615928,-0.45055557085201,4.14133001056348));
#86262=CARTESIAN_POINT('Ctrl Pts',(12.5083357132044,-0.369138702648425,
4.13609650111542));
#86263=CARTESIAN_POINT('Ctrl Pts',(12.4975616595679,-0.287087401455886,
4.13086299166736));
#86264=CARTESIAN_POINT('Ctrl Pts',(12.4908469665597,-0.204834823155961,
4.1256294822193));
#86265=CARTESIAN_POINT('Ctrl Pts',(12.4852674669627,-0.136487956529057,
4.12128075565497));
#86266=CARTESIAN_POINT('Ctrl Pts',(12.4824898390633,-0.0680023103452117,
4.11693202909065));
#86267=CARTESIAN_POINT('Ctrl Pts',(12.4825000279491,0.000375131315901805,
4.11258330252632));
#86268=CARTESIAN_POINT('Ctrl Pts',(12.4825000279491,0.000375131855856907,
4.11258330249198));
#86269=CARTESIAN_POINT('Ctrl Pts',(12.482503096382,0.0209673034085757,4.1112736640897));
#86270=CARTESIAN_POINT('Ctrl Pts',(12.4827588140224,0.041557321852414,4.10996402568741));
#86271=CARTESIAN_POINT('Ctrl Pts',(12.4832670510668,0.062141079441871,4.10865438728512));
#86272=CARTESIAN_POINT('Ctrl Pts',(12.4853066576079,0.144745775577443,4.10339867623244));
#86273=CARTESIAN_POINT('Ctrl Pts',(12.4914212102481,0.227401430820226,4.09814296517976));
#86274=CARTESIAN_POINT('Ctrl Pts',(12.501618824813,0.309673624112754,4.09288725412709));
#86275=CARTESIAN_POINT('Ctrl Pts',(12.5118038118859,0.391843941476571,4.08763805111102));
#86276=CARTESIAN_POINT('Ctrl Pts',(12.5260617710905,0.473631285663338,4.08238884809495));
#86277=CARTESIAN_POINT('Ctrl Pts',(12.5443488333121,0.554602197565569,4.07713964507888));
#86278=CARTESIAN_POINT('Ctrl Pts',(12.5626153556443,0.635482163553971,4.07189633792781));
#86279=CARTESIAN_POINT('Ctrl Pts',(12.5849018858058,0.715547072294699,4.06665303077675));
#86280=CARTESIAN_POINT('Ctrl Pts',(12.6111130818692,0.794371161601245,4.06140972362568));
#86281=CARTESIAN_POINT('Ctrl Pts',(12.6198333339686,0.820595296073974,4.05966531791138));
#86282=CARTESIAN_POINT('Ctrl Pts',(12.628987563394,0.846682173052394,4.05792091219707));
#86283=CARTESIAN_POINT('Ctrl Pts',(12.6385710119932,0.872616401748848,4.05617650648277));
#86284=CARTESIAN_POINT('',(12.4825009521567,-0.00218954522945693,4.38741669750802));
#86285=CARTESIAN_POINT('Ctrl Pts',(12.6421214752944,0.871321765791516,4.3311309048973));
#86286=CARTESIAN_POINT('Ctrl Pts',(12.5397813919921,0.591632227618603,4.34989269415061));
#86287=CARTESIAN_POINT('Ctrl Pts',(12.4844694673097,0.294291735004427,4.36865448340391));
#86288=CARTESIAN_POINT('Ctrl Pts',(12.4817777656426,-0.00218346073577532,
4.38741627265722));
#86289=CARTESIAN_POINT('Ctrl Pts',(12.4825009521567,-0.00218954522945693,
4.38741669750802));
#86290=CARTESIAN_POINT('Ctrl Pts',(12.4826026785113,-0.119152646681798,
4.39482064432068));
#86291=CARTESIAN_POINT('Ctrl Pts',(12.4908590803219,-0.235770821827561,
4.40222459113333));
#86292=CARTESIAN_POINT('Ctrl Pts',(12.5071061350226,-0.351121671159536,
4.40962853794598));
#86293=CARTESIAN_POINT('Ctrl Pts',(12.5145083371291,-0.403675830399398,
4.4130017961582));
#86294=CARTESIAN_POINT('Ctrl Pts',(12.5235685720467,-0.455967358934549,
4.41637505437042));
#86295=CARTESIAN_POINT('Ctrl Pts',(12.5342682792954,-0.507910751521386,
4.41974831258264));
#86296=CARTESIAN_POINT('Ctrl Pts',(12.5509424201429,-0.588857961006813,
4.42500510898262));
#86297=CARTESIAN_POINT('Ctrl Pts',(12.5716374708985,-0.669131665759261,
4.43026190538259));
#86298=CARTESIAN_POINT('Ctrl Pts',(12.5962842531434,-0.748302651547934,
4.43551870178256));
#86299=CARTESIAN_POINT('Ctrl Pts',(12.6208962422798,-0.827361874077981,
4.44076807732388));
#86300=CARTESIAN_POINT('Ctrl Pts',(12.6494487461163,-0.905321033100365,
4.44601745286519));
#86301=CARTESIAN_POINT('Ctrl Pts',(12.6818216267449,-0.981761315072212,
4.4512668284065));
#86302=CARTESIAN_POINT('Ctrl Pts',(12.7143285470236,-1.05851809741272,4.45653793894475));
#86303=CARTESIAN_POINT('Ctrl Pts',(12.7506874579344,-1.13374293511867,4.46180904948299));
#86304=CARTESIAN_POINT('Ctrl Pts',(12.7907261080111,-1.20702738998586,4.46708016002124));
#86305=CARTESIAN_POINT('Ctrl Pts',(12.8305289366073,-1.27988021070443,4.4723202245305));
#86306=CARTESIAN_POINT('Ctrl Pts',(12.8739680542269,-1.3508150337928,4.47756028903977));
#86307=CARTESIAN_POINT('Ctrl Pts',(12.9208268435731,-1.41945244217396,4.48280035354904));
#86308=CARTESIAN_POINT('Ctrl Pts',(12.9676703512691,-1.48806746643316,4.48803870916157));
#86309=CARTESIAN_POINT('Ctrl Pts',(13.017931055935,-1.55438618354357,4.4932770647741));
#86310=CARTESIAN_POINT('Ctrl Pts',(13.071348553121,-1.61805742989904,4.49851542038663));
#86311=CARTESIAN_POINT('Ctrl Pts',(13.1247647147894,-1.68172708437781,4.50375364503241));
#86312=CARTESIAN_POINT('Ctrl Pts',(13.1813372148716,-1.74274904716061,4.50899186967819));
#86313=CARTESIAN_POINT('Ctrl Pts',(13.2407657232065,-1.80080565563164,4.51423009432397));
#86314=CARTESIAN_POINT('Ctrl Pts',(13.3008415593174,-1.85949464839591,4.51952537657401));
#86315=CARTESIAN_POINT('Ctrl Pts',(13.3638356695576,-1.91515294399448,4.52482065882404));
#86316=CARTESIAN_POINT('Ctrl Pts',(13.4294013205346,-1.967492322237,4.53011594107407));
#86317=CARTESIAN_POINT('Ctrl Pts',(13.4943532315647,-2.01934176761457,4.53536165581126));
#86318=CARTESIAN_POINT('Ctrl Pts',(13.5618283271267,-2.067933948377,4.54060737054844));
#86319=CARTESIAN_POINT('Ctrl Pts',(13.6314595714653,-2.11303178997998,4.54585308528563));
#86320=CARTESIAN_POINT('Ctrl Pts',(13.7020777492643,-2.15876883556806,4.55117315129209));
#86321=CARTESIAN_POINT('Ctrl Pts',(13.7749132499518,-2.20091146499363,4.55649321729855));
#86322=CARTESIAN_POINT('Ctrl Pts',(13.8495582792929,-2.2392610605413,4.561813283305));
#86323=CARTESIAN_POINT('Ctrl Pts',(13.924203308634,-2.27761065608897,4.56713334931146));
#86324=CARTESIAN_POINT('Ctrl Pts',(14.0006573958101,-2.31216707511688,4.57245341531792));
#86325=CARTESIAN_POINT('Ctrl Pts',(14.0784945123771,-2.34278336307069,4.57777348132438));
#86326=CARTESIAN_POINT('Ctrl Pts',(14.1554076810325,-2.37303622729349,4.58303039668892));
#86327=CARTESIAN_POINT('Ctrl Pts',(14.2339531941902,-2.39955296223892,4.58828731205347));
#86328=CARTESIAN_POINT('Ctrl Pts',(14.3137337174689,-2.42215706333446,4.59354422741801));
#86329=CARTESIAN_POINT('Ctrl Pts',(14.393401662519,-2.44472926780212,4.59879372475374));
#86330=CARTESIAN_POINT('Ctrl Pts',(14.4743007160961,-2.4633996805871,4.60404322208948));
#86331=CARTESIAN_POINT('Ctrl Pts',(14.5560144214902,-2.4780401643386,4.60929271942521));
#86332=CARTESIAN_POINT('Ctrl Pts',(14.6380640896605,-2.49274084187942,4.61456379986858));
#86333=CARTESIAN_POINT('Ctrl Pts',(14.7209346856385,-2.50337820526777,4.61983488031195));
#86334=CARTESIAN_POINT('Ctrl Pts',(14.8041900168466,-2.50987344312367,4.62510596075533));
#86335=CARTESIAN_POINT('Ctrl Pts',(14.8869574766042,-2.51633061925946,4.63034615297058));
#86336=CARTESIAN_POINT('Ctrl Pts',(14.9701047104277,-2.51869404562131,4.63558634518584));
#86337=CARTESIAN_POINT('Ctrl Pts',(15.0531955631248,-2.51693791780088,4.6408265374011));
#86338=CARTESIAN_POINT('Ctrl Pts',(15.1362593492159,-2.51518236203403,4.64606502263883));
#86339=CARTESIAN_POINT('Ctrl Pts',(15.2192663300518,-2.50930992706722,4.65130350787656));
#86340=CARTESIAN_POINT('Ctrl Pts',(15.3017800988686,-2.49934691908243,4.65654199311428));
#86341=CARTESIAN_POINT('Ctrl Pts',(15.3842918320055,-2.48938415689293,4.66178034911444));
#86342=CARTESIAN_POINT('Ctrl Pts',(15.4663099197064,-2.47533107868237,4.66701870511459));
#86343=CARTESIAN_POINT('Ctrl Pts',(15.5474042080151,-2.4572657330959,4.67225706111475));
#86344=CARTESIAN_POINT('Ctrl Pts',(15.629377444368,-2.43900458456816,4.67755219352736));
#86345=CARTESIAN_POINT('Ctrl Pts',(15.7104062614077,-2.41664375387076,4.68284732593997));
#86346=CARTESIAN_POINT('Ctrl Pts',(15.7900598880583,-2.39031621826095,4.68814245835259));
#86347=CARTESIAN_POINT('Ctrl Pts',(15.8689721532152,-2.36423372135111,4.69338830729326));
#86348=CARTESIAN_POINT('Ctrl Pts',(15.9465343076132,-2.33425827725141,4.69863415623393));
#86349=CARTESIAN_POINT('Ctrl Pts',(16.0223472614685,-2.30056782707396,4.7038800051746));
#86350=CARTESIAN_POINT('Ctrl Pts',(16.0992285816531,-2.26640260654717,4.70919977932318));
#86351=CARTESIAN_POINT('Ctrl Pts',(16.1743105791559,-2.22841708208727,4.71451955347177));
#86352=CARTESIAN_POINT('Ctrl Pts',(16.2472042039599,-2.18684428426554,4.71983932762036));
#86353=CARTESIAN_POINT('Ctrl Pts',(16.3200978287638,-2.14527148644381,4.72515910176894));
#86354=CARTESIAN_POINT('Ctrl Pts',(16.390802704373,-2.10011173155922,4.73047887591753));
#86355=CARTESIAN_POINT('Ctrl Pts',(16.458963082923,-2.05164153122999,4.73579865006611));
#86356=CARTESIAN_POINT('Ctrl Pts',(16.5263035212876,-2.00375440666842,4.74105442960823));
#86357=CARTESIAN_POINT('Ctrl Pts',(16.5914075487985,-1.95246031526691,4.74631020915035));
#86358=CARTESIAN_POINT('Ctrl Pts',(16.6539103478986,-1.89799547183706,4.75156598869247));
#86359=CARTESIAN_POINT('Ctrl Pts',(16.7163248871285,-1.8436075379229,4.75681434657625));
#86360=CARTESIAN_POINT('Ctrl Pts',(16.7761451491439,-1.78605804606437,4.76206270446003));
#86361=CARTESIAN_POINT('Ctrl Pts',(16.8330363715109,-1.72562565775953,4.76731106234382));
#86362=CARTESIAN_POINT('Ctrl Pts',(16.8901769851375,-1.66492835495987,4.77258242719648));
#86363=CARTESIAN_POINT('Ctrl Pts',(16.9443624322927,-1.60132309141237,4.77785379204915));
#86364=CARTESIAN_POINT('Ctrl Pts',(16.9952882348807,-1.53513227760557,4.78312515690182));
#86365=CARTESIAN_POINT('Ctrl Pts',(17.0459018711517,-1.46934720198099,4.7883642092043));
#86366=CARTESIAN_POINT('Ctrl Pts',(17.0932954269318,-1.40100855361851,4.79360326150678));
#86367=CARTESIAN_POINT('Ctrl Pts',(17.1372090912285,-1.33046741800404,4.79884231380926));
#86368=CARTESIAN_POINT('Ctrl Pts',(17.181108467436,-1.25994923419866,4.80407966149319));
#86369=CARTESIAN_POINT('Ctrl Pts',(17.2215299573087,-1.18723037771864,4.80931700917712));
#86370=CARTESIAN_POINT('Ctrl Pts',(17.2582572587677,-1.1126906143322,4.81455435686105));
#86371=CARTESIAN_POINT('Ctrl Pts',(17.2949836812295,-1.03815263491123,4.81979157919916));
#86372=CARTESIAN_POINT('Ctrl Pts',(17.3280158881588,-0.961794249499344,
4.82502880153728));
#86373=CARTESIAN_POINT('Ctrl Pts',(17.3571843329208,-0.88401825243195,4.83026602387539));
#86374=CARTESIAN_POINT('Ctrl Pts',(17.3866828264446,-0.805362199134683,
4.83556250678643));
#86375=CARTESIAN_POINT('Ctrl Pts',(17.4122293803436,-0.725256695124534,
4.84085898969747));
#86376=CARTESIAN_POINT('Ctrl Pts',(17.4336999597987,-0.644135665582961,
4.8461554726085));
#86377=CARTESIAN_POINT('Ctrl Pts',(17.4549607719518,-0.563807187520034,
4.85140020894549));
#86378=CARTESIAN_POINT('Ctrl Pts',(17.4722248706125,-0.482483410093979,
4.85664494528247));
#86379=CARTESIAN_POINT('Ctrl Pts',(17.4854233756316,-0.400595673796245,
4.86188968161945));
#86380=CARTESIAN_POINT('Ctrl Pts',(17.4988172128962,-0.317496033923638,
4.86721203781751));
#86381=CARTESIAN_POINT('Ctrl Pts',(17.508024083252,-0.233816096765077,4.87253439401558));
#86382=CARTESIAN_POINT('Ctrl Pts',(17.513026721991,-0.150009814875842,4.87785675021365));
#86383=CARTESIAN_POINT('Ctrl Pts',(17.51802936073,-0.0662035329866071,4.88317910641171));
#86384=CARTESIAN_POINT('Ctrl Pts',(17.5188278275939,0.0177286035890774,
4.88850146260978));
#86385=CARTESIAN_POINT('Ctrl Pts',(17.5154596198684,0.101336818636153,4.89382381880785));
#86386=CARTESIAN_POINT('Ctrl Pts',(17.5121322980462,0.183930132684131,4.89908156814138));
#86387=CARTESIAN_POINT('Ctrl Pts',(17.5047267383458,0.266510655466996,4.90433931747492));
#86388=CARTESIAN_POINT('Ctrl Pts',(17.4932416552582,0.348643512036484,4.90959706680846));
#86389=CARTESIAN_POINT('Ctrl Pts',(17.4817727907503,0.430660385267855,4.91484739144811));
#86390=CARTESIAN_POINT('Ctrl Pts',(17.4662359093044,0.51223039527895,4.92009771608775));
#86391=CARTESIAN_POINT('Ctrl Pts',(17.4466816967508,0.592920673264535,4.9253480407274));
#86392=CARTESIAN_POINT('Ctrl Pts',(17.4270509550653,0.67392674800837,4.93061891351165));
#86393=CARTESIAN_POINT('Ctrl Pts',(17.4033713892679,0.754045720168594,4.93588978629591));
#86394=CARTESIAN_POINT('Ctrl Pts',(17.3757467156412,0.832846800510245,4.94116065908017));
#86395=CARTESIAN_POINT('Ctrl Pts',(17.3482786185898,0.911201236541949,4.94640165657176));
#86396=CARTESIAN_POINT('Ctrl Pts',(17.3169101696193,0.988252241036131,4.95164265406335));
#86397=CARTESIAN_POINT('Ctrl Pts',(17.2817936326646,1.06359017856083,4.95688365155495));
#86398=CARTESIAN_POINT('Ctrl Pts',(17.2466886001331,1.13890343485042,4.96212293205912));
#86399=CARTESIAN_POINT('Ctrl Pts',(17.2078381129796,1.21250432138666,4.96736221256328));
#86400=CARTESIAN_POINT('Ctrl Pts',(17.1654422248974,1.28400397999053,4.97260149306745));
#86401=CARTESIAN_POINT('Ctrl Pts',(17.1230474718603,1.3555017243676,4.97784063330282));
#86402=CARTESIAN_POINT('Ctrl Pts',(17.0771077426224,1.42489795675396,4.98307977353819));
#86403=CARTESIAN_POINT('Ctrl Pts',(17.0278679227338,1.49183039851959,4.98831891377356));
#86404=CARTESIAN_POINT('Ctrl Pts',(16.9781108816657,1.55946590696097,4.99361308658823));
#86405=CARTESIAN_POINT('Ctrl Pts',(16.9249842830702,1.62458516320357,4.9989072594029));
#86406=CARTESIAN_POINT('Ctrl Pts',(16.8687832353091,1.68684779082991,5.00420143221757));
#86407=CARTESIAN_POINT('Ctrl Pts',(16.8130872209956,1.7485509144836,5.0094480305749));
#86408=CARTESIAN_POINT('Ctrl Pts',(16.754372163587,1.80744825725024,5.01469462893223));
#86409=CARTESIAN_POINT('Ctrl Pts',(16.6929618352904,1.86324621943808,5.01994122728956));
#86410=CARTESIAN_POINT('Ctrl Pts',(16.6307162334952,1.91980311844294,5.0252591873329));
#86411=CARTESIAN_POINT('Ctrl Pts',(16.5657018681939,1.97317537879475,5.03057714737624));
#86412=CARTESIAN_POINT('Ctrl Pts',(16.4982883485331,2.02310115284677,5.03589510741957));
#86413=CARTESIAN_POINT('Ctrl Pts',(16.4308748288723,2.07302692689879,5.04121306746291));
#86414=CARTESIAN_POINT('Ctrl Pts',(16.3610625947837,2.11950599799578,5.04653102750625));
#86415=CARTESIAN_POINT('Ctrl Pts',(16.2892475889811,2.16232442161354,5.05184898754959));
#86416=CARTESIAN_POINT('Ctrl Pts',(16.2182439398869,2.20465908818283,5.05710686596364));
#86417=CARTESIAN_POINT('Ctrl Pts',(16.1450232189915,2.24357007403483,5.06236474437769));
#86418=CARTESIAN_POINT('Ctrl Pts',(16.0699490872646,2.27881881698867,5.06762262279174));
#86419=CARTESIAN_POINT('Ctrl Pts',(15.9949806778278,2.31401792130211,5.07287309685846));
#86420=CARTESIAN_POINT('Ctrl Pts',(15.9181644558188,2.34556483276518,5.07812357092518));
#86421=CARTESIAN_POINT('Ctrl Pts',(15.8398907776888,2.37326562600002,5.0833740449919));
#86422=CARTESIAN_POINT('Ctrl Pts',(15.7613135159864,2.40107385644709,5.08864488296271));
#86423=CARTESIAN_POINT('Ctrl Pts',(15.6812678730099,2.42500583125158,5.09391572093352));
#86424=CARTESIAN_POINT('Ctrl Pts',(15.6001713694366,2.44491320445299,5.09918655890433));
#86425=CARTESIAN_POINT('Ctrl Pts',(15.5195309540679,2.46470861822704,5.10442775358695));
#86426=CARTESIAN_POINT('Ctrl Pts',(15.4378519187879,2.48052446793078,5.10966894826957));
#86427=CARTESIAN_POINT('Ctrl Pts',(15.355560620274,2.492264611816,5.11491014295219));
#86428=CARTESIAN_POINT('Ctrl Pts',(15.2732960073148,2.50400094858847,5.12014963801177));
#86429=CARTESIAN_POINT('Ctrl Pts',(15.1904199813549,2.51166413955409,5.12538913307134));
#86430=CARTESIAN_POINT('Ctrl Pts',(15.1073675872123,2.51520942492195,5.13062862813092));
#86431=CARTESIAN_POINT('Ctrl Pts',(15.024317147798,2.51875462684768,5.1358679998733));
#86432=CARTESIAN_POINT('Ctrl Pts',(14.9410908089415,2.51818209731604,5.14110737161567));
#86433=CARTESIAN_POINT('Ctrl Pts',(14.8581258282308,2.51349914847505,5.14634674335805));
#86434=CARTESIAN_POINT('Ctrl Pts',(14.7742965886488,2.50876741664099,5.15164069443582));
#86435=CARTESIAN_POINT('Ctrl Pts',(14.690734664194,2.49983913751875,5.1569346455136));
#86436=CARTESIAN_POINT('Ctrl Pts',(14.6078862702578,2.48677563783862,5.16222859659137));
#86437=CARTESIAN_POINT('Ctrl Pts',(14.5257746996796,2.47382832015363,5.1674754652017));
#86438=CARTESIAN_POINT('Ctrl Pts',(14.444364461817,2.45681919966076,5.17272233381203));
#86439=CARTESIAN_POINT('Ctrl Pts',(14.3640783581804,2.4358591739806,5.17796920242236));
#86440=CARTESIAN_POINT('Ctrl Pts',(14.2827115905875,2.41461702296057,5.18328669473385));
#86441=CARTESIAN_POINT('Ctrl Pts',(14.2024999117225,2.38931696199221,5.18860418704535));
#86442=CARTESIAN_POINT('Ctrl Pts',(14.1238643774788,2.3601255519462,5.19392167935684));
#86443=CARTESIAN_POINT('Ctrl Pts',(14.0452288432351,2.3309341419002,5.19923917166833));
#86444=CARTESIAN_POINT('Ctrl Pts',(13.9681698749681,2.29785163286193,5.20455666397982));
#86445=CARTESIAN_POINT('Ctrl Pts',(13.8930827918329,2.26109277657146,5.20987415629132));
#86446=CARTESIAN_POINT('Ctrl Pts',(13.818967537694,2.22480967883919,5.21512282593718));
#86447=CARTESIAN_POINT('Ctrl Pts',(13.7465001655502,2.18481109152274,5.22037149558304));
#86448=CARTESIAN_POINT('Ctrl Pts',(13.6760781339948,2.14126998361096,5.22562016522891));
#86449=CARTESIAN_POINT('Ctrl Pts',(13.6057473964787,2.0977853217222,5.23086203058012));
#86450=CARTESIAN_POINT('Ctrl Pts',(13.5374571258062,2.05076749601277,5.23610389593133));
#86451=CARTESIAN_POINT('Ctrl Pts',(13.4715822306485,2.00043629549423,5.24134576128255));
#86452=CARTESIAN_POINT('Ctrl Pts',(13.4057727555764,1.95015507868241,5.246582420959));
#86453=CARTESIAN_POINT('Ctrl Pts',(13.3423742584481,1.89656729989107,5.25181908063545));
#86454=CARTESIAN_POINT('Ctrl Pts',(13.2817333769281,1.83993642880321,5.2570557403119));
#86455=CARTESIAN_POINT('Ctrl Pts',(13.2211343290392,1.78334462500638,5.26228878743386));
#86456=CARTESIAN_POINT('Ctrl Pts',(13.163289454592,1.72371421395633,5.26752183455582));
#86457=CARTESIAN_POINT('Ctrl Pts',(13.1085118484535,1.66134849521679,5.27275488167778));
#86458=CARTESIAN_POINT('Ctrl Pts',(13.0537414455995,1.59899097760267,5.27798724065124));
#86459=CARTESIAN_POINT('Ctrl Pts',(13.0020378243509,1.53389920553269,5.2832195996247));
#86460=CARTESIAN_POINT('Ctrl Pts',(12.9536760086717,1.46641207459365,5.28845195859816));
#86461=CARTESIAN_POINT('Ctrl Pts',(12.9053194971707,1.39893234543989,5.29368374370224));
#86462=CARTESIAN_POINT('Ctrl Pts',(12.8603043270388,1.32905815925125,5.29891552880632));
#86463=CARTESIAN_POINT('Ctrl Pts',(12.8188630687219,1.25715867614815,5.30414731391041));
#86464=CARTESIAN_POINT('Ctrl Pts',(12.7773933060078,1.18520973867258,5.30938269757513));
#86465=CARTESIAN_POINT('Ctrl Pts',(12.7395025915379,1.11123312576133,5.31461808123984));
#86466=CARTESIAN_POINT('Ctrl Pts',(12.7053778834278,1.03562328678803,5.31985346490456));
#86467=CARTESIAN_POINT('Ctrl Pts',(12.6812025435737,0.982058182360065,5.32356242496225));
#86468=CARTESIAN_POINT('Ctrl Pts',(12.6589163547355,0.927673907001395,5.32727138501995));
#86469=CARTESIAN_POINT('Ctrl Pts',(12.6385710119932,0.872616401748844,5.33098034507765));
#86470=CARTESIAN_POINT('Origin',(-15.,0.,3.));
#86471=CARTESIAN_POINT('',(-17.5174999720511,0.000375130022130284,4.11258330252632));
#86472=CARTESIAN_POINT('Ctrl Pts',(-17.3614291890287,0.872615857753804,
5.05624492860065));
#86473=CARTESIAN_POINT('Ctrl Pts',(-17.3327792589059,0.950146859115319,
5.05098830411758));
#86474=CARTESIAN_POINT('Ctrl Pts',(-17.3002548807785,1.02640647843984,5.04573167963452));
#86475=CARTESIAN_POINT('Ctrl Pts',(-17.2639892861135,1.10098081834484,5.04047505515146));
#86476=CARTESIAN_POINT('Ctrl Pts',(-17.2277744395237,1.17545080302707,5.0352257864991));
#86477=CARTESIAN_POINT('Ctrl Pts',(-17.1878289755028,1.24823978142076,5.02997651784674));
#86478=CARTESIAN_POINT('Ctrl Pts',(-17.1443349279334,1.3189518440204,5.02472724919438));
#86479=CARTESIAN_POINT('Ctrl Pts',(-17.1008531119921,1.38964402059651,5.01947945676935));
#86480=CARTESIAN_POINT('Ctrl Pts',(-17.0538248976113,1.45826002793457,5.01423166434433));
#86481=CARTESIAN_POINT('Ctrl Pts',(-17.0034791048836,1.52442701573245,5.00898387191931));
#86482=CARTESIAN_POINT('Ctrl Pts',(-16.9532069480364,1.59049722753091,5.00374375492842));
#86483=CARTESIAN_POINT('Ctrl Pts',(-16.8996271665276,1.65412519481614,4.99850363793753));
#86484=CARTESIAN_POINT('Ctrl Pts',(-16.8430110295824,1.71496839470516,4.99326352094664));
#86485=CARTESIAN_POINT('Ctrl Pts',(-16.7864128081436,1.7757923414837,4.98802506212875));
#86486=CARTESIAN_POINT('Ctrl Pts',(-16.7267804534695,1.83383293379899,4.98278660331086));
#86487=CARTESIAN_POINT('Ctrl Pts',(-16.6644242655098,1.88878217759019,4.97754814449297));
#86488=CARTESIAN_POINT('Ctrl Pts',(-16.6020690354947,1.94373057722563,4.97230976615072));
#86489=CARTESIAN_POINT('Ctrl Pts',(-16.5369904021032,1.99558741882749,4.96707138780846));
#86490=CARTESIAN_POINT('Ctrl Pts',(-16.4695330877559,2.04408384221165,4.9618330094662));
#86491=CARTESIAN_POINT('Ctrl Pts',(-16.4018694773153,2.09272857601661,4.95657861126017));
#86492=CARTESIAN_POINT('Ctrl Pts',(-16.331812990079,2.13799203022439,4.95132421305414));
#86493=CARTESIAN_POINT('Ctrl Pts',(-16.2597407645321,2.17964663562147,4.94606981484811));
#86494=CARTESIAN_POINT('Ctrl Pts',(-16.1877848051222,2.22123404425838,4.94082389298059));
#86495=CARTESIAN_POINT('Ctrl Pts',(-16.1138200329979,2.25922405593769,4.93557797111307));
#86496=CARTESIAN_POINT('Ctrl Pts',(-16.0382448064517,2.29343715237112,4.93033204924555));
#86497=CARTESIAN_POINT('Ctrl Pts',(-15.9624864087051,2.32773317087077,4.92507341287026));
#86498=CARTESIAN_POINT('Ctrl Pts',(-15.8851101795222,2.35823379105163,4.91981477649497));
#86499=CARTESIAN_POINT('Ctrl Pts',(-15.8065340626515,2.38480797042086,4.91455614011968));
#86500=CARTESIAN_POINT('Ctrl Pts',(-15.7279579457808,2.41138214979008,4.90929750374439));
#86501=CARTESIAN_POINT('Ctrl Pts',(-15.6481824004284,2.43402982120515,4.9040388673691));
#86502=CARTESIAN_POINT('Ctrl Pts',(-15.5676352687526,2.45267128895581,4.89878023099381));
#86503=CARTESIAN_POINT('Ctrl Pts',(-15.487116541093,2.47130618300806,4.89352344901594));
#86504=CARTESIAN_POINT('Ctrl Pts',(-15.4055315770578,2.48600601948482,4.88826666703806));
#86505=CARTESIAN_POINT('Ctrl Pts',(-15.3232992948241,2.49665452475232,4.88300988506018));
#86506=CARTESIAN_POINT('Ctrl Pts',(-15.2411830485188,2.50728800417886,4.87776052079662));
#86507=CARTESIAN_POINT('Ctrl Pts',(-15.158421751876,2.51388144903671,4.87251115653306));
#86508=CARTESIAN_POINT('Ctrl Pts',(-15.0754461398187,2.51636923562232,4.8672617922695));
#86509=CARTESIAN_POINT('Ctrl Pts',(-14.9921267381292,2.51886732975751,4.86199067851878));
#86510=CARTESIAN_POINT('Ctrl Pts',(-14.9085916996311,2.51722556004416,4.85671956476805));
#86511=CARTESIAN_POINT('Ctrl Pts',(-14.8252840835758,2.5114299907718,4.85144845101732));
#86512=CARTESIAN_POINT('Ctrl Pts',(-14.7424672432149,2.50566856393045,4.84620839006385));
#86513=CARTESIAN_POINT('Ctrl Pts',(-14.6598756179712,2.49580217612066,4.84096832911037));
#86514=CARTESIAN_POINT('Ctrl Pts',(-14.577944408213,2.48186932118541,4.8357282681569));
#86515=CARTESIAN_POINT('Ctrl Pts',(-14.4960398725376,2.46794100232533,4.83048991319336));
#86516=CARTESIAN_POINT('Ctrl Pts',(-14.4147957795282,2.44994892302203,4.82525155822983));
#86517=CARTESIAN_POINT('Ctrl Pts',(-14.3346399292213,2.4279831601997,4.8200132032663));
#86518=CARTESIAN_POINT('Ctrl Pts',(-14.2544860384891,2.40601793437565,4.81477497636513));
#86519=CARTESIAN_POINT('Ctrl Pts',(-14.1754207819724,2.38007934109304,4.80953674946397));
#86520=CARTESIAN_POINT('Ctrl Pts',(-14.0978581791351,2.35030772135193,4.80429852256281));
#86521=CARTESIAN_POINT('Ctrl Pts',(-14.0194506653589,2.32021179110205,4.79900323420358));
#86522=CARTESIAN_POINT('Ctrl Pts',(-13.9425791976959,2.28619897293829,4.79370794584435));
#86523=CARTESIAN_POINT('Ctrl Pts',(-13.8676504069068,2.24846406442746,4.78841265748512));
#86524=CARTESIAN_POINT('Ctrl Pts',(-13.793422954735,2.21108235724662,4.78316693338788));
#86525=CARTESIAN_POINT('Ctrl Pts',(-13.7211023392919,2.17004823056789,4.77792120929063));
#86526=CARTESIAN_POINT('Ctrl Pts',(-13.6510571864243,2.12559627768362,4.77267548519338));
#86527=CARTESIAN_POINT('Ctrl Pts',(-13.5800193003584,2.08051431790306,4.76735541470316));
#86528=CARTESIAN_POINT('Ctrl Pts',(-13.51132228214,2.03191717762586,4.76203534421294));
#86529=CARTESIAN_POINT('Ctrl Pts',(-13.4453168195322,1.9800925378301,4.75671527372273));
#86530=CARTESIAN_POINT('Ctrl Pts',(-13.3793113569244,1.92826789803434,4.75139520323251));
#86531=CARTESIAN_POINT('Ctrl Pts',(-13.3159977760365,1.87321612704899,4.74607513274229));
#86532=CARTESIAN_POINT('Ctrl Pts',(-13.2556874259808,1.81526303717081,4.74075506225207));
#86533=CARTESIAN_POINT('Ctrl Pts',(-13.1960969185787,1.75800165453635,4.73549849021039));
#86534=CARTESIAN_POINT('Ctrl Pts',(-13.1392196674876,1.6976977798114,4.73024191816871));
#86535=CARTESIAN_POINT('Ctrl Pts',(-13.085381905456,1.63463873747217,4.72498534612703));
#86536=CARTESIAN_POINT('Ctrl Pts',(-13.0316201585583,1.57166873006624,4.71973619599542));
#86537=CARTESIAN_POINT('Ctrl Pts',(-12.980889673235,1.50595162989935,4.71448704586381));
#86538=CARTESIAN_POINT('Ctrl Pts',(-12.9334807161726,1.43781233113695,4.70923789573219));
#86539=CARTESIAN_POINT('Ctrl Pts',(-12.8858729106628,1.36938723419194,4.70396672897295));
#86540=CARTESIAN_POINT('Ctrl Pts',(-12.8416149007883,1.29851989865549,4.6986955622137));
#86541=CARTESIAN_POINT('Ctrl Pts',(-12.8009604323891,1.22557383705823,4.69342439545446));
#86542=CARTESIAN_POINT('Ctrl Pts',(-12.7605475893236,1.15306132230515,4.68818455729149));
#86543=CARTESIAN_POINT('Ctrl Pts',(-12.7236957990021,1.07849512938316,4.68294471912852));
#86544=CARTESIAN_POINT('Ctrl Pts',(-12.6906105599817,1.00226077661048,4.67770488096555));
#86545=CARTESIAN_POINT('Ctrl Pts',(-12.6575361103228,0.926051284471185,
4.6724667515558));
#86546=CARTESIAN_POINT('Ctrl Pts',(-12.6282259558573,0.848175135617082,
4.66722862214605));
#86547=CARTESIAN_POINT('Ctrl Pts',(-12.6028383473798,0.769039830702783,
4.66199049273629));
#86548=CARTESIAN_POINT('Ctrl Pts',(-12.5774513715141,0.689906497692163,
4.65675249385092));
#86549=CARTESIAN_POINT('Ctrl Pts',(-12.5559868871348,0.609514510427808,
4.65151449496555));
#86550=CARTESIAN_POINT('Ctrl Pts',(-12.5385535162026,0.528287286806343,
4.64627649608018));
#86551=CARTESIAN_POINT('Ctrl Pts',(-12.5209286000478,0.446167597425535,
4.64098094586603));
#86552=CARTESIAN_POINT('Ctrl Pts',(-12.5074240417744,0.363194671680445,
4.63568539565187));
#86553=CARTESIAN_POINT('Ctrl Pts',(-12.4980988283269,0.27981561282562,4.63038984543772));
#86554=CARTESIAN_POINT('Ctrl Pts',(-12.4888617644595,0.197224721347708,
4.62514435311554));
#86555=CARTESIAN_POINT('Ctrl Pts',(-12.4837253326637,0.114235811919584,
4.61989886079337));
#86556=CARTESIAN_POINT('Ctrl Pts',(-12.482694406598,0.0312857703605018,
4.6146533684712));
#86557=CARTESIAN_POINT('Ctrl Pts',(-12.4816487232943,-0.0528516633340902,
4.60933278931105));
#86558=CARTESIAN_POINT('Ctrl Pts',(-12.4848269926099,-0.136948615955238,
4.60401221015091));
#86559=CARTESIAN_POINT('Ctrl Pts',(-12.4921797979398,-0.220554039043703,
4.59869163099077));
#86560=CARTESIAN_POINT('Ctrl Pts',(-12.4995326032696,-0.304159462132168,
4.59337105183062));
#86561=CARTESIAN_POINT('Ctrl Pts',(-12.5110598141303,-0.38727288095522,
4.58805047267048));
#86562=CARTESIAN_POINT('Ctrl Pts',(-12.5266585556508,-0.469455375583696,
4.58272989351034));
#86563=CARTESIAN_POINT('Ctrl Pts',(-12.5420700921414,-0.550651574212894,
4.57747316816679));
#86564=CARTESIAN_POINT('Ctrl Pts',(-12.5615124562054,-0.631236973215575,
4.57221644282324));
#86565=CARTESIAN_POINT('Ctrl Pts',(-12.5849231616556,-0.710781341125662,
4.56695971747969));
#86566=CARTESIAN_POINT('Ctrl Pts',(-12.6083008235378,-0.790213434344449,
4.56171041185964));
#86567=CARTESIAN_POINT('Ctrl Pts',(-12.6356355718122,-0.868606976466571,
4.55646110623958));
#86568=CARTESIAN_POINT('Ctrl Pts',(-12.6668138050427,-0.94554134212144,
4.55121180061953));
#86569=CARTESIAN_POINT('Ctrl Pts',(-12.6981216531792,-1.02279554118366,
4.54594067245907));
#86570=CARTESIAN_POINT('Ctrl Pts',(-12.7333049283758,-1.09857794117082,
4.54066954429862));
#86571=CARTESIAN_POINT('Ctrl Pts',(-12.7721977519031,-1.17247745964443,
4.53539841613816));
#86572=CARTESIAN_POINT('Ctrl Pts',(-12.8108608814067,-1.24594054084748,
4.53015841831299));
#86573=CARTESIAN_POINT('Ctrl Pts',(-12.8531896473533,-1.31754250667629,
4.52491842048781));
#86574=CARTESIAN_POINT('Ctrl Pts',(-12.8989733665958,-1.38690062215215,
4.51967842266263));
#86575=CARTESIAN_POINT('Ctrl Pts',(-12.9447421664479,-1.45623613612651,
4.51444013237836));
#86576=CARTESIAN_POINT('Ctrl Pts',(-12.993963429686,-1.52332886746602,4.50920184209408));
#86577=CARTESIAN_POINT('Ctrl Pts',(-13.04638225176,-1.58782365008259,4.5039635518098));
#86578=CARTESIAN_POINT('Ctrl Pts',(-13.0987997776424,-1.65231683789809,
4.49872539105586));
#86579=CARTESIAN_POINT('Ctrl Pts',(-13.154414413487,-1.71421184757884,4.49348723030191));
#86580=CARTESIAN_POINT('Ctrl Pts',(-13.2129308127959,-1.77318638900303,
4.48824906954797));
#86581=CARTESIAN_POINT('Ctrl Pts',(-13.2720862178385,-1.83280493912491,
4.48295370748302));
#86582=CARTESIAN_POINT('Ctrl Pts',(-13.3342068223973,-1.88943849383192,
4.47765834541808));
#86583=CARTESIAN_POINT('Ctrl Pts',(-13.3989503966091,-1.94279345723676,
4.47236298335313));
#86584=CARTESIAN_POINT('Ctrl Pts',(-13.463086228857,-1.99564758251758,4.46711732836384));
#86585=CARTESIAN_POINT('Ctrl Pts',(-13.5297955828649,-2.04528418147697,
4.46187167337454));
#86586=CARTESIAN_POINT('Ctrl Pts',(-13.5987151606304,-2.09146050619011,
4.45662601838525));
#86587=CARTESIAN_POINT('Ctrl Pts',(-13.6686143464734,-2.13829317126612,
4.45130580278248));
#86588=CARTESIAN_POINT('Ctrl Pts',(-13.7407866586839,-2.18156617012225,
4.4459855871797));
#86589=CARTESIAN_POINT('Ctrl Pts',(-13.8148274004604,-2.22107455059496,
4.44066537157692));
#86590=CARTESIAN_POINT('Ctrl Pts',(-13.888868142237,-2.26058293106766,4.43534515597415));
#86591=CARTESIAN_POINT('Ctrl Pts',(-13.9647768449265,-2.29632654319577,
4.43002494037137));
#86592=CARTESIAN_POINT('Ctrl Pts',(-14.0421297747511,-2.32815181669531,
4.42470472476859));
#86593=CARTESIAN_POINT('Ctrl Pts',(-14.1185591457568,-2.35959711089642,
4.41944803012165));
#86594=CARTESIAN_POINT('Ctrl Pts',(-14.1966787820551,-2.38733251946412,
4.4141913354747));
#86595=CARTESIAN_POINT('Ctrl Pts',(-14.2760941871876,-2.41117536155635,
4.40893464082776));
#86596=CARTESIAN_POINT('Ctrl Pts',(-14.3553974971509,-2.43498454937946,
4.4036853660268));
#86597=CARTESIAN_POINT('Ctrl Pts',(-14.4359925049753,-2.45491195290006,
4.39843609122585));
#86598=CARTESIAN_POINT('Ctrl Pts',(-14.517464837691,-2.47082295341763,4.3931868164249));
#86599=CARTESIAN_POINT('Ctrl Pts',(-14.5992764688284,-2.48680021664284,
4.38791568057498));
#86600=CARTESIAN_POINT('Ctrl Pts',(-14.6819723137276,-2.49872736740562,
4.38264454472506));
#86601=CARTESIAN_POINT('Ctrl Pts',(-14.7651174257217,-2.506518786345,4.37737340887515));
#86602=CARTESIAN_POINT('Ctrl Pts',(-14.8477708899315,-2.51426413361802,
4.37213344193221));
#86603=CARTESIAN_POINT('Ctrl Pts',(-14.930867858799,-2.51792248063566,4.36689347498927));
#86604=CARTESIAN_POINT('Ctrl Pts',(-15.0139726641947,-2.51746122406191,
4.36165350804633));
#86605=CARTESIAN_POINT('Ctrl Pts',(-15.0970503890841,-2.51700011779309,
4.35641524859741));
#86606=CARTESIAN_POINT('Ctrl Pts',(-15.1801354846832,-2.51242207668247,
4.35117698914848));
#86607=CARTESIAN_POINT('Ctrl Pts',(-15.2627912183508,-2.50374659771266,
4.34593872969956));
#86608=CARTESIAN_POINT('Ctrl Pts',(-15.3454449095488,-2.4950713331188,4.34070059969096));
#86609=CARTESIAN_POINT('Ctrl Pts',(-15.4276688014327,-2.48229888118847,
4.33546246968237));
#86610=CARTESIAN_POINT('Ctrl Pts',(-15.5090316067901,-2.46550057255899,
4.33022433967377));
#86611=CARTESIAN_POINT('Ctrl Pts',(-15.591283954079,-2.44851860752976,4.32492894103653));
#86612=CARTESIAN_POINT('Ctrl Pts',(-15.6726557964936,-2.42742229782486,
4.31963354239929));
#86613=CARTESIAN_POINT('Ctrl Pts',(-15.7527142546424,-2.40233792395204,
4.31433814376204));
#86614=CARTESIAN_POINT('Ctrl Pts',(-15.83202020704,-2.3774893294839,4.30909251897782));
#86615=CARTESIAN_POINT('Ctrl Pts',(-15.9100369455761,-2.3487275469003,4.3038468941936));
#86616=CARTESIAN_POINT('Ctrl Pts',(-15.9863626897743,-2.31622427545806,
4.29860126940938));
#86617=CARTESIAN_POINT('Ctrl Pts',(-16.0637747754083,-2.28325838618039,
4.29328098384563));
#86618=CARTESIAN_POINT('Ctrl Pts',(-16.1394469105356,-2.24644388140251,
4.28796069828187));
#86619=CARTESIAN_POINT('Ctrl Pts',(-16.2129863368797,-2.20600779612022,
4.28264041271812));
#86620=CARTESIAN_POINT('Ctrl Pts',(-16.2865257632238,-2.16557171083793,
4.27732012715437));
#86621=CARTESIAN_POINT('Ctrl Pts',(-16.3579320991304,-2.12151435572198,
4.27199984159062));
#86622=CARTESIAN_POINT('Ctrl Pts',(-16.4268452282784,-2.07410678233767,
4.26667955602687));
#86623=CARTESIAN_POINT('Ctrl Pts',(-16.4946545814488,-2.02745853219561,
4.26144448504373));
#86624=CARTESIAN_POINT('Ctrl Pts',(-16.5603033967977,-1.97739226031036,
4.2562094140606));
#86625=CARTESIAN_POINT('Ctrl Pts',(-16.6234248823249,-1.92413562449436,
4.25097434307746));
#86626=CARTESIAN_POINT('Ctrl Pts',(-16.6864570895403,-1.87095431425895,
4.24574667651925));
#86627=CARTESIAN_POINT('Ctrl Pts',(-16.7469687131128,-1.81459189887532,
4.24051900996103));
#86628=CARTESIAN_POINT('Ctrl Pts',(-16.8046221950517,-1.75531905451028,
4.23529134340281));
#86629=CARTESIAN_POINT('Ctrl Pts',(-16.8622102350915,-1.6961134901667,4.23006961071738));
#86630=CARTESIAN_POINT('Ctrl Pts',(-16.9169462578319,-1.63400439384777,
4.22484787803195));
#86631=CARTESIAN_POINT('Ctrl Pts',(-16.9685271800743,-1.56930143417665,
4.21962614534652));
#86632=CARTESIAN_POINT('Ctrl Pts',(-17.0200762519165,-1.50463842755525,
4.21440763699807));
#86633=CARTESIAN_POINT('Ctrl Pts',(-17.06847380093,-1.43738509969373,4.20918912864962));
#86634=CARTESIAN_POINT('Ctrl Pts',(-17.1134557013779,-1.36788568539674,
4.20397062030117));
#86635=CARTESIAN_POINT('Ctrl Pts',(-17.1584236734685,-1.2984077911481,4.1987537278304));
#86636=CARTESIAN_POINT('Ctrl Pts',(-17.1999778445977,-1.22668558204242,
4.19353683535962));
#86637=CARTESIAN_POINT('Ctrl Pts',(-17.2378971126337,-1.15309269500148,
4.18831994288885));
#86638=CARTESIAN_POINT('Ctrl Pts',(-17.2758163121788,-1.07949994088627,
4.18310305984098));
#86639=CARTESIAN_POINT('Ctrl Pts',(-17.3101004099534,-1.00403693001966,
4.17788617679312));
#86640=CARTESIAN_POINT('Ctrl Pts',(-17.3405746914721,-0.927101053629093,
4.17266929374526));
#86641=CARTESIAN_POINT('Ctrl Pts',(-17.371078541097,-0.850090529107456,
4.16744734894223));
#86642=CARTESIAN_POINT('Ctrl Pts',(-17.3977650199345,-0.771604718545424,
4.1622254041392));
#86643=CARTESIAN_POINT('Ctrl Pts',(-17.4205081717154,-0.692059564386758,
4.15700345933618));
#86644=CARTESIAN_POINT('Ctrl Pts',(-17.4432623819275,-0.612475732887851,
4.15177897546037));
#86645=CARTESIAN_POINT('Ctrl Pts',(-17.462069340882,-0.531831985657823,
4.14655449158456));
#86646=CARTESIAN_POINT('Ctrl Pts',(-17.4768540464178,-0.450555526815343,
4.14133000770875));
#86647=CARTESIAN_POINT('Ctrl Pts',(-17.4916642936618,-0.369138656681709,
4.13609649813797));
#86648=CARTESIAN_POINT('Ctrl Pts',(-17.5024383459796,-0.287087353593853,
4.13086298856718));
#86649=CARTESIAN_POINT('Ctrl Pts',(-17.5091530374981,-0.204834773449096,
4.12562947899639));
#86650=CARTESIAN_POINT('Ctrl Pts',(-17.514732534348,-0.136487923776358,
4.12128075350637));
#86651=CARTESIAN_POINT('Ctrl Pts',(-17.5175101608992,-0.0680022946564488,
4.11693202801635));
#86652=CARTESIAN_POINT('Ctrl Pts',(-17.5174999720511,0.000375130022128299,
4.11258330252632));
#86653=CARTESIAN_POINT('Ctrl Pts',(-17.5174999720511,0.000375130562157188,
4.11258330249198));
#86654=CARTESIAN_POINT('Ctrl Pts',(-17.5174969036288,0.0209673020875996,
4.1112736640897));
#86655=CARTESIAN_POINT('Ctrl Pts',(-17.5172411859996,0.0415573205068692,
4.10996402568741));
#86656=CARTESIAN_POINT('Ctrl Pts',(-17.5167329489669,0.0621410780745678,
4.10865438728513));
#86657=CARTESIAN_POINT('Ctrl Pts',(-17.5146933424961,0.144745773182198,
4.10339867629233));
#86658=CARTESIAN_POINT('Ctrl Pts',(-17.5085787900268,0.227401427432359,
4.09814296529952));
#86659=CARTESIAN_POINT('Ctrl Pts',(-17.4983811757245,0.309673619776567,
4.09288725430672));
#86660=CARTESIAN_POINT('Ctrl Pts',(-17.4881961889154,0.391843936179619,
4.08763805135131));
#86661=CARTESIAN_POINT('Ctrl Pts',(-17.4739382300675,0.473631279449932,
4.0823888483959));
#86662=CARTESIAN_POINT('Ctrl Pts',(-17.4556511682864,0.554602190487785,
4.07713964544048));
#86663=CARTESIAN_POINT('Ctrl Pts',(-17.4373846463994,0.635482155589933,
4.07189633835148));
#86664=CARTESIAN_POINT('Ctrl Pts',(-17.415098116769,0.715547063496811,4.06665303126248));
#86665=CARTESIAN_POINT('Ctrl Pts',(-17.3888869213139,0.794371152028817,
4.06140972417347));
#86666=CARTESIAN_POINT('Ctrl Pts',(-17.3801667292314,0.820595106365506,
4.05966533044516));
#86667=CARTESIAN_POINT('Ctrl Pts',(-17.3710125657857,0.846681805097609,
4.05792093671685));
#86668=CARTESIAN_POINT('Ctrl Pts',(-17.3614291890287,0.872615857753799,
4.05617654298853));
#86669=CARTESIAN_POINT('',(-17.5174990478294,-0.00218956111536468,4.38741669750802));
#86670=CARTESIAN_POINT('Ctrl Pts',(-17.3578782887762,0.871321062777582,
4.33113094084205));
#86671=CARTESIAN_POINT('Ctrl Pts',(-17.4602182294948,0.591631726374291,
4.3498927182036));
#86672=CARTESIAN_POINT('Ctrl Pts',(-17.515530076098,0.294291473546931,4.36865449556515));
#86673=CARTESIAN_POINT('Ctrl Pts',(-17.518221775146,-0.00218348048635318,
4.3874162729267));
#86674=CARTESIAN_POINT('Ctrl Pts',(-17.5174990478294,-0.00218956111536468,
4.38741669750802));
#86675=CARTESIAN_POINT('Ctrl Pts',(-17.5173973207564,-0.119152639980189,
4.39482064288431));
#86676=CARTESIAN_POINT('Ctrl Pts',(-17.5091409213801,-0.23577079206408,
4.40222458826058));
#86677=CARTESIAN_POINT('Ctrl Pts',(-17.4928938724097,-0.351121618392081,
4.40962853363686));
#86678=CARTESIAN_POINT('Ctrl Pts',(-17.4854916683259,-0.403675799725012,
4.41300179328546));
#86679=CARTESIAN_POINT('Ctrl Pts',(-17.4764314300592,-0.455967350040209,
4.41637505293405));
#86680=CARTESIAN_POINT('Ctrl Pts',(-17.4657317181364,-0.507910763989177,
4.41974831258264));
#86681=CARTESIAN_POINT('Ctrl Pts',(-17.4490575762057,-0.588857976661858,
4.42500510926611));
#86682=CARTESIAN_POINT('Ctrl Pts',(-17.4283625240479,-0.669131684515691,
4.43026190594957));
#86683=CARTESIAN_POINT('Ctrl Pts',(-17.4037157400883,-0.748302673289332,
4.43551870263304));
#86684=CARTESIAN_POINT('Ctrl Pts',(-17.3791037492572,-0.827361898743446,
4.44076807845367));
#86685=CARTESIAN_POINT('Ctrl Pts',(-17.3505512434199,-0.905321060575425,
4.44601745427432));
#86686=CARTESIAN_POINT('Ctrl Pts',(-17.3181783604909,-0.981761345211712,
4.45126683009496));
#86687=CARTESIAN_POINT('Ctrl Pts',(-17.2856714400657,-1.0585181251189,4.45653794056285));
#86688=CARTESIAN_POINT('Ctrl Pts',(-17.2493125292196,-1.13374296044936,
4.46180905103074));
#86689=CARTESIAN_POINT('Ctrl Pts',(-17.2092738793896,-1.20702741304689,
4.46708016149863));
#86690=CARTESIAN_POINT('Ctrl Pts',(-17.1694710484767,-1.27988023619848,
4.47232022627525));
#86691=CARTESIAN_POINT('Ctrl Pts',(-17.1260319282515,-1.35081506157744,
4.47756029105186));
#86692=CARTESIAN_POINT('Ctrl Pts',(-17.0791731360148,-1.41945247207302,
4.48280035582848));
#86693=CARTESIAN_POINT('Ctrl Pts',(-17.0323296254735,-1.48806749838096,
4.48803871170331));
#86694=CARTESIAN_POINT('Ctrl Pts',(-16.9820689176839,-1.55438621736842,
4.49327706757815));
#86695=CARTESIAN_POINT('Ctrl Pts',(-16.9286514171008,-1.61805746539338,
4.49851542345298));
#86696=CARTESIAN_POINT('Ctrl Pts',(-16.8752352520899,-1.68172712147643,
4.50375364835569));
#86697=CARTESIAN_POINT('Ctrl Pts',(-16.8186627483982,-1.7427490856614,4.50899187325841));
#86698=CARTESIAN_POINT('Ctrl Pts',(-16.7592342361937,-1.80080569529415,
4.51423009816112));
#86699=CARTESIAN_POINT('Ctrl Pts',(-16.6991584027456,-1.8594946828101,4.51952538009139));
#86700=CARTESIAN_POINT('Ctrl Pts',(-16.6361642955416,-1.91515297357877,
4.52482066202166));
#86701=CARTESIAN_POINT('Ctrl Pts',(-16.5705986478698,-1.96749234745897,
4.53011594395194));
#86702=CARTESIAN_POINT('Ctrl Pts',(-16.5056467332036,-2.01934179403145,
4.53536165893046));
#86703=CARTESIAN_POINT('Ctrl Pts',(-16.4381716337318,-2.06793397575382,
4.54060737390898));
#86704=CARTESIAN_POINT('Ctrl Pts',(-16.3685403852193,-2.11303181803396,
4.5458530888875));
#86705=CARTESIAN_POINT('Ctrl Pts',(-16.2979222144046,-2.15876885704368,
4.55117315429365));
#86706=CARTESIAN_POINT('Ctrl Pts',(-16.2250867211346,-2.20091148074323,
4.55649321969979));
#86707=CARTESIAN_POINT('Ctrl Pts',(-16.1504416994653,-2.23926107145446,
4.56181328510594));
#86708=CARTESIAN_POINT('Ctrl Pts',(-16.075796677796,-2.2776106621657,4.56713335051208));
#86709=CARTESIAN_POINT('Ctrl Pts',(-15.9993425985454,-2.31216707724679,
4.57245341591823));
#86710=CARTESIAN_POINT('Ctrl Pts',(-15.9215054899763,-2.34278336214503,
4.57777348132438));
#86711=CARTESIAN_POINT('Ctrl Pts',(-15.8445922977486,-2.37303623572891,
4.58303039824702));
#86712=CARTESIAN_POINT('Ctrl Pts',(-15.7660467606654,-2.39955297748993,
4.58828731516967));
#86713=CARTESIAN_POINT('Ctrl Pts',(-15.6862662133858,-2.42215708292529,
4.59354423209231));
#86714=CARTESIAN_POINT('Ctrl Pts',(-15.6065982441887,-2.44472929177766,
4.59879373099581));
#86715=CARTESIAN_POINT('Ctrl Pts',(-15.5256991663836,-2.46339970646124,
4.60404322989931));
#86716=CARTESIAN_POINT('Ctrl Pts',(-15.4439854369365,-2.47804018970401,
4.60929272880281));
#86717=CARTESIAN_POINT('Ctrl Pts',(-15.3619357752006,-2.49274086125392,
4.61456380885545));
#86718=CARTESIAN_POINT('Ctrl Pts',(-15.2790651864459,-2.50337821925715,
4.61983488890809));
#86719=CARTESIAN_POINT('Ctrl Pts',(-15.1958098629986,-2.50987345249765,
4.62510596896073));
#86720=CARTESIAN_POINT('Ctrl Pts',(-15.1130423798701,-2.51633062647031,
4.63034616275568));
#86721=CARTESIAN_POINT('Ctrl Pts',(-15.0298951229203,-2.51869404835166,
4.63558635655064));
#86722=CARTESIAN_POINT('Ctrl Pts',(-14.9468042475614,-2.51693791379972,
4.6408265503456));
#86723=CARTESIAN_POINT('Ctrl Pts',(-14.8637404387927,-2.51518235130307,
4.64606503716398));
#86724=CARTESIAN_POINT('Ctrl Pts',(-14.7807334357432,-2.5093099073547,4.65130352398236));
#86725=CARTESIAN_POINT('Ctrl Pts',(-14.6982196453878,-2.49934688820302,
4.65654201080074));
#86726=CARTESIAN_POINT('Ctrl Pts',(-14.615707890731,-2.4893841148491,4.66178036838036));
#86727=CARTESIAN_POINT('Ctrl Pts',(-14.5336897821847,-2.47533102329068,
4.66701872595997));
#86728=CARTESIAN_POINT('Ctrl Pts',(-14.4525954739112,-2.45726566223871,
4.67225708353958));
#86729=CARTESIAN_POINT('Ctrl Pts',(-14.3706222710231,-2.43900451002857,
4.67755221408346));
#86730=CARTESIAN_POINT('Ctrl Pts',(-14.2895934871098,-2.41664367885642,
4.68284734462734));
#86731=CARTESIAN_POINT('Ctrl Pts',(-14.2099398926202,-2.39031614576965,
4.68814247517121));
#86732=CARTESIAN_POINT('Ctrl Pts',(-14.131027608002,-2.36423363439584,4.69338832567233));
#86733=CARTESIAN_POINT('Ctrl Pts',(-14.0534654349526,-2.33425817370456,
4.69863417617345));
#86734=CARTESIAN_POINT('Ctrl Pts',(-13.9776524634773,-2.30056770484286,
4.70388002667457));
#86735=CARTESIAN_POINT('Ctrl Pts',(-13.9007712000801,-2.26640249854467,
4.70919979723983));
#86736=CARTESIAN_POINT('Ctrl Pts',(-13.8256892569259,-2.22841699358774,
4.71451956780508));
#86737=CARTESIAN_POINT('Ctrl Pts',(-13.7527956831576,-2.18684421988622,
4.71983933837034));
#86738=CARTESIAN_POINT('Ctrl Pts',(-13.6799021093894,-2.14527144618471,
4.7251591089356));
#86739=CARTESIAN_POINT('Ctrl Pts',(-13.6091972815012,-2.10011172003563,
4.73047887950086));
#86740=CARTESIAN_POINT('Ctrl Pts',(-13.5410369466336,-2.05164155224831,
4.73579865006611));
#86741=CARTESIAN_POINT('Ctrl Pts',(-13.473696553835,-2.00375446155025,4.74105442588));
#86742=CARTESIAN_POINT('Ctrl Pts',(-13.4085925676905,-1.9524604078873,4.74631020169388));
#86743=CARTESIAN_POINT('Ctrl Pts',(-13.34608980551,-1.8979956055171,4.75156597750776));
#86744=CARTESIAN_POINT('Ctrl Pts',(-13.2836753032737,-1.84360771271447,
4.75681433165797));
#86745=CARTESIAN_POINT('Ctrl Pts',(-13.2238550738078,-1.78605826529202,
4.76206268580818));
#86746=CARTESIAN_POINT('Ctrl Pts',(-13.1669638793344,-1.72562592421854,
4.76731103995839));
#86747=CARTESIAN_POINT('Ctrl Pts',(-13.1098232429645,-1.66492861493858,
4.77258240574378));
#86748=CARTESIAN_POINT('Ctrl Pts',(-13.0556377736257,-1.60132334255888,
4.77785377152917));
#86749=CARTESIAN_POINT('Ctrl Pts',(-13.0047119500196,-1.53513251792973,
4.78312513731457));
#86750=CARTESIAN_POINT('Ctrl Pts',(-12.9540983377516,-1.4693474898979,4.78836418589722));
#86751=CARTESIAN_POINT('Ctrl Pts',(-12.9067048014093,-1.4010088916989,4.79360323447988));
#86752=CARTESIAN_POINT('Ctrl Pts',(-12.8627911517787,-1.33046780836091,
4.79884228306254));
#86753=CARTESIAN_POINT('Ctrl Pts',(-12.8188917901316,-1.25994967665272,
4.80407962703991));
#86754=CARTESIAN_POINT('Ctrl Pts',(-12.7784703100671,-1.18723087437197,
4.80931697101728));
#86755=CARTESIAN_POINT('Ctrl Pts',(-12.7417430134631,-1.11269116683712,
4.81455431499465));
#86756=CARTESIAN_POINT('Ctrl Pts',(-12.7050165957296,-1.0381532430097,4.81979153364433));
#86757=CARTESIAN_POINT('Ctrl Pts',(-12.6719843886013,-0.961794914831745,
4.82502875229401));
#86758=CARTESIAN_POINT('Ctrl Pts',(-12.6428159385109,-0.884018976188743,
4.83026597094369));
#86759=CARTESIAN_POINT('Ctrl Pts',(-12.6133173942567,-0.805362861075901,
4.8355624582657));
#86760=CARTESIAN_POINT('Ctrl Pts',(-12.5877707965439,-0.725257292009281,
4.84085894558771));
#86761=CARTESIAN_POINT('Ctrl Pts',(-12.5663001805094,-0.644136195700586,
4.84615543290973));
#86762=CARTESIAN_POINT('Ctrl Pts',(-12.5450393644627,-0.563807773667335,
4.85140016563964));
#86763=CARTESIAN_POINT('Ctrl Pts',(-12.5277752568343,-0.482484053626239,
4.85664489836955));
#86764=CARTESIAN_POINT('Ctrl Pts',(-12.514576737485,-0.400596375607034,
4.86188963109946));
#86765=CARTESIAN_POINT('Ctrl Pts',(-12.5011828552773,-0.317496606259529,
4.86721199571752));
#86766=CARTESIAN_POINT('Ctrl Pts',(-12.4919759534833,-0.23381653791337,
4.87253436033559));
#86767=CARTESIAN_POINT('Ctrl Pts',(-12.4869732965618,-0.150010125680739,
4.87785672495365));
#86768=CARTESIAN_POINT('Ctrl Pts',(-12.4819706396403,-0.06620371344811,
4.88317908957172));
#86769=CARTESIAN_POINT('Ctrl Pts',(-12.4811721678482,0.0177285526205801,
4.88850145418978));
#86770=CARTESIAN_POINT('Ctrl Pts',(-12.4845403831624,0.10133689386932,4.89382381880785));
#86771=CARTESIAN_POINT('Ctrl Pts',(-12.4878677084383,0.183930232228006,
4.89908157007049));
#86772=CARTESIAN_POINT('Ctrl Pts',(-12.4952732739897,0.266510778938183,
4.90433932133313));
#86773=CARTESIAN_POINT('Ctrl Pts',(-12.5067583652682,0.348643658826417,
4.90959707259578));
#86774=CARTESIAN_POINT('Ctrl Pts',(-12.5182272379199,0.430660555089282,
4.91484739914552));
#86775=CARTESIAN_POINT('Ctrl Pts',(-12.5337641298177,0.512230587528115,
4.92009772569527));
#86776=CARTESIAN_POINT('Ctrl Pts',(-12.5533183550739,0.592920887118621,
4.92534805224501));
#86777=CARTESIAN_POINT('Ctrl Pts',(-12.5729491005826,0.673926946706005,
4.93061892454937));
#86778=CARTESIAN_POINT('Ctrl Pts',(-12.5966286687847,0.754045903688691,
4.93588979685373));
#86779=CARTESIAN_POINT('Ctrl Pts',(-12.6242533434921,0.832846969191615,
4.94116066915808));
#86780=CARTESIAN_POINT('Ctrl Pts',(-12.6517214538202,0.911201425275966,
4.9464016685007));
#86781=CARTESIAN_POINT('Ctrl Pts',(-12.6830899182278,0.988252448999663,
4.95164266784331));
#86782=CARTESIAN_POINT('Ctrl Pts',(-12.7182064727464,1.06359040470633,4.95688366718592));
#86783=CARTESIAN_POINT('Ctrl Pts',(-12.7533115226655,1.13890367880604,4.96212294951505));
#86784=CARTESIAN_POINT('Ctrl Pts',(-12.7921620292958,1.21250458212242,4.96736223184418));
#86785=CARTESIAN_POINT('Ctrl Pts',(-12.8345579389069,1.28400425624248,4.9726015141733));
#86786=CARTESIAN_POINT('Ctrl Pts',(-12.8769527132436,1.35550201574984,4.97784065620534));
#86787=CARTESIAN_POINT('Ctrl Pts',(-12.9228924657952,1.42489826202544,4.98307979823737));
#86788=CARTESIAN_POINT('Ctrl Pts',(-12.9721323109669,1.49183071619249,4.9883189402694));
#86789=CARTESIAN_POINT('Ctrl Pts',(-13.0218893397688,1.55946618576321,4.99361311087609));
#86790=CARTESIAN_POINT('Ctrl Pts',(-13.075015922983,1.62458540544535,4.99890728148277));
#86791=CARTESIAN_POINT('Ctrl Pts',(-13.1312169528721,1.68684799930738,5.00420145208945));
#86792=CARTESIAN_POINT('Ctrl Pts',(-13.1869129908552,1.74855113534443,5.00944805215676));
#86793=CARTESIAN_POINT('Ctrl Pts',(-13.2456280739797,1.8074484890672,5.01469465222407));
#86794=CARTESIAN_POINT('Ctrl Pts',(-13.3070384299949,1.86324646047852,5.01994125229138));
#86795=CARTESIAN_POINT('Ctrl Pts',(-13.3692839908249,1.91980330608318,5.02525920816775));
#86796=CARTESIAN_POINT('Ctrl Pts',(-13.4342983110701,1.97317551832977,5.03057716404411));
#86797=CARTESIAN_POINT('Ctrl Pts',(-13.5017117827493,2.0231012500732,5.03589511992048));
#86798=CARTESIAN_POINT('Ctrl Pts',(-13.5691252544285,2.07302698181663,5.04121307579685));
#86799=CARTESIAN_POINT('Ctrl Pts',(-13.638937437613,2.11950601640244,5.04653103167322));
#86800=CARTESIAN_POINT('Ctrl Pts',(-13.7107523908196,2.16232440957011,5.05184898754958));
#86801=CARTESIAN_POINT('Ctrl Pts',(-13.7817561485304,2.20465914179915,5.05710687373766));
#86802=CARTESIAN_POINT('Ctrl Pts',(-13.8549769818467,2.24357018102277,5.06236475992573));
#86803=CARTESIAN_POINT('Ctrl Pts',(-13.9300512283673,2.27881896518385,5.06762264611381));
#86804=CARTESIAN_POINT('Ctrl Pts',(-14.0050197533126,2.31401811105805,5.07287312800499));
#86805=CARTESIAN_POINT('Ctrl Pts',(-14.0818360932399,2.34556505186817,5.07812360989618));
#86806=CARTESIAN_POINT('Ctrl Pts',(-14.1601098903681,2.37326586242301,5.08337409178736));
#86807=CARTESIAN_POINT('Ctrl Pts',(-14.2386871253636,2.40107405852944,5.08864492780836));
#86808=CARTESIAN_POINT('Ctrl Pts',(-14.3187327372534,2.42500600131077,5.09391576382936));
#86809=CARTESIAN_POINT('Ctrl Pts',(-14.3998292064608,2.44491334582281,5.09918659985036));
#86810=CARTESIAN_POINT('Ctrl Pts',(-14.4804697388657,2.4647087681872,5.1044278024219));
#86811=CARTESIAN_POINT('Ctrl Pts',(-14.5621488918436,2.48052461483988,5.10966900499344));
#86812=CARTESIAN_POINT('Ctrl Pts',(-14.6444403075757,2.49226474418813,5.11491020756499));
#86813=CARTESIAN_POINT('Ctrl Pts',(-14.726705037857,2.5040010664486,5.12014971051996));
#86814=CARTESIAN_POINT('Ctrl Pts',(-14.8095811806631,2.5116642314104,5.12538921347494));
#86815=CARTESIAN_POINT('Ctrl Pts',(-14.8926336900799,2.51520947944583,5.13062871642992));
#86816=CARTESIAN_POINT('Ctrl Pts',(-14.9756842447002,2.51875464403719,5.13586809606337));
#86817=CARTESIAN_POINT('Ctrl Pts',(-15.0589106971921,2.51818206584989,5.14110747569682));
#86818=CARTESIAN_POINT('Ctrl Pts',(-15.141875788897,2.51349905719594,5.14634685533028));
#86819=CARTESIAN_POINT('Ctrl Pts',(-15.2257048666175,2.50876728039258,5.15164079707703));
#86820=CARTESIAN_POINT('Ctrl Pts',(-15.3092666282684,2.49983897237347,5.15693473882378));
#86821=CARTESIAN_POINT('Ctrl Pts',(-15.3921148617149,2.48677545934938,5.16222868057053));
#86822=CARTESIAN_POINT('Ctrl Pts',(-15.4742265400234,2.47382808637122,5.16747555698069));
#86823=CARTESIAN_POINT('Ctrl Pts',(-15.5556368833323,2.45681889943722,5.17272243339085));
#86824=CARTESIAN_POINT('Ctrl Pts',(-15.6359230890096,2.43585879616708,5.17796930980101));
#86825=CARTESIAN_POINT('Ctrl Pts',(-15.7172895652132,2.41461666958296,5.18328678421606));
#86826=CARTESIAN_POINT('Ctrl Pts',(-15.7975009604204,2.38931666101742,5.18860425863111));
#86827=CARTESIAN_POINT('Ctrl Pts',(-15.8761362235756,2.3601253288202,5.19392173304616));
#86828=CARTESIAN_POINT('Ctrl Pts',(-15.9547714867308,2.33093399662298,5.19923920746121));
#86829=CARTESIAN_POINT('Ctrl Pts',(-16.0318301964893,2.29785159087143,5.20455668187626));
#86830=CARTESIAN_POINT('Ctrl Pts',(-16.1069170379196,2.26109285991606,5.20987415629132));
#86831=CARTESIAN_POINT('Ctrl Pts',(-16.1810320417782,2.22480989162625,5.21512280744354));
#86832=CARTESIAN_POINT('Ctrl Pts',(-16.2534991811834,2.18481145602326,5.22037145859576));
#86833=CARTESIAN_POINT('Ctrl Pts',(-16.3239209991794,2.14127051955888,5.22562010974799));
#86834=CARTESIAN_POINT('Ctrl Pts',(-16.3942515227484,2.09778602930612,5.23086195658));
#86835=CARTESIAN_POINT('Ctrl Pts',(-16.4625415986379,2.05076839498171,5.23610380341202));
#86836=CARTESIAN_POINT('Ctrl Pts',(-16.5284163196141,2.00043740315396,5.24134565024404));
#86837=CARTESIAN_POINT('Ctrl Pts',(-16.59422562042,1.95015639502268,5.24658229139918));
#86838=CARTESIAN_POINT('Ctrl Pts',(-16.6576239638578,1.89656884220967,5.25181893255431));
#86839=CARTESIAN_POINT('Ctrl Pts',(-16.7182647135537,1.83993821204854,5.25705557370944));
#86840=CARTESIAN_POINT('Ctrl Pts',(-16.7788636298067,1.78334664892138,5.26228860233126));
#86841=CARTESIAN_POINT('Ctrl Pts',(-16.8367083944421,1.72371649346041,5.26752163095307));
#86842=CARTESIAN_POINT('Ctrl Pts',(-16.8914859137858,1.66135104296163,5.27275465957489));
#86843=CARTESIAN_POINT('Ctrl Pts',(-16.9462562311214,1.59899379211289,5.27798700017148));
#86844=CARTESIAN_POINT('Ctrl Pts',(-16.9979597897181,1.53390229933247,5.28321934076807));
#86845=CARTESIAN_POINT('Ctrl Pts',(-17.0463215667391,1.46641545801271,5.28845168136466));
#86846=CARTESIAN_POINT('Ctrl Pts',(-17.0946780400812,1.39893601775537,5.29368344814748));
#86847=CARTESIAN_POINT('Ctrl Pts',(-17.139693195972,1.32906213074443,5.29891521493029));
#86848=CARTESIAN_POINT('Ctrl Pts',(-17.1811344650775,1.25716295493104,5.3041469817131));
#86849=CARTESIAN_POINT('Ctrl Pts',(-17.2226042404479,1.18521432172907,5.30938234727879));
#86850=CARTESIAN_POINT('Ctrl Pts',(-17.2604949923158,1.11123802103591,5.31461771284448));
#86851=CARTESIAN_POINT('Ctrl Pts',(-17.2946197636733,1.03562850007135,5.31985307841017));
#86852=CARTESIAN_POINT('Ctrl Pts',(-17.3187960910826,0.982061532106858,
5.32356217028064));
#86853=CARTESIAN_POINT('Ctrl Pts',(-17.3410831330273,0.927675332202151,
5.32727126215111));
#86854=CARTESIAN_POINT('Ctrl Pts',(-17.3614291890287,0.872615857753799,
5.33098035402157));
#86855=CARTESIAN_POINT('Origin',(-15.,0.,8.20842344717746));
#86856=CARTESIAN_POINT('',(-18.0734988375387,-0.00267313449380446,4.70842344717746));
#86857=CARTESIAN_POINT('Ctrl Pts',(-13.1256826865589,2.43995710119902,5.35407232013781));
#86858=CARTESIAN_POINT('Ctrl Pts',(-12.4214282668293,1.88987704449842,5.30765840291763));
#86859=CARTESIAN_POINT('Ctrl Pts',(-11.4362126399874,0.0231526869172058,
5.20856942945022));
#86860=CARTESIAN_POINT('Ctrl Pts',(-12.8980243432311,-2.95589590321946,
5.05680539973554));
#86861=CARTESIAN_POINT('Ctrl Pts',(-16.3276370895773,-3.37529447323561,
4.89878023099381));
#86862=CARTESIAN_POINT('Ctrl Pts',(-17.9625769261592,-1.43265780425104,
4.78265291347444));
#86863=CARTESIAN_POINT('Ctrl Pts',(-18.0762683537743,-0.210587979812296,
4.71920065220233));
#86864=CARTESIAN_POINT('Ctrl Pts',(-18.0743812564454,-0.00267390196584321,
4.70842344717746));
#86865=CARTESIAN_POINT('Ctrl Pts',(-18.0734988375387,-0.00267313449380446,
4.70842344717746));
#86866=CARTESIAN_POINT('Ctrl Pts',(-18.0735813825829,0.0922349585720596,
4.70350244085089));
#86867=CARTESIAN_POINT('Ctrl Pts',(-18.0692636450065,0.187280803106169,
4.69858143452432));
#86868=CARTESIAN_POINT('Ctrl Pts',(-18.060534039328,0.282017098975876,4.69366042819775));
#86869=CARTESIAN_POINT('Ctrl Pts',(-18.0518123136726,0.376667878473905,
4.68874386395541));
#86870=CARTESIAN_POINT('Ctrl Pts',(-18.0386866748694,0.471009216033492,
4.68382729971307));
#86871=CARTESIAN_POINT('Ctrl Pts',(-18.0211975937825,0.564594854141415,
4.67891073547073));
#86872=CARTESIAN_POINT('Ctrl Pts',(-18.0037167736861,0.65813628694975,4.67399649357399));
#86873=CARTESIAN_POINT('Ctrl Pts',(-17.9818766860609,0.750922285092664,
4.66908225167725));
#86874=CARTESIAN_POINT('Ctrl Pts',(-17.9557693956204,0.842513815859346,
4.66416800978052));
#86875=CARTESIAN_POINT('Ctrl Pts',(-17.9296668378427,0.934088743147806,
4.65925465872497));
#86876=CARTESIAN_POINT('Ctrl Pts',(-17.8992987380668,1.02446919830555,4.65434130766943));
#86877=CARTESIAN_POINT('Ctrl Pts',(-17.8648075022904,1.11322963705626,4.64942795661389));
#86878=CARTESIAN_POINT('Ctrl Pts',(-17.8303124793768,1.20199982170196,4.64451406607246));
#86879=CARTESIAN_POINT('Ctrl Pts',(-17.7916935870412,1.28914921573111,4.63960017553104));
#86880=CARTESIAN_POINT('Ctrl Pts',(-17.7491415414118,1.37427182001377,4.63468628498961));
#86881=CARTESIAN_POINT('Ctrl Pts',(-17.7065467708575,1.45947989273455,4.62976746059362));
#86882=CARTESIAN_POINT('Ctrl Pts',(-17.6600111677927,1.54265670890348,4.62484863619764));
#86883=CARTESIAN_POINT('Ctrl Pts',(-17.609771422396,1.6234208859212,4.61992981180165));
#86884=CARTESIAN_POINT('Ctrl Pts',(-17.5595035797688,1.70423023135443,4.61500823648919));
#86885=CARTESIAN_POINT('Ctrl Pts',(-17.5055277299802,1.78262388120401,4.61008666117675));
#86886=CARTESIAN_POINT('Ctrl Pts',(-17.448122605106,1.85825131787087,4.60516508586429));
#86887=CARTESIAN_POINT('Ctrl Pts',(-17.390627285648,1.93399757990731,4.60023577780258));
#86888=CARTESIAN_POINT('Ctrl Pts',(-17.3296922277719,2.00696860864084,4.59530646974086));
#86889=CARTESIAN_POINT('Ctrl Pts',(-17.2656347354978,2.07684893415625,4.59037716167914));
#86890=CARTESIAN_POINT('Ctrl Pts',(-17.232508732449,2.1129860946021,4.58782807228954));
#86891=CARTESIAN_POINT('Ctrl Pts',(-17.1985482981898,2.14829736031872,4.58527898289994));
#86892=CARTESIAN_POINT('Ctrl Pts',(-17.1638007572219,2.18274335024668,4.58272989351033));
#86893=CARTESIAN_POINT('Ctrl Pts',(-17.0956315306495,2.25032098096535,4.57772897985392));
#86894=CARTESIAN_POINT('Ctrl Pts',(-17.0241745908414,2.31481993889649,4.5727280661975));
#86895=CARTESIAN_POINT('Ctrl Pts',(-16.949739211895,2.37590388180985,4.56772715254109));
#86896=CARTESIAN_POINT('Ctrl Pts',(-16.8754043569385,2.43690533167016,4.5627329925521));
#86897=CARTESIAN_POINT('Ctrl Pts',(-16.7980993933822,2.49450065668835,4.55773883256311));
#86898=CARTESIAN_POINT('Ctrl Pts',(-16.7181705057759,2.54839015126839,4.55274467257412));
#86899=CARTESIAN_POINT('Ctrl Pts',(-16.6383255019237,2.60222308991171,4.54775575385523));
#86900=CARTESIAN_POINT('Ctrl Pts',(-16.5558624102442,2.65235768582453,4.54276683513634));
#86901=CARTESIAN_POINT('Ctrl Pts',(-16.4711597656437,2.69853500884297,4.53777791641744));
#86902=CARTESIAN_POINT('Ctrl Pts',(-16.3865172554687,2.74467954838925,4.53279253956861));
#86903=CARTESIAN_POINT('Ctrl Pts',(-16.2996387372562,2.78687219081721,4.52780716271978));
#86904=CARTESIAN_POINT('Ctrl Pts',(-16.2109301182278,2.82489831653616,4.52282178587095));
#86905=CARTESIAN_POINT('Ctrl Pts',(-16.1222534637121,2.86291074024294,4.5178382054106));
#86906=CARTESIAN_POINT('Ctrl Pts',(-16.0317484214375,2.89675945764434,4.51285462495025));
#86907=CARTESIAN_POINT('Ctrl Pts',(-15.9398429224663,2.92627707695119,4.5078710444899));
#86908=CARTESIAN_POINT('Ctrl Pts',(-15.8479454918753,2.95579210490739,4.50288790153789));
#86909=CARTESIAN_POINT('Ctrl Pts',(-15.7546482667519,2.98097665682237,4.49790475858587));
#86910=CARTESIAN_POINT('Ctrl Pts',(-15.6603954428957,3.00171286251743,4.49292161563386));
#86911=CARTESIAN_POINT('Ctrl Pts',(-15.5661252060733,3.02245289917303,4.48793755205903));
#86912=CARTESIAN_POINT('Ctrl Pts',(-15.4708994483097,3.0387428632294,4.4829534884842));
#86913=CARTESIAN_POINT('Ctrl Pts',(-15.3751726340627,3.05051598006804,4.47796942490938));
#86914=CARTESIAN_POINT('Ctrl Pts',(-15.2793429939833,3.06230174310773,4.47298000765711));
#86915=CARTESIAN_POINT('Ctrl Pts',(-15.1830116590368,3.06956091934624,4.46799059040484));
#86916=CARTESIAN_POINT('Ctrl Pts',(-15.086638068938,3.07227864865977,4.46300117315258));
#86917=CARTESIAN_POINT('Ctrl Pts',(-14.9902073545031,3.07499798887606,4.45800879848067));
#86918=CARTESIAN_POINT('Ctrl Pts',(-14.8937347733996,3.07317053042643,4.45301642380876));
#86919=CARTESIAN_POINT('Ctrl Pts',(-14.7976774998649,3.06683352269716,4.44802404913685));
#86920=CARTESIAN_POINT('Ctrl Pts',(-14.7014664692317,3.06048637143701,4.44302368326329));
#86921=CARTESIAN_POINT('Ctrl Pts',(-14.6056725090362,3.04961530742927,4.43802331738972));
#86922=CARTESIAN_POINT('Ctrl Pts',(-14.5107453496793,3.03430916966936,4.43302295151615));
#86923=CARTESIAN_POINT('Ctrl Pts',(-14.4581074923707,3.02582179576277,4.43025020926697));
#86924=CARTESIAN_POINT('Ctrl Pts',(-14.4057359491156,3.01597163605999,4.42747746701779));
#86925=CARTESIAN_POINT('Ctrl Pts',(-14.3537053912016,3.00478044599569,4.42470472476861));
#86926=CARTESIAN_POINT('Ctrl Pts',(-14.259856853012,2.98459467689687,4.4197034751704));
#86927=CARTESIAN_POINT('Ctrl Pts',(-14.1667911929647,2.95997271228434,4.41470222557219));
#86928=CARTESIAN_POINT('Ctrl Pts',(-14.0749591752603,2.93098988783053,4.40970097597398));
#86929=CARTESIAN_POINT('Ctrl Pts',(-13.9832739652492,2.90205339690736,4.40470772164731));
#86930=CARTESIAN_POINT('Ctrl Pts',(-13.8928188892288,2.86877004520901,4.39971446732065));
#86931=CARTESIAN_POINT('Ctrl Pts',(-13.8040338573033,2.83126601285062,4.39472121299398));
#86932=CARTESIAN_POINT('Ctrl Pts',(-13.71533125354,2.79379679929444,4.38973259441242));
#86933=CARTESIAN_POINT('Ctrl Pts',(-13.6282960156907,2.75211485854518,4.38474397583087));
#86934=CARTESIAN_POINT('Ctrl Pts',(-13.5433517367207,2.70639577428827,4.37975535724932));
#86935=CARTESIAN_POINT('Ctrl Pts',(-13.4584655126854,2.66070793661422,4.37477014812546));
#86936=CARTESIAN_POINT('Ctrl Pts',(-13.3756677923777,2.61098864655695,4.36978493900161));
#86937=CARTESIAN_POINT('Ctrl Pts',(-13.2953600436244,2.55746062904744,4.36479972987776));
#86938=CARTESIAN_POINT('Ctrl Pts',(-13.2381613227809,2.51933561398523,4.36124904405418));
#86939=CARTESIAN_POINT('Ctrl Pts',(-13.1822253101393,2.47927946661832,4.35769835823061));
#86940=CARTESIAN_POINT('Ctrl Pts',(-13.1276888212995,2.43738653071546,4.35414767240703));
#86941=CARTESIAN_POINT('',(-18.0734992704458,0.00211768020265139,4.79157655282255));
#86942=CARTESIAN_POINT('Ctrl Pts',(-18.0702676004121,0.00213770170989528,
4.791575403523));
#86943=CARTESIAN_POINT('Ctrl Pts',(-18.0725846333099,0.362048543166639,
4.7729831523707));
#86944=CARTESIAN_POINT('Ctrl Pts',(-17.8482361699865,1.73885344748678,4.70171584497116));
#86945=CARTESIAN_POINT('Ctrl Pts',(-15.9143185581385,3.44829888129498,4.58366527076405));
#86946=CARTESIAN_POINT('Ctrl Pts',(-13.8440432611115,2.98320055308787,4.48420694770922));
#86947=CARTESIAN_POINT('Ctrl Pts',(-13.1255958151414,2.44015351965519,4.43742368090164));
#86948=CARTESIAN_POINT('Ctrl Pts',(-13.1276888212995,2.43738653071547,5.43736138633702));
#86949=CARTESIAN_POINT('Ctrl Pts',(-13.0510205330792,2.37849275606065,5.43236854431858));
#86950=CARTESIAN_POINT('Ctrl Pts',(-12.9771508045237,2.31599130424347,5.42737570230014));
#86951=CARTESIAN_POINT('Ctrl Pts',(-12.906424534798,2.25018755251741,5.4223828602817));
#86952=CARTESIAN_POINT('Ctrl Pts',(-12.8356222754107,2.1843130999775,5.41738465385797));
#86953=CARTESIAN_POINT('Ctrl Pts',(-12.7679705386501,2.11512956162114,5.41238644743423));
#86954=CARTESIAN_POINT('Ctrl Pts',(-12.7037777600287,2.04297960701055,5.4073882410105));
#86955=CARTESIAN_POINT('Ctrl Pts',(-12.6395477110153,1.97078776206371,5.40238713262309));
#86956=CARTESIAN_POINT('Ctrl Pts',(-12.5787808943321,1.89562641057895,5.39738602423567));
#86957=CARTESIAN_POINT('Ctrl Pts',(-12.5217444641205,1.81787011331464,5.39238491584826));
#86958=CARTESIAN_POINT('Ctrl Pts',(-12.4646153147323,1.73998741438342,5.3873756775928));
#86959=CARTESIAN_POINT('Ctrl Pts',(-12.4112289040444,1.65950170923796,5.38236643933734));
#86960=CARTESIAN_POINT('Ctrl Pts',(-12.3618081980268,1.57681522887158,5.37735720108188));
#86961=CARTESIAN_POINT('Ctrl Pts',(-12.3307046723726,1.5247754813533,5.37420457573227));
#86962=CARTESIAN_POINT('Ctrl Pts',(-12.3011710274356,1.4718645107532,5.37105195038266));
#86963=CARTESIAN_POINT('Ctrl Pts',(-12.2732531150491,1.41818675618217,5.36789932503305));
#86964=CARTESIAN_POINT('Ctrl Pts',(-12.229020765757,1.333141242874,5.36290439476317));
#86965=CARTESIAN_POINT('Ctrl Pts',(-12.1886920459263,1.24587254939232,5.3579094644933));
#86966=CARTESIAN_POINT('Ctrl Pts',(-12.1524966929214,1.15677446642659,5.35291453422342));
#86967=CARTESIAN_POINT('Ctrl Pts',(-12.1163508613921,1.06779828498065,5.34792643787826));
#86968=CARTESIAN_POINT('Ctrl Pts',(-12.0843273221457,0.97699809214518,5.3429383415331));
#86969=CARTESIAN_POINT('Ctrl Pts',(-12.0566099351616,0.884792165545563,
5.33795024518793));
#86970=CARTESIAN_POINT('Ctrl Pts',(-12.0289220695585,0.79268444612118,5.33296746159077));
#86971=CARTESIAN_POINT('Ctrl Pts',(-12.0055313651088,0.699174388146253,
5.3279846779936));
#86972=CARTESIAN_POINT('Ctrl Pts',(-11.9865731849166,0.604699164987345,
5.32300189439644));
#86973=CARTESIAN_POINT('Ctrl Pts',(-11.9676287900181,0.510292638754096,
5.31802273399171));
#86974=CARTESIAN_POINT('Ctrl Pts',(-11.9531105984872,0.41492277249696,5.31304357358699));
#86975=CARTESIAN_POINT('Ctrl Pts',(-11.9431035598391,0.319039815903618,
5.30806441318226));
#86976=CARTESIAN_POINT('Ctrl Pts',(-11.9331002282061,0.223192378265826,
5.30308709726151));
#86977=CARTESIAN_POINT('Ctrl Pts',(-11.9276047749072,0.126832664968066,
5.29810978134076));
#86978=CARTESIAN_POINT('Ctrl Pts',(-11.926650525246,0.0304180214548819,
5.29313246542001));
#86979=CARTESIAN_POINT('Ctrl Pts',(-11.9256963672343,-0.0659873620615559,
5.28815562753795));
#86980=CARTESIAN_POINT('Ctrl Pts',(-11.9292825499124,-0.162447225441892,
5.28317878965589));
#86981=CARTESIAN_POINT('Ctrl Pts',(-11.9373902825083,-0.258503323625889,
5.27820195177382));
#86982=CARTESIAN_POINT('Ctrl Pts',(-11.9454994611287,-0.354576553536986,
5.2732242262664));
#86983=CARTESIAN_POINT('Ctrl Pts',(-11.9581317540368,-0.450245436929502,
5.26824650075898));
#86984=CARTESIAN_POINT('Ctrl Pts',(-11.9752165244132,-0.545057039048925,
5.26326877525155));
#86985=CARTESIAN_POINT('Ctrl Pts',(-11.9923196282558,-0.639970382384078,
5.2582857082054));
#86986=CARTESIAN_POINT('Ctrl Pts',(-12.0138846697799,-0.734024174307596,
5.25330264115925));
#86987=CARTESIAN_POINT('Ctrl Pts',(-12.0397899523229,-0.826776102479868,
5.2483195741131));
#86988=CARTESIAN_POINT('Ctrl Pts',(-12.0657105249464,-0.919582775642581,
5.24333356591022));
#86989=CARTESIAN_POINT('Ctrl Pts',(-12.0959763010442,-1.01108563773112,
5.23834755770734));
#86990=CARTESIAN_POINT('Ctrl Pts',(-12.1304164882122,-1.10085999058721,
5.23336154950445));
#86991=CARTESIAN_POINT('Ctrl Pts',(-12.1649121265169,-1.19077888649965,
5.22836751347579));
#86992=CARTESIAN_POINT('Ctrl Pts',(-12.2035954191685,-1.2789633138907,5.22337347744712));
#86993=CARTESIAN_POINT('Ctrl Pts',(-12.2462485114045,-1.36501098495866,
5.21837944141845));
#86994=CARTESIAN_POINT('Ctrl Pts',(-12.2704625077885,-1.41385991681506,
5.21554434637608));
#86995=CARTESIAN_POINT('Ctrl Pts',(-12.2959550612654,-1.46202069568636,
5.2127092513337));
#86996=CARTESIAN_POINT('Ctrl Pts',(-12.3226801324512,-1.50942392217305,
5.20987415629133));
#86997=CARTESIAN_POINT('Ctrl Pts',(-12.3698321797499,-1.59305921585964,
5.20487209157818));
#86998=CARTESIAN_POINT('Ctrl Pts',(-12.4209889291442,-1.67462839778874,
5.19987002686503));
#86999=CARTESIAN_POINT('Ctrl Pts',(-12.4759444281291,-1.75372338756921,
5.19486796215188));
#87000=CARTESIAN_POINT('Ctrl Pts',(-12.5308257731993,-1.83271165093968,
5.18987264694854));
#87001=CARTESIAN_POINT('Ctrl Pts',(-12.5894954322247,-1.90923200048418,
5.1848773317452));
#87002=CARTESIAN_POINT('Ctrl Pts',(-12.6517019533244,-1.98290154419724,
5.17988201654187));
#87003=CARTESIAN_POINT('Ctrl Pts',(-12.7138432361192,-2.05649382790485,
5.17489194011239));
#87004=CARTESIAN_POINT('Ctrl Pts',(-12.7795137256188,-2.12724091618579,
5.16990186368291));
#87005=CARTESIAN_POINT('Ctrl Pts',(-12.8484197281198,-2.1947903279484,5.16491178725343));
#87006=CARTESIAN_POINT('Ctrl Pts',(-12.9172768052121,-2.26229177752404,
5.15992525393369));
#87007=CARTESIAN_POINT('Ctrl Pts',(-12.9893645160051,-2.32659975821772,
5.15493872061394));
#87008=CARTESIAN_POINT('Ctrl Pts',(-13.0643507490039,-2.38739695633515,
5.1499521872942));
#87009=CARTESIAN_POINT('Ctrl Pts',(-13.1393099497156,-2.44817223726517,
5.14496745160312));
#87010=CARTESIAN_POINT('Ctrl Pts',(-13.2171652562067,-2.50543897454987,
5.13998271591203));
#87011=CARTESIAN_POINT('Ctrl Pts',(-13.2975504868493,-2.55891928461466,
5.13499798022094));
#87012=CARTESIAN_POINT('Ctrl Pts',(-13.3779286184244,-2.61239487166843,
5.13001368474722));
#87013=CARTESIAN_POINT('Ctrl Pts',(-13.4608358647743,-2.66208445369521,
5.12502938927351));
#87014=CARTESIAN_POINT('Ctrl Pts',(-13.5458768866329,-2.70775335309025,
5.12004509379979));
#87015=CARTESIAN_POINT('Ctrl Pts',(-13.6309335446414,-2.7534306494418,5.11505988188375));
#87016=CARTESIAN_POINT('Ctrl Pts',(-13.7181243710789,-2.79508558755098,
5.11007466996771));
#87017=CARTESIAN_POINT('Ctrl Pts',(-13.8070302054619,-2.83252984438289,
5.10508945805167));
#87018=CARTESIAN_POINT('Ctrl Pts',(-13.8960312768007,-2.87001421193485,
5.10009890591909));
#87019=CARTESIAN_POINT('Ctrl Pts',(-13.9867506189721,-2.90327872310088,
5.09510835378651));
#87020=CARTESIAN_POINT('Ctrl Pts',(-14.0787501182962,-2.93218364115564,
5.09011780165394));
#87021=CARTESIAN_POINT('Ctrl Pts',(-14.170804026667,-2.96110565374948,5.08512429807938));
#87022=CARTESIAN_POINT('Ctrl Pts',(-14.2641391759466,-2.98566282778118,
5.08013079450483));
#87023=CARTESIAN_POINT('Ctrl Pts',(-14.3583054066296,-3.00576617501083,
5.07513729093028));
#87024=CARTESIAN_POINT('Ctrl Pts',(-14.4526219465686,-3.02590161144211,
5.07013581666601));
#87025=CARTESIAN_POINT('Ctrl Pts',(-14.5477717844515,-3.04156895477625,
5.06513434240174));
#87026=CARTESIAN_POINT('Ctrl Pts',(-14.6432978387497,-3.05273087876402,
5.06013286813747));
#87027=CARTESIAN_POINT('Ctrl Pts',(-14.696037383467,-3.05889333144365,5.05737157460817));
#87028=CARTESIAN_POINT('Ctrl Pts',(-14.7488915569139,-3.0636834119157,5.05461028107888));
#87029=CARTESIAN_POINT('Ctrl Pts',(-14.8017835631764,-3.0671016439259,5.05184898754958));
#87030=CARTESIAN_POINT('Ctrl Pts',(-14.8975915662202,-3.07329339209314,
5.04684721057884));
#87031=CARTESIAN_POINT('Ctrl Pts',(-14.9938563775379,-3.07500241943791,
5.04184543360811));
#87032=CARTESIAN_POINT('Ctrl Pts',(-15.0901237054268,-3.07217837498413,
5.03684365663737));
#87033=CARTESIAN_POINT('Ctrl Pts',(-15.1862614035205,-3.06935813327748,
5.03184861486266));
#87034=CARTESIAN_POINT('Ctrl Pts',(-15.2824011768329,-3.06201696431892,
5.02685357308795));
#87035=CARTESIAN_POINT('Ctrl Pts',(-15.3780849852503,-3.05015638843785,
5.02185853131324));
#87036=CARTESIAN_POINT('Ctrl Pts',(-15.4736687214783,-3.03830821709854,
5.01686871366971));
#87037=CARTESIAN_POINT('Ctrl Pts',(-15.568797007958,-3.02195008915829,5.01187889602618));
#87038=CARTESIAN_POINT('Ctrl Pts',(-15.6630142108175,-3.00113551947493,
5.00688907838265));
#87039=CARTESIAN_POINT('Ctrl Pts',(-15.7571649491824,-2.98033563320194,
5.00190278075136));
#87040=CARTESIAN_POINT('Ctrl Pts',(-15.8504054546709,-2.95508564923108,
4.99691648312007));
#87041=CARTESIAN_POINT('Ctrl Pts',(-15.9422885710765,-2.92549047149681,
4.99193018548879));
#87042=CARTESIAN_POINT('Ctrl Pts',(-16.0341388282225,-2.89590587759627,
4.98694567105831));
#87043=CARTESIAN_POINT('Ctrl Pts',(-16.1246322438638,-2.86197931184187,
4.98196115662784));
#87044=CARTESIAN_POINT('Ctrl Pts',(-16.2133360878607,-2.82386575245617,
4.97697664219736));
#87045=CARTESIAN_POINT('Ctrl Pts',(-16.3020323605703,-2.78575544624075,
4.97199255321847));
#87046=CARTESIAN_POINT('Ctrl Pts',(-16.3889389625577,-2.74345903026862,
4.96700846423958));
#87047=CARTESIAN_POINT('Ctrl Pts',(-16.4736434362022,-2.69717950328451,
4.96202437526069));
#87048=CARTESIAN_POINT('Ctrl Pts',(-16.5583637416606,-2.65089132635758,
4.95703935472334));
#87049=CARTESIAN_POINT('Ctrl Pts',(-16.6408807165536,-2.60061877010777,
4.95205433418599));
#87050=CARTESIAN_POINT('Ctrl Pts',(-16.7208077281701,-2.54661010220842,
4.94706931364865));
#87051=CARTESIAN_POINT('Ctrl Pts',(-16.8008207528596,-2.49254331313833,
4.94207892850519));
#87052=CARTESIAN_POINT('Ctrl Pts',(-16.8782378861775,-2.43473263176821,
4.93708854336173));
#87053=CARTESIAN_POINT('Ctrl Pts',(-16.952702846875,-2.37346873621838,4.93209815821828));
#87054=CARTESIAN_POINT('Ctrl Pts',(-17.0272120506079,-2.31216844098918,
4.927104808059));
#87055=CARTESIAN_POINT('Ctrl Pts',(-17.0987652641845,-2.24741114029537,
4.92211145789973));
#87056=CARTESIAN_POINT('Ctrl Pts',(-17.1670421439888,-2.17952531441518,
4.91711810774046));
#87057=CARTESIAN_POINT('Ctrl Pts',(-17.2354283256271,-2.11153081272407,
4.91211676391873));
#87058=CARTESIAN_POINT('Ctrl Pts',(-17.3005274050842,-2.04039810889525,
4.907115420097));
#87059=CARTESIAN_POINT('Ctrl Pts',(-17.3620585382765,-1.96648969276608,
4.90211407627527));
#87060=CARTESIAN_POINT('Ctrl Pts',(-17.3960566632211,-1.92565268171733,
4.89935065711946));
#87061=CARTESIAN_POINT('Ctrl Pts',(-17.4289662609585,-1.88396880226838,
4.89658723796366));
#87062=CARTESIAN_POINT('Ctrl Pts',(-17.4607457414077,-1.84150282273583,
4.89382381880785));
#87063=CARTESIAN_POINT('Ctrl Pts',(-17.5184291891083,-1.76442213813061,
4.88880789211252));
#87064=CARTESIAN_POINT('Ctrl Pts',(-17.5725898992664,-1.68449167440274,
4.88379196541719));
#87065=CARTESIAN_POINT('Ctrl Pts',(-17.6229351526086,-1.60206536546108,
4.87877603872186));
#87066=CARTESIAN_POINT('Ctrl Pts',(-17.6732122760822,-1.51975060017493,
4.87376689984472));
#87067=CARTESIAN_POINT('Ctrl Pts',(-17.7196839777768,-1.43494706825674,
4.86875776096759));
#87068=CARTESIAN_POINT('Ctrl Pts',(-17.762098714886,-1.34804040711883,4.86374862209045));
#87069=CARTESIAN_POINT('Ctrl Pts',(-17.8044673660001,-1.26122817495158,
4.85874492592417));
#87070=CARTESIAN_POINT('Ctrl Pts',(-17.8427876244817,-1.17231774389179,
4.85374122975788));
#87071=CARTESIAN_POINT('Ctrl Pts',(-17.8768526283568,-1.08172140808836,
4.8487375335916));
#87072=CARTESIAN_POINT('Ctrl Pts',(-17.9108890317255,-0.991201135716088,
4.84373803845945));
#87073=CARTESIAN_POINT('Ctrl Pts',(-17.9406771326098,-0.898998178990735,
4.8387385433273));
#87074=CARTESIAN_POINT('Ctrl Pts',(-17.9660576270989,-0.805546027690952,
4.83373904819515));
#87075=CARTESIAN_POINT('Ctrl Pts',(-17.991425186168,-0.712141505203933,
4.82874210110512));
#87076=CARTESIAN_POINT('Ctrl Pts',(-18.012389492138,-0.617489473104872,
4.82374515401509));
#87077=CARTESIAN_POINT('Ctrl Pts',(-18.0288409625587,-0.522038957862991,
4.81874820692505));
#87078=CARTESIAN_POINT('Ctrl Pts',(-18.0452922989824,-0.426589220063481,
4.81375130053505));
#87079=CARTESIAN_POINT('Ctrl Pts',(-18.0572307877008,-0.330341438581802,
4.80875439414504));
#87080=CARTESIAN_POINT('Ctrl Pts',(-18.0645980267115,-0.233754539369315,
4.80375748775503));
#87081=CARTESIAN_POINT('Ctrl Pts',(-18.070584387873,-0.155271397813929,
4.79969717611087));
#87082=CARTESIAN_POINT('Ctrl Pts',(-18.0735534835641,-0.0765646343269345,
4.79563686446671));
#87083=CARTESIAN_POINT('Ctrl Pts',(-18.0734992704458,0.00211768020265139,
4.79157655282255));
#87084=CARTESIAN_POINT('Origin',(15.,0.,8.20842344717745));
#87085=CARTESIAN_POINT('',(11.9265011624444,-0.00267311509943158,4.70842344717746));
#87086=CARTESIAN_POINT('Ctrl Pts',(16.8743174193178,2.43995797974749,5.35407234097178));
#87087=CARTESIAN_POINT('Ctrl Pts',(17.5785721639147,1.88987785061309,5.30765841680695));
#87088=CARTESIAN_POINT('Ctrl Pts',(18.5637879643976,0.0231525210448785,
5.20856943639487));
#87089=CARTESIAN_POINT('Ctrl Pts',(17.1019761085213,-2.95589625912284,5.05680539973555));
#87090=CARTESIAN_POINT('Ctrl Pts',(13.6723626328074,-3.37529520198335,4.8987802309938));
#87091=CARTESIAN_POINT('Ctrl Pts',(12.0374225320172,-1.43265805207317,4.78265291347445));
#87092=CARTESIAN_POINT('Ctrl Pts',(11.9237310852615,-0.210587998618168,
4.71920065220233));
#87093=CARTESIAN_POINT('Ctrl Pts',(11.9256181828774,-0.00267388305352438,
4.70842344717746));
#87094=CARTESIAN_POINT('Ctrl Pts',(11.9265011624444,-0.00267311509943158,
4.70842344717746));
#87095=CARTESIAN_POINT('Ctrl Pts',(11.9264186179886,0.0922349900664025,
4.70350244021915));
#87096=CARTESIAN_POINT('Ctrl Pts',(11.9307363572755,0.187280846398732,4.69858143326084));
#87097=CARTESIAN_POINT('Ctrl Pts',(11.9394659657117,0.282017153668012,4.69366042630253));
#87098=CARTESIAN_POINT('Ctrl Pts',(11.9481876941353,0.37666794469639,4.6887438614217));
#87099=CARTESIAN_POINT('Ctrl Pts',(11.9613133367653,0.471009293387588,4.68382729654086));
#87100=CARTESIAN_POINT('Ctrl Pts',(11.9788024226627,0.564594942140883,4.67891073166003));
#87101=CARTESIAN_POINT('Ctrl Pts',(11.9962832475833,0.658136385675146,4.6739964891206));
#87102=CARTESIAN_POINT('Ctrl Pts',(12.0181233410234,0.750922394056947,4.66908224658118));
#87103=CARTESIAN_POINT('Ctrl Pts',(12.0442306381959,0.842513934496294,4.66416800404175));
#87104=CARTESIAN_POINT('Ctrl Pts',(12.0703332027249,0.934088871527253,4.65925465233979));
#87105=CARTESIAN_POINT('Ctrl Pts',(12.1007013101754,1.02446933585973,4.65434130063783));
#87106=CARTESIAN_POINT('Ctrl Pts',(12.1351925544778,1.11322978314479,4.64942794893587));
#87107=CARTESIAN_POINT('Ctrl Pts',(12.1696875859408,1.20199997638338,4.64451405774477));
#87108=CARTESIAN_POINT('Ctrl Pts',(12.2083064876828,1.28914937836292,4.63960016655367));
#87109=CARTESIAN_POINT('Ctrl Pts',(12.2508585435057,1.37427198988562,4.63468627536257));
#87110=CARTESIAN_POINT('Ctrl Pts',(12.2934533242757,1.4594800698779,4.62976745031486));
#87111=CARTESIAN_POINT('Ctrl Pts',(12.3399889383471,1.54265689260553,4.62484862526715));
#87112=CARTESIAN_POINT('Ctrl Pts',(12.3902286954731,1.62342107540458,4.61992980021943));
#87113=CARTESIAN_POINT('Ctrl Pts',(12.440496549854,1.70423042665118,4.61500822425314));
#87114=CARTESIAN_POINT('Ctrl Pts',(12.4944724121225,1.78262408153428,4.61008664828685));
#87115=CARTESIAN_POINT('Ctrl Pts',(12.551877550136,1.85825152239187,4.60516507232055));
#87116=CARTESIAN_POINT('Ctrl Pts',(12.6093728827216,1.93399778858301,4.60023576360674));
#87117=CARTESIAN_POINT('Ctrl Pts',(12.6703079543828,2.00696882062901,4.59530645489292));
#87118=CARTESIAN_POINT('Ctrl Pts',(12.7343654610338,2.07684914855259,4.59037714617911));
#87119=CARTESIAN_POINT('Ctrl Pts',(12.7674913999929,2.11298623221784,4.58782806195618));
#87120=CARTESIAN_POINT('Ctrl Pts',(12.8014517667167,2.14829742447959,4.58527897773326));
#87121=CARTESIAN_POINT('Ctrl Pts',(12.836199237003,2.18274334452163,4.58272989351033));
#87122=CARTESIAN_POINT('Ctrl Pts',(12.9043684592838,2.25032097134355,4.57772898013236));
#87123=CARTESIAN_POINT('Ctrl Pts',(12.9758253945357,2.31481992588043,4.5727280667544));
#87124=CARTESIAN_POINT('Ctrl Pts',(13.0502607687252,2.37590386590618,4.56772715337643));
#87125=CARTESIAN_POINT('Ctrl Pts',(13.1245956188818,2.43690531284224,4.56273299366883));
#87126=CARTESIAN_POINT('Ctrl Pts',(13.2019005774341,2.49450063544591,4.55773883396123));
#87127=CARTESIAN_POINT('Ctrl Pts',(13.2818294598922,2.5483901281212,4.55274467425363));
#87128=CARTESIAN_POINT('Ctrl Pts',(13.3616744585565,2.60222306483138,4.54775575581865));
#87129=CARTESIAN_POINT('Ctrl Pts',(13.4441375449011,2.65235765932386,4.54276683738367));
#87130=CARTESIAN_POINT('Ctrl Pts',(13.528840184076,2.69853498143165,4.53777791894869));
#87131=CARTESIAN_POINT('Ctrl Pts',(13.6134826887818,2.74467952004211,4.53279254238636));
#87132=CARTESIAN_POINT('Ctrl Pts',(13.7003612014318,2.78687216204757,4.52780716582402));
#87133=CARTESIAN_POINT('Ctrl Pts',(13.7890698148569,2.82489828785204,4.52282178926169));
#87134=CARTESIAN_POINT('Ctrl Pts',(13.8777464637431,2.86291071163217,4.51783820908933));
#87135=CARTESIAN_POINT('Ctrl Pts',(13.9682515003463,2.89675942961718,4.51285462891697));
#87136=CARTESIAN_POINT('Ctrl Pts',(14.0601569936535,2.9262770500111,4.50787104874461));
#87137=CARTESIAN_POINT('Ctrl Pts',(14.1520544185593,2.95579207904727,4.50288790608174));
#87138=CARTESIAN_POINT('Ctrl Pts',(14.2453516380043,2.98097663254759,4.49790476341887));
#87139=CARTESIAN_POINT('Ctrl Pts',(14.3396044562356,3.0017128403257,4.492921620756));
#87140=CARTESIAN_POINT('Ctrl Pts',(14.4338746874182,3.02245287906166,4.48793755747111));
#87141=CARTESIAN_POINT('Ctrl Pts',(14.5291004395952,3.03874284569756,4.48295349418622));
#87142=CARTESIAN_POINT('Ctrl Pts',(14.6248272483537,3.05051596560683,4.47796943090132));
#87143=CARTESIAN_POINT('Ctrl Pts',(14.720656882956,3.06230173172257,4.47298001393841));
#87144=CARTESIAN_POINT('Ctrl Pts',(14.8169882125238,3.06956091152766,4.46799059697549));
#87145=CARTESIAN_POINT('Ctrl Pts',(14.9133617973856,3.0722786448901,4.46300118001257));
#87146=CARTESIAN_POINT('Ctrl Pts',(15.0097925065817,3.07499798915774,4.45800880563012));
#87147=CARTESIAN_POINT('Ctrl Pts',(15.1062650825882,3.07317053524227,4.45301643124767));
#87148=CARTESIAN_POINT('Ctrl Pts',(15.2023223512108,3.06683353252187,4.44802405686522));
#87149=CARTESIAN_POINT('Ctrl Pts',(15.2985333769842,3.06048638627462,4.44302369127844));
#87150=CARTESIAN_POINT('Ctrl Pts',(15.3943273325049,3.04961532775035,4.43802332569166));
#87151=CARTESIAN_POINT('Ctrl Pts',(15.4892544874145,3.03430919593649,4.43302296010487));
#87152=CARTESIAN_POINT('Ctrl Pts',(15.5418923996255,3.0258218160769,4.43025021499278));
#87153=CARTESIAN_POINT('Ctrl Pts',(15.5942639972722,3.01597164759197,4.42747746988069));
#87154=CARTESIAN_POINT('Ctrl Pts',(15.6462946088311,3.00478044598868,4.4247047247686));
#87155=CARTESIAN_POINT('Ctrl Pts',(15.7401431465919,2.98459467698101,4.41970347518578));
#87156=CARTESIAN_POINT('Ctrl Pts',(15.833208806245,2.95997271249419,4.41470222560295));
#87157=CARTESIAN_POINT('Ctrl Pts',(15.9250408235919,2.93098988819278,4.40970097602012));
#87158=CARTESIAN_POINT('Ctrl Pts',(16.0167260332122,2.90205339743246,4.40470772171066));
#87159=CARTESIAN_POINT('Ctrl Pts',(16.107181108879,2.86877004592674,4.39971446740119));
#87160=CARTESIAN_POINT('Ctrl Pts',(16.1959661404893,2.83126601378307,4.39472121309172));
#87161=CARTESIAN_POINT('Ctrl Pts',(16.2846687439218,2.79379680044808,4.38973259452824));
#87162=CARTESIAN_POINT('Ctrl Pts',(16.3717039814793,2.75211485994354,4.38474397596476));
#87163=CARTESIAN_POINT('Ctrl Pts',(16.4566482601966,2.70639577594747,4.37975535740128));
#87164=CARTESIAN_POINT('Ctrl Pts',(16.541534483932,2.66070793855956,4.37477014829827));
#87165=CARTESIAN_POINT('Ctrl Pts',(16.6243322039809,2.61098864880902,4.36978493919526));
#87166=CARTESIAN_POINT('Ctrl Pts',(16.7046399525167,2.55746063161955,4.36479973009225));
#87167=CARTESIAN_POINT('Ctrl Pts',(16.7618385480427,2.51933570021064,4.36124905205315));
#87168=CARTESIAN_POINT('Ctrl Pts',(16.8177744409165,2.47927964495925,4.35769837401405));
#87169=CARTESIAN_POINT('Ctrl Pts',(16.8723108164276,2.43738680900022,4.35414769597494));
#87170=CARTESIAN_POINT('',(11.9265007295358,0.00211765345701963,4.79157655282255));
#87171=CARTESIAN_POINT('Ctrl Pts',(11.9297330560105,0.002137679106189,4.791575403287));
#87172=CARTESIAN_POINT('Ctrl Pts',(11.9274160148606,0.362048478990828,4.77298315221337));
#87173=CARTESIAN_POINT('Ctrl Pts',(12.151764398138,1.73885322680167,4.70171584489249));
#87174=CARTESIAN_POINT('Ctrl Pts',(14.0856815469411,3.44829792336913,4.58366527839654));
#87175=CARTESIAN_POINT('Ctrl Pts',(16.1559561762778,2.98319997967846,4.48420696297422));
#87176=CARTESIAN_POINT('Ctrl Pts',(16.8744034286678,2.4401532777456,4.43742370379915));
#87177=CARTESIAN_POINT('Ctrl Pts',(16.8723108164276,2.43738680900022,5.43736140735745));
#87178=CARTESIAN_POINT('Ctrl Pts',(16.9489792105581,2.37849297110846,5.4323685573755));
#87179=CARTESIAN_POINT('Ctrl Pts',(17.0228490367164,2.31599144785443,5.42737570739354));
#87180=CARTESIAN_POINT('Ctrl Pts',(17.0935753952956,2.25018761755837,5.42238285741159));
#87181=CARTESIAN_POINT('Ctrl Pts',(17.1643777456509,2.18431308448554,5.41738464287325));
#87182=CARTESIAN_POINT('Ctrl Pts',(17.2320295644332,2.11512945825866,5.41238642833491));
#87183=CARTESIAN_POINT('Ctrl Pts',(17.2962224157258,2.04297940946999,5.40738821379658));
#87184=CARTESIAN_POINT('Ctrl Pts',(17.3604525385292,1.97078746908027,5.40238709720602));
#87185=CARTESIAN_POINT('Ctrl Pts',(17.4212194195263,1.89562601573753,5.39738598061546));
#87186=CARTESIAN_POINT('Ctrl Pts',(17.4782559042015,1.81786961119069,5.3923848640249));
#87187=CARTESIAN_POINT('Ctrl Pts',(17.53538510908,1.73998680352338,5.38737561747068));
#87188=CARTESIAN_POINT('Ctrl Pts',(17.588771565254,1.65950098411322,5.38236637091647));
#87189=CARTESIAN_POINT('Ctrl Pts',(17.6381923063921,1.57681438492086,5.37735712436226));
#87190=CARTESIAN_POINT('Ctrl Pts',(17.6692955503182,1.52477507096333,5.37420452458586));
#87191=CARTESIAN_POINT('Ctrl Pts',(17.6988289401045,1.47186454914168,5.37105192480945));
#87192=CARTESIAN_POINT('Ctrl Pts',(17.7267466251365,1.41818725572712,5.36789932503305));
#87193=CARTESIAN_POINT('Ctrl Pts',(17.7709788012614,1.33314211342738,5.3629044141584));
#87194=CARTESIAN_POINT('Ctrl Pts',(17.8113073878468,1.24587379722512,5.35790950328374));
#87195=CARTESIAN_POINT('Ctrl Pts',(17.8475026461821,1.15677609328071,5.35291459240909));
#87196=CARTESIAN_POINT('Ctrl Pts',(17.88364838107,1.06780029551037,5.34792651572261));
#87197=CARTESIAN_POINT('Ctrl Pts',(17.9156718626184,0.977000488300628,5.34293843903613));
#87198=CARTESIAN_POINT('Ctrl Pts',(17.9433892292822,0.884794945140182,5.33795036234965));
#87199=CARTESIAN_POINT('Ctrl Pts',(17.9710770731585,0.792687613497772,5.33296759864726));
#87200=CARTESIAN_POINT('Ctrl Pts',(17.9944677936174,0.699177941269497,5.32798483494486));
#87201=CARTESIAN_POINT('Ctrl Pts',(18.0134260258391,0.604703098053697,5.32300207124247));
#87202=CARTESIAN_POINT('Ctrl Pts',(18.0323704716355,0.510296956937685,5.31802293100551));
#87203=CARTESIAN_POINT('Ctrl Pts',(18.0468887505391,0.414927470116671,5.31304379076856));
#87204=CARTESIAN_POINT('Ctrl Pts',(18.0568959112316,0.319044883826335,5.3080646505316));
#87205=CARTESIAN_POINT('Ctrl Pts',(18.0668993645224,0.223197819625414,5.30308735494101));
#87206=CARTESIAN_POINT('Ctrl Pts',(18.0723949744294,0.126838470676509,5.29811005935043));
#87207=CARTESIAN_POINT('Ctrl Pts',(18.0733494138018,0.0304241792676716,
5.29313276375984));
#87208=CARTESIAN_POINT('Ctrl Pts',(18.0743037614796,-0.06598084944974,5.28815594634684));
#87209=CARTESIAN_POINT('Ctrl Pts',(18.0707178018187,-0.162440370266277,
5.28317912893384));
#87210=CARTESIAN_POINT('Ctrl Pts',(18.0626103237388,-0.258496141032276,
5.27820231152084));
#87211=CARTESIAN_POINT('Ctrl Pts',(18.0545013998621,-0.354569041308425,
5.27322460659797));
#87212=CARTESIAN_POINT('Ctrl Pts',(18.0418693934093,-0.450237610231264,
5.2682469016751));
#87213=CARTESIAN_POINT('Ctrl Pts',(18.0247849393674,-0.545048915764779,
5.26326919675224));
#87214=CARTESIAN_POINT('Ctrl Pts',(18.0076821523099,-0.639961961578314,
5.25828615034515));
#87215=CARTESIAN_POINT('Ctrl Pts',(17.9861174575717,-0.734015473909388,
5.25330310393805));
#87216=CARTESIAN_POINT('Ctrl Pts',(17.9602125500155,-0.826767142991621,
5.24832005753096));
#87217=CARTESIAN_POINT('Ctrl Pts',(17.9342923528586,-0.919573555986063,
5.24333407002904));
#87218=CARTESIAN_POINT('Ctrl Pts',(17.9040269805487,-1.01107617845491,5.23834808252711));
#87219=CARTESIAN_POINT('Ctrl Pts',(17.8695872237241,-1.10085031472934,5.23336209502518));
#87220=CARTESIAN_POINT('Ctrl Pts',(17.8350920155099,-1.1907689961763,5.2283680795939));
#87221=CARTESIAN_POINT('Ctrl Pts',(17.7964091793615,-1.27895323211523,5.22337406416262));
#87222=CARTESIAN_POINT('Ctrl Pts',(17.753756568313,-1.36500073716947,5.21838004873134));
#87223=CARTESIAN_POINT('Ctrl Pts',(17.7295410162616,-1.41385326427879,5.21554475125133));
#87224=CARTESIAN_POINT('Ctrl Pts',(17.7040467218771,-1.46201754260581,5.21270945377133));
#87225=CARTESIAN_POINT('Ctrl Pts',(17.6773197348229,-1.50942415759379,5.20987415629132));
#87226=CARTESIAN_POINT('Ctrl Pts',(17.6301675940733,-1.59305959984705,5.20487208308445));
#87227=CARTESIAN_POINT('Ctrl Pts',(17.5790107393177,-1.67462891798103,5.19987000987758));
#87228=CARTESIAN_POINT('Ctrl Pts',(17.5240551248562,-1.75372403093742,5.19486793667072));
#87229=CARTESIAN_POINT('Ctrl Pts',(17.46917366344,-1.83271241879279,5.18987261289182));
#87230=CARTESIAN_POINT('Ctrl Pts',(17.4105038778397,-1.90923287973844,5.18487728911293));
#87231=CARTESIAN_POINT('Ctrl Pts',(17.3482972216521,-1.98290252125038,5.17988196533404));
#87232=CARTESIAN_POINT('Ctrl Pts',(17.2861558029351,-2.05649490381021,5.17489188025963));
#87233=CARTESIAN_POINT('Ctrl Pts',(17.2204851689074,-2.12724207728245,5.16990179518521));
#87234=CARTESIAN_POINT('Ctrl Pts',(17.1515790149052,-2.19479156017599,5.16491171011079));
#87235=CARTESIAN_POINT('Ctrl Pts',(17.0827217854077,-2.26229308182359,5.15992516807901));
#87236=CARTESIAN_POINT('Ctrl Pts',(17.0106339151512,-2.32660112045707,5.15493862604722));
#87237=CARTESIAN_POINT('Ctrl Pts',(16.9356475171831,-2.38739836207175,5.14995208401543));
#87238=CARTESIAN_POINT('Ctrl Pts',(16.860688150942,-2.44817368698582,5.14496733957423));
#87239=CARTESIAN_POINT('Ctrl Pts',(16.7828326733712,-2.50544045376631,5.13998259513302));
#87240=CARTESIAN_POINT('Ctrl Pts',(16.7024472675756,-2.55892077859485,5.13499785069181));
#87241=CARTESIAN_POINT('Ctrl Pts',(16.6220689604118,-2.61239638071116,5.13001354644078));
#87242=CARTESIAN_POINT('Ctrl Pts',(16.5391615343711,-2.66208596303015,5.12502924218975));
#87243=CARTESIAN_POINT('Ctrl Pts',(16.4541203301321,-2.70775484774686,5.12004493793871));
#87244=CARTESIAN_POINT('Ctrl Pts',(16.3690634894584,-2.75343212955223,5.11505971722903));
#87245=CARTESIAN_POINT('Ctrl Pts',(16.2818724776512,-2.79508703811668,5.11007449651934));
#87246=CARTESIAN_POINT('Ctrl Pts',(16.1929664565577,-2.83253125022976,5.10508927580965));
#87247=CARTESIAN_POINT('Ctrl Pts',(16.1039651989865,-2.87001557272939,5.10009871491203));
#87248=CARTESIAN_POINT('Ctrl Pts',(16.0132456692638,-2.90328002370169,5.0951081540144));
#87249=CARTESIAN_POINT('Ctrl Pts',(15.9212459823961,-2.93218486625912,5.09011759311678));
#87250=CARTESIAN_POINT('Ctrl Pts',(15.8291918865314,-2.96110680326053,5.08512408078071));
#87251=CARTESIAN_POINT('Ctrl Pts',(15.7358565497685,-2.98566388639374,5.08013056844464));
#87252=CARTESIAN_POINT('Ctrl Pts',(15.6416901329319,-3.00576712725685,5.07513705610856));
#87253=CARTESIAN_POINT('Ctrl Pts',(15.5473734085243,-3.02590245672863,5.0701355731739));
#87254=CARTESIAN_POINT('Ctrl Pts',(15.45222338754,-3.0415696777737,5.06513409023924));
#87255=CARTESIAN_POINT('Ctrl Pts',(15.3566971528226,-3.05273146397914,5.06013260730458));
#87256=CARTESIAN_POINT('Ctrl Pts',(15.3039592605239,-3.05889363587365,5.05737140071958));
#87257=CARTESIAN_POINT('Ctrl Pts',(15.2511067479274,-3.06368352204467,5.05461019413458));
#87258=CARTESIAN_POINT('Ctrl Pts',(15.1982164035266,-3.06710164607777,5.05184898754958));
#87259=CARTESIAN_POINT('Ctrl Pts',(15.1024083595404,-3.07329339584653,5.04684720877601));
#87260=CARTESIAN_POINT('Ctrl Pts',(15.006143508681,-3.07500242085317,5.04184543000244));
#87261=CARTESIAN_POINT('Ctrl Pts',(14.9098761430184,-3.0721783705382,5.03684365122887));
#87262=CARTESIAN_POINT('Ctrl Pts',(14.8137384062145,-3.06935812294928,5.03184860760245));
#87263=CARTESIAN_POINT('Ctrl Pts',(14.7175985959546,-3.06201694450271,5.02685356397604));
#87264=CARTESIAN_POINT('Ctrl Pts',(14.6219147526597,-3.05015635595024,5.02185852034962));
#87265=CARTESIAN_POINT('Ctrl Pts',(14.52633098067,-3.03830817183864,5.01686870080825));
#87266=CARTESIAN_POINT('Ctrl Pts',(14.4312026605024,-3.02195002786311,5.01187888126688));
#87267=CARTESIAN_POINT('Ctrl Pts',(14.3369854262807,-3.00113543930223,5.00688906172551));
#87268=CARTESIAN_POINT('Ctrl Pts',(14.2428346553922,-2.98033553390359,5.00190276213505));
#87269=CARTESIAN_POINT('Ctrl Pts',(14.1495941197248,-2.95508552785747,4.99691646254458));
#87270=CARTESIAN_POINT('Ctrl Pts',(14.0577109756917,-2.92549032551266,4.99193016295412));
#87271=CARTESIAN_POINT('Ctrl Pts',(13.9658606902278,-2.89590570678482,4.98694564652717));
#87272=CARTESIAN_POINT('Ctrl Pts',(13.8753672488383,-2.86197911360387,4.98196113010021));
#87273=CARTESIAN_POINT('Ctrl Pts',(13.7866633818244,-2.82386552459466,4.97697661367326));
#87274=CARTESIAN_POINT('Ctrl Pts',(13.697967085474,-2.78575518848935,4.9719925226629));
#87275=CARTESIAN_POINT('Ctrl Pts',(13.6110604626015,-2.74345874037196,4.96700843165253));
#87276=CARTESIAN_POINT('Ctrl Pts',(13.5263559709507,-2.69717917937375,4.96202434064216));
#87277=CARTESIAN_POINT('Ctrl Pts',(13.4416356469328,-2.65089096812596,4.95703931804061));
#87278=CARTESIAN_POINT('Ctrl Pts',(13.3591186563884,-2.60061837563425,4.95205429543906));
#87279=CARTESIAN_POINT('Ctrl Pts',(13.2791916321199,-2.54660966994035,4.94706927283751));
#87280=CARTESIAN_POINT('Ctrl Pts',(13.1991785941939,-2.49254284264924,4.94207888559201));
#87281=CARTESIAN_POINT('Ctrl Pts',(13.1217614506819,-2.43473212144877,4.93708849834652));
#87282=CARTESIAN_POINT('Ctrl Pts',(13.0472964829005,-2.37346818481038,4.93209811110102));
#87283=CARTESIAN_POINT('Ctrl Pts',(12.9727872717327,-2.31216784818284,4.92710475881522));
#87284=CARTESIAN_POINT('Ctrl Pts',(12.9012340538619,-2.24741050479877,4.92211140652942));
#87285=CARTESIAN_POINT('Ctrl Pts',(12.8329571729522,-2.17952463526812,4.91711805424361));
#87286=CARTESIAN_POINT('Ctrl Pts',(12.7645709900054,-2.11153008965672,4.91211670827724));
#87287=CARTESIAN_POINT('Ctrl Pts',(12.6994719124577,-2.04039734092574,4.90711536231086));
#87288=CARTESIAN_POINT('Ctrl Pts',(12.6379407844251,-1.96648887922559,4.90211401634449));
#87289=CARTESIAN_POINT('Ctrl Pts',(12.6039429226847,-1.92565215572201,4.89935061716561));
#87290=CARTESIAN_POINT('Ctrl Pts',(12.5710335724665,-1.883968576587,4.89658721798673));
#87291=CARTESIAN_POINT('Ctrl Pts',(12.5392543229165,-1.84150290869026,4.89382381880785));
#87292=CARTESIAN_POINT('Ctrl Pts',(12.4815709191545,-1.76442228841168,4.88880789574964));
#87293=CARTESIAN_POINT('Ctrl Pts',(12.4274102455408,-1.68449189134849,4.88379197269143));
#87294=CARTESIAN_POINT('Ctrl Pts',(12.3770650214843,-1.60206565048959,4.87877604963322));
#87295=CARTESIAN_POINT('Ctrl Pts',(12.3267879278441,-1.51975095415582,4.87376691444681));
#87296=CARTESIAN_POINT('Ctrl Pts',(12.2803162486563,-1.43494749266234,4.8687577792604));
#87297=CARTESIAN_POINT('Ctrl Pts',(12.2379015269199,-1.34804090257257,4.86374864407399));
#87298=CARTESIAN_POINT('Ctrl Pts',(12.1955328916047,-1.26122874228337,4.85874495164671));
#87299=CARTESIAN_POINT('Ctrl Pts',(12.1572126417202,-1.1723183837677,4.85374125921942));
#87300=CARTESIAN_POINT('Ctrl Pts',(12.1231476394767,-1.08172212039477,4.84873756679214));
#87301=CARTESIAN_POINT('Ctrl Pts',(12.0891112381515,-0.991201921491761,
4.84373807545658));
#87302=CARTESIAN_POINT('Ctrl Pts',(12.0593231322546,-0.898999038163477,
4.83873858412102));
#87303=CARTESIAN_POINT('Ctrl Pts',(12.0339426259614,-0.805546959469903,
4.83373909278546));
#87304=CARTESIAN_POINT('Ctrl Pts',(12.0085750552694,-0.7121425101975,4.82874214952462));
#87305=CARTESIAN_POINT('Ctrl Pts',(11.9876107308319,-0.617490550540763,
4.82374520626377));
#87306=CARTESIAN_POINT('Ctrl Pts',(11.9711592353833,-0.522040106309965,
4.81874826300292));
#87307=CARTESIAN_POINT('Ctrl Pts',(11.9547078740308,-0.426590440095431,
4.81375136047214));
#87308=CARTESIAN_POINT('Ctrl Pts',(11.9427693537697,-0.330342728777753,
4.80875445794136));
#87309=CARTESIAN_POINT('Ctrl Pts',(11.9354020768965,-0.233755897700299,
4.80375755541058));
#87310=CARTESIAN_POINT('Ctrl Pts',(11.9294156470961,-0.155272314982306,
4.79969722121457));
#87311=CARTESIAN_POINT('Ctrl Pts',(11.9264465167955,-0.0765651061646668,
4.79563688701856));
#87312=CARTESIAN_POINT('Ctrl Pts',(11.9265007295358,0.00211765345701963,
4.79157655282255));
#87313=CARTESIAN_POINT('Ctrl Pts',(16.9092545419647,1.63408129378416,5.99751862268169));
#87314=CARTESIAN_POINT('Ctrl Pts',(17.4503910847081,1.00187072518604,5.94481637259664));
#87315=CARTESIAN_POINT('Ctrl Pts',(17.846030394839,-0.831019091968321,5.83943906626436));
#87316=CARTESIAN_POINT('Ctrl Pts',(15.854778737488,-2.84170029323275,5.68138670368482));
#87317=CARTESIAN_POINT('Ctrl Pts',(13.0882748849575,-2.26629684041423,5.52336153494307));
#87318=CARTESIAN_POINT('Ctrl Pts',(12.0566111632693,0.362281029851998,5.36533636620135));
#87319=CARTESIAN_POINT('Ctrl Pts',(13.6960010987147,2.66384541131324,5.20731119745959));
#87320=CARTESIAN_POINT('Ctrl Pts',(16.5187402906678,2.54713911068689,5.04928602871788));
#87321=CARTESIAN_POINT('Ctrl Pts',(17.963258105202,0.119422738630435,4.89126085997614));
#87322=CARTESIAN_POINT('Ctrl Pts',(16.7186900320778,-2.41690160788,4.7332356912344));
#87323=CARTESIAN_POINT('Ctrl Pts',(13.9144514535833,-2.75982500250668,4.57521052249267));
#87324=CARTESIAN_POINT('Ctrl Pts',(12.0953224532673,-0.598334453229223,
4.41718535375093));
#87325=CARTESIAN_POINT('Ctrl Pts',(12.9121191859219,2.10616193894731,4.2591601850092));
#87326=CARTESIAN_POINT('Ctrl Pts',(15.6236181183402,2.89935030149973,4.10113501626745));
#87327=CARTESIAN_POINT('Ctrl Pts',(17.7691984294259,1.061455514847,3.94310984752573));
#87328=CARTESIAN_POINT('Ctrl Pts',(17.4017970424563,-1.73968914675123,3.78508467878397));
#87329=CARTESIAN_POINT('Ctrl Pts',(14.8548219664639,-2.96210511531461,3.62705951004225));
#87330=CARTESIAN_POINT('Ctrl Pts',(12.4395925050909,-1.49648226314551,3.46903434130051));
#87331=CARTESIAN_POINT('Ctrl Pts',(12.3478719394043,1.32716321501271,3.31100917255878));
#87332=CARTESIAN_POINT('Ctrl Pts',(14.662894506894,2.94643935627629,3.15298400381705));
#87333=CARTESIAN_POINT('Ctrl Pts',(17.283832284677,1.89189200897181,2.99495883507531));
#87334=CARTESIAN_POINT('Ctrl Pts',(17.8322466004053,-0.879502394853007,
2.83693366633358));
#87335=CARTESIAN_POINT('Ctrl Pts',(15.8104644735628,-2.85276928882038,2.67890849759183));
#87336=CARTESIAN_POINT('Ctrl Pts',(13.0532051588045,-2.23721586799097,2.52088332885009));
#87337=CARTESIAN_POINT('Ctrl Pts',(12.0626157696289,0.408557624148013,2.36285816010837));
#87338=CARTESIAN_POINT('Ctrl Pts',(13.7376328649657,2.6835750260205,2.20483299136663));
#87339=CARTESIAN_POINT('Ctrl Pts',(16.5582177838479,2.52331145792478,2.04680782262489));
#87340=CARTESIAN_POINT('Ctrl Pts',(17.9647577610854,0.0732036785898677,
1.88878265388316));
#87341=CARTESIAN_POINT('Ctrl Pts',(16.6808493574509,-2.44333648707884,1.73075748514142));
#87342=CARTESIAN_POINT('Ctrl Pts',(13.8716125530259,-2.74260341607019,1.57273231639968));
#87343=CARTESIAN_POINT('Ctrl Pts',(12.0863558135253,-0.553029801627824,
1.41470714765794));
#87344=CARTESIAN_POINT('Ctrl Pts',(12.9451710463004,2.13841851363382,1.2566819789162));
#87345=CARTESIAN_POINT('Ctrl Pts',(15.6686767610793,2.88927691304951,1.09865681017448));
#87346=CARTESIAN_POINT('Ctrl Pts',(17.7854091902781,1.01823595067672,0.940631641432738));
#87347=CARTESIAN_POINT('Ctrl Pts',(17.3743807791228,-1.77692889679917,0.782606472691003));
#87348=CARTESIAN_POINT('Ctrl Pts',(14.8087915159287,-2.95937983964669,0.624581303949266));
#87349=CARTESIAN_POINT('Ctrl Pts',(12.4164593581283,-1.45664108884959,0.466556135207532));
#87350=CARTESIAN_POINT('Ctrl Pts',(12.3691365153999,1.3687011047629,0.308530966465794));
#87351=CARTESIAN_POINT('Ctrl Pts',(14.7082682063417,2.95054009376668,0.150505797724059));
#87352=CARTESIAN_POINT('Ctrl Pts',(17.3140818173384,1.85766858973412,-0.00751937101767656));
#87353=CARTESIAN_POINT('Ctrl Pts',(17.816056514554,-0.926786128220127,-0.165544539759413));
#87354=CARTESIAN_POINT('Ctrl Pts',(16.4525749211699,-2.21298286387085,-0.270894652253902));
#87355=CARTESIAN_POINT('Ctrl Pts',(15.649053482972,-2.42779823849155,-0.323569708501147));
#87356=CARTESIAN_POINT('Ctrl Pts',(17.0521313248951,1.75636581539771,6.10609621406853));
#87357=CARTESIAN_POINT('Ctrl Pts',(17.6337631743951,1.07684452411148,6.05339396398347));
#87358=CARTESIAN_POINT('Ctrl Pts',(18.0590096796851,-0.8932074130143,5.94801665765119));
#87359=CARTESIAN_POINT('Ctrl Pts',(15.9187450832242,-3.0543555400977,5.78996429507165));
#87360=CARTESIAN_POINT('Ctrl Pts',(12.945213219642,-2.43589245724096,5.63193912632992));
#87361=CARTESIAN_POINT('Ctrl Pts',(11.8363461757247,0.389391897954849,5.47391395758817));
#87362=CARTESIAN_POINT('Ctrl Pts',(13.5984178986409,2.86319110054791,5.31588878884644));
#87363=CARTESIAN_POINT('Ctrl Pts',(16.6323934060946,2.73775122332677,5.15786362010471));
#87364=CARTESIAN_POINT('Ctrl Pts',(18.1850099857178,0.128359596618317,4.99983845136296));
#87365=CARTESIAN_POINT('Ctrl Pts',(16.8473061475514,-2.59776755257373,4.84181328262124));
#87366=CARTESIAN_POINT('Ctrl Pts',(13.8332157248642,-2.96635320979502,4.68378811387949));
#87367=CARTESIAN_POINT('Ctrl Pts',(11.8779543788667,-0.643110097290728,
4.52576294513777));
#87368=CARTESIAN_POINT('Ctrl Pts',(12.7558751192975,2.26377405171339,4.36773777639603));
#87369=CARTESIAN_POINT('Ctrl Pts',(15.6702858352774,3.11631971786699,4.20971260765429));
#87370=CARTESIAN_POINT('Ctrl Pts',(17.9764280859206,1.14088827032916,4.05168743891255));
#87371=CARTESIAN_POINT('Ctrl Pts',(17.5815326550398,-1.86987670588675,3.89366227017082));
#87372=CARTESIAN_POINT('Ctrl Pts',(14.843957741748,-3.18377071320937,3.73563710142908));
#87373=CARTESIAN_POINT('Ctrl Pts',(12.2479874687677,-1.6084697256714,3.57761193268735));
#87374=CARTESIAN_POINT('Ctrl Pts',(12.1494031041135,1.42647988883321,3.41958676394561));
#87375=CARTESIAN_POINT('Ctrl Pts',(14.6376676200099,3.1669326258071,3.26156159520388));
#87376=CARTESIAN_POINT('Ctrl Pts',(17.454740145528,2.03346948748628,3.10353642646214));
#87377=CARTESIAN_POINT('Ctrl Pts',(18.0441943914605,-0.945318905954183,
2.9455112577204));
#87378=CARTESIAN_POINT('Ctrl Pts',(15.8711146142941,-3.06625287074756,2.78748608897867));
#87379=CARTESIAN_POINT('Ctrl Pts',(12.9075190924252,-2.40463524498535,2.62946092023693));
#87380=CARTESIAN_POINT('Ctrl Pts',(11.8428001296284,0.439131545904872,2.47143575149519));
#87381=CARTESIAN_POINT('Ctrl Pts',(13.6431651283877,2.8843971574036,2.31341058275346));
#87382=CARTESIAN_POINT('Ctrl Pts',(16.6748251503188,2.71214045663376,2.15538541401172));
#87383=CARTESIAN_POINT('Ctrl Pts',(18.1866218665578,0.0786817884310189,
1.99736024526999));
#87384=CARTESIAN_POINT('Ctrl Pts',(16.8066337112417,-2.62618065437941,1.83933507652825));
#87385=CARTESIAN_POINT('Ctrl Pts',(13.7871710263571,-2.94784286650975,1.68130990778652));
#87386=CARTESIAN_POINT('Ctrl Pts',(11.8683167313509,-0.594415126205828,
1.52328473904478));
#87387=CARTESIAN_POINT('Ctrl Pts',(12.791400376165,2.29844450863419,1.36525957030304));
#87388=CARTESIAN_POINT('Ctrl Pts',(15.7187163877207,3.10549249942535,1.20723440156131));
#87389=CARTESIAN_POINT('Ctrl Pts',(17.9938519596965,1.09443442170253,1.04920923281957));
#87390=CARTESIAN_POINT('Ctrl Pts',(17.5520647283902,-1.90990324814445,0.89118406407784));
#87391=CARTESIAN_POINT('Ctrl Pts',(14.794482657433,-3.18084149479233,0.733158895336105));
#87392=CARTESIAN_POINT('Ctrl Pts',(12.223123180386,-1.56564708468969,0.575133726594368));
#87393=CARTESIAN_POINT('Ctrl Pts',(12.172258989252,1.47112621694339,0.417108557852632));
#87394=CARTESIAN_POINT('Ctrl Pts',(14.6864368060542,3.17134023708901,0.259083389110896));
#87395=CARTESIAN_POINT('Ctrl Pts',(17.4872533658312,1.99668499955184,0.10105822036916));
#87396=CARTESIAN_POINT('Ctrl Pts',(18.0267927398745,-0.996141061024619,
-0.0569669483725758));
#87397=CARTESIAN_POINT('Ctrl Pts',(16.5612766302089,-2.37858879294967,-0.162317060867066));
#87398=CARTESIAN_POINT('Ctrl Pts',(15.6976246250374,-2.60947961952043,-0.214992117114311));
#87399=CARTESIAN_POINT('Ctrl Pts',(17.1950081078255,1.87865033701126,6.21467380545536));
#87400=CARTESIAN_POINT('Ctrl Pts',(17.8171352640822,1.15181832303692,6.16197155537032));
#87401=CARTESIAN_POINT('Ctrl Pts',(18.2719889645311,-0.955395734060278,
6.05659424903803));
#87402=CARTESIAN_POINT('Ctrl Pts',(15.9827114289604,-3.26701078696264,5.89854188645848));
#87403=CARTESIAN_POINT('Ctrl Pts',(12.8021515543266,-2.60548807406771,5.74051671771676));
#87404=CARTESIAN_POINT('Ctrl Pts',(11.6160811881801,0.416502766057701,5.58249154897501));
#87405=CARTESIAN_POINT('Ctrl Pts',(13.5008346985671,3.0625367897826,5.42446638023328));
#87406=CARTESIAN_POINT('Ctrl Pts',(16.7460465215216,2.92836333596666,5.26644121149155));
#87407=CARTESIAN_POINT('Ctrl Pts',(18.4067618662335,0.137296454606198,5.10841604274981));
#87408=CARTESIAN_POINT('Ctrl Pts',(16.9759222630251,-2.77863349726747,4.95039087400808));
#87409=CARTESIAN_POINT('Ctrl Pts',(13.7519799961451,-3.17288141708336,4.79236570526634));
#87410=CARTESIAN_POINT('Ctrl Pts',(11.6605863044662,-0.687885741352231,
4.63434053652461));
#87411=CARTESIAN_POINT('Ctrl Pts',(12.5996310526731,2.42138616447946,4.47631536778287));
#87412=CARTESIAN_POINT('Ctrl Pts',(15.7169535522147,3.33328913423425,4.31829019904113));
#87413=CARTESIAN_POINT('Ctrl Pts',(18.1836577424154,1.22032102581132,4.1602650302994));
#87414=CARTESIAN_POINT('Ctrl Pts',(17.7612682676234,-2.00006426502227,4.00223986155766));
#87415=CARTESIAN_POINT('Ctrl Pts',(14.8330935170321,-3.40543631110413,3.84421469281592));
#87416=CARTESIAN_POINT('Ctrl Pts',(12.0563824324444,-1.72045718819729,3.68618952407419));
#87417=CARTESIAN_POINT('Ctrl Pts',(11.9509342688227,1.52579656265371,3.52816435533245));
#87418=CARTESIAN_POINT('Ctrl Pts',(14.6124407331258,3.38742589533789,3.37013918659072));
#87419=CARTESIAN_POINT('Ctrl Pts',(17.625648006379,2.17504696600075,3.21211401784898));
#87420=CARTESIAN_POINT('Ctrl Pts',(18.2561421825157,-1.01113541705537,3.05408884910725));
#87421=CARTESIAN_POINT('Ctrl Pts',(15.9317647550255,-3.27973645267473,2.89606368036551));
#87422=CARTESIAN_POINT('Ctrl Pts',(12.761833026046,-2.57205462197974,2.73803851162378));
#87423=CARTESIAN_POINT('Ctrl Pts',(11.6229844896278,0.469705467661738,2.58001334288204));
#87424=CARTESIAN_POINT('Ctrl Pts',(13.5486973918097,3.0852192887867,2.4219881741403));
#87425=CARTESIAN_POINT('Ctrl Pts',(16.7914325167898,2.90096945534274,2.26396300539856));
#87426=CARTESIAN_POINT('Ctrl Pts',(18.40848597203,0.0841598982721637,2.10593783665683));
#87427=CARTESIAN_POINT('Ctrl Pts',(16.9324180650325,-2.80902482167996,1.94791266791509));
#87428=CARTESIAN_POINT('Ctrl Pts',(13.7027294996884,-3.15308231694932,1.78988749917336));
#87429=CARTESIAN_POINT('Ctrl Pts',(11.6502776491765,-0.635800450783829,
1.63186233043162));
#87430=CARTESIAN_POINT('Ctrl Pts',(12.6376297060296,2.45847050363454,1.47383716168988));
#87431=CARTESIAN_POINT('Ctrl Pts',(15.7687560143621,3.3217080858012,1.31581199294815));
#87432=CARTESIAN_POINT('Ctrl Pts',(18.2022947291149,1.17063289272834,1.15778682420641));
#87433=CARTESIAN_POINT('Ctrl Pts',(17.7297486776575,-2.04287759948972,0.999761655464675));
#87434=CARTESIAN_POINT('Ctrl Pts',(14.7801737989374,-3.40230314993799,0.841736486722942));
#87435=CARTESIAN_POINT('Ctrl Pts',(12.0297870026437,-1.67465308052978,0.683711317981204));
#87436=CARTESIAN_POINT('Ctrl Pts',(11.9753814631039,1.57355132912387,0.525686149239469));
#87437=CARTESIAN_POINT('Ctrl Pts',(14.6646054057666,3.39214038041133,0.367660980497734));
#87438=CARTESIAN_POINT('Ctrl Pts',(17.6604249143241,2.13570140936955,0.209635811755997));
#87439=CARTESIAN_POINT('Ctrl Pts',(18.2375289651951,-1.06549599382911,0.0516106430142612));
#87440=CARTESIAN_POINT('Ctrl Pts',(16.669978339248,-2.54419472202848,-0.0537394694802286));
#87441=CARTESIAN_POINT('Ctrl Pts',(15.7461957671028,-2.7911610005493,-0.106414525727474));
#87442=CARTESIAN_POINT('Ctrl Pts',(17.337884890756,2.00093485862481,6.3232513968422));
#87443=CARTESIAN_POINT('Ctrl Pts',(18.0005073537692,1.22679212196236,6.27054914675716));
#87444=CARTESIAN_POINT('Ctrl Pts',(18.4849682493773,-1.01758405510626,6.16517184042487));
#87445=CARTESIAN_POINT('Ctrl Pts',(16.0466777746965,-3.47966603382759,6.00711947784533));
#87446=CARTESIAN_POINT('Ctrl Pts',(12.6590898890111,-2.77508369089444,5.8490943091036));
#87447=CARTESIAN_POINT('Ctrl Pts',(11.3958162006355,0.44361363416055,5.69106914036185));
#87448=CARTESIAN_POINT('Ctrl Pts',(13.4032514984932,3.26188247901728,5.53304397162013));
#87449=CARTESIAN_POINT('Ctrl Pts',(16.8596996369486,3.11897544860654,5.37501880287838));
#87450=CARTESIAN_POINT('Ctrl Pts',(18.6285137467491,0.146233312594081,5.21699363413665));
#87451=CARTESIAN_POINT('Ctrl Pts',(17.1045383784986,-2.9594994419612,5.05896846539492));
#87452=CARTESIAN_POINT('Ctrl Pts',(13.6707442674259,-3.3794096243717,4.90094329665316));
#87453=CARTESIAN_POINT('Ctrl Pts',(11.4432182300656,-0.732661385413735,
4.74291812791145));
#87454=CARTESIAN_POINT('Ctrl Pts',(12.4433869860487,2.57899827724554,4.58489295916969));
#87455=CARTESIAN_POINT('Ctrl Pts',(15.7636212691519,3.55025855060152,4.42686779042797));
#87456=CARTESIAN_POINT('Ctrl Pts',(18.3908873989101,1.29975378129348,4.26884262168623));
#87457=CARTESIAN_POINT('Ctrl Pts',(17.9410038802068,-2.13025182415778,4.1108174529445));
#87458=CARTESIAN_POINT('Ctrl Pts',(14.8222292923162,-3.62710190899889,3.95279228420276));
#87459=CARTESIAN_POINT('Ctrl Pts',(11.8647773961211,-1.83244465072319,3.79476711546102));
#87460=CARTESIAN_POINT('Ctrl Pts',(11.7524654335319,1.6251132364742,3.63674194671928));
#87461=CARTESIAN_POINT('Ctrl Pts',(14.5872138462417,3.6079191648687,3.47871677797756));
#87462=CARTESIAN_POINT('Ctrl Pts',(17.7965558672301,2.31662444451522,3.32069160923582));
#87463=CARTESIAN_POINT('Ctrl Pts',(18.4680899735709,-1.07695192815655,3.16266644049408));
#87464=CARTESIAN_POINT('Ctrl Pts',(15.9924148957568,-3.49322003460191,3.00464127175234));
#87465=CARTESIAN_POINT('Ctrl Pts',(12.6161469596667,-2.73947399897413,2.8466161030106));
#87466=CARTESIAN_POINT('Ctrl Pts',(11.4031688496272,0.500279389418601,2.68859093426888));
#87467=CARTESIAN_POINT('Ctrl Pts',(13.4542296552316,3.28604142016981,2.53056576552714));
#87468=CARTESIAN_POINT('Ctrl Pts',(16.9080398832607,3.08979845405171,2.3725405967854));
#87469=CARTESIAN_POINT('Ctrl Pts',(18.6303500775023,0.0896380081133119,
2.21451542804366));
#87470=CARTESIAN_POINT('Ctrl Pts',(17.0582024188234,-2.99186898898052,2.05649025930192));
#87471=CARTESIAN_POINT('Ctrl Pts',(13.6182879730196,-3.35832176738888,1.89846509056019));
#87472=CARTESIAN_POINT('Ctrl Pts',(11.4322385670019,-0.677185775361829,
1.74043992181845));
#87473=CARTESIAN_POINT('Ctrl Pts',(12.4838590358943,2.61849649863489,1.58241475307672));
#87474=CARTESIAN_POINT('Ctrl Pts',(15.8187956410036,3.53792367217705,1.42438958433498));
#87475=CARTESIAN_POINT('Ctrl Pts',(18.4107374985333,1.24683136375414,1.26636441559324));
#87476=CARTESIAN_POINT('Ctrl Pts',(17.9074326269248,-2.17585195083499,1.10833924685151));
#87477=CARTESIAN_POINT('Ctrl Pts',(14.7658649404417,-3.62376480508365,0.950314078109777));
#87478=CARTESIAN_POINT('Ctrl Pts',(11.8364508249014,-1.78365907636988,0.792288909368042));
#87479=CARTESIAN_POINT('Ctrl Pts',(11.778503936956,1.67597644130436,0.634263740626305));
#87480=CARTESIAN_POINT('Ctrl Pts',(14.6427740054791,3.61294052373364,0.476238571884569));
#87481=CARTESIAN_POINT('Ctrl Pts',(17.833596462817,2.27471781918727,0.318213403142834));
#87482=CARTESIAN_POINT('Ctrl Pts',(18.4482651905155,-1.1348509266336,0.160188234401097));
#87483=CARTESIAN_POINT('Ctrl Pts',(16.7786800482871,-2.7098006511073,0.0548381219066082));
#87484=CARTESIAN_POINT('Ctrl Pts',(15.7947669091682,-2.97284238157818,0.00216306565936305));
#87485=CARTESIAN_POINT('',(16.915303916182,1.63722281354575,-0.00127815611057945));
#87486=CARTESIAN_POINT('Ctrl Pts',(15.7937992825328,-2.9692229537457,-1.0547118733939E-15));
#87487=CARTESIAN_POINT('Ctrl Pts',(15.8877631253111,-2.93485056032367,7.25862686238765E-15));
#87488=CARTESIAN_POINT('Ctrl Pts',(15.9796217175756,-2.89562062532635,1.07572107203012E-14));
#87489=CARTESIAN_POINT('Ctrl Pts',(16.0691601441602,-2.85186997887123,1.02695629777827E-14));
#87490=CARTESIAN_POINT('Ctrl Pts',(16.1600181502287,-2.80747455388162,9.77472848895889E-15));
#87491=CARTESIAN_POINT('Ctrl Pts',(16.2484877472778,-2.75842350101316,3.64929086425418E-15));
#87492=CARTESIAN_POINT('Ctrl Pts',(16.3343150074473,-2.70502273461287,-5.55111512312578E-16));
#87493=CARTESIAN_POINT('Ctrl Pts',(16.420213530084,-2.65157762949835,-4.76300480873003E-15));
#87494=CARTESIAN_POINT('Ctrl Pts',(16.5034659125644,-2.59377480350178,1.56120952333745E-14));
#87495=CARTESIAN_POINT('Ctrl Pts',(16.5837791746464,-2.53188639447444,1.50435219836709E-14));
#87496=CARTESIAN_POINT('Ctrl Pts',(16.6470097276724,-2.48316171031579,1.45958848178708E-14));
#87497=CARTESIAN_POINT('Ctrl Pts',(16.708417838421,-2.43190381471692,1.97835687267867E-15));
#87498=CARTESIAN_POINT('Ctrl Pts',(16.7678402202613,-2.37823520474345,-3.71924713249427E-15));
#87499=CARTESIAN_POINT('Ctrl Pts',(16.7818815953477,-2.36555343299908,-4.8695573782049E-15));
#87500=CARTESIAN_POINT('Ctrl Pts',(16.7958146517509,-2.35273441817498,7.35895762980806E-15));
#87501=CARTESIAN_POINT('Ctrl Pts',(16.8096179419118,-2.33979804184713,3.99680288865056E-15));
#87502=CARTESIAN_POINT('Ctrl Pts',(16.8820575556246,-2.27190798859838,-1.27952815608437E-14));
#87503=CARTESIAN_POINT('Ctrl Pts',(16.9510310384028,-2.20069650513415,2.17879392813487E-15));
#87504=CARTESIAN_POINT('Ctrl Pts',(17.0162982669385,-2.12645339766838,-5.93969318174459E-15));
#87505=CARTESIAN_POINT('Ctrl Pts',(17.0812101119845,-2.05261454782477,-1.40139747026275E-14));
#87506=CARTESIAN_POINT('Ctrl Pts',(17.1424564417789,-1.97577620343073,4.24462762398128E-15));
#87507=CARTESIAN_POINT('Ctrl Pts',(17.1997573990558,-1.89619667621841,9.35362898246694E-15));
#87508=CARTESIAN_POINT('Ctrl Pts',(17.2557584952793,-1.81842239507851,1.43467336403883E-14));
#87509=CARTESIAN_POINT('Ctrl Pts',(17.3079914815835,-1.73802914831672,-8.69766376979819E-15));
#87510=CARTESIAN_POINT('Ctrl Pts',(17.3561478113119,-1.65524376258327,-6.24500451351651E-15));
#87511=CARTESIAN_POINT('Ctrl Pts',(17.3754619924059,-1.62204081831805,-5.26131025556974E-15));
#87512=CARTESIAN_POINT('Ctrl Pts',(17.394119841153,-1.58845297300426,-6.73148743896928E-15));
#87513=CARTESIAN_POINT('Ctrl Pts',(17.4120990805709,-1.55449458909069,-8.49320613838245E-15));
#87514=CARTESIAN_POINT('Ctrl Pts',(17.4253275583043,-1.52950923153335,-8.21298736870903E-15));
#87515=CARTESIAN_POINT('Ctrl Pts',(17.4381886433291,-1.50432328064783,-9.92679727242235E-15));
#87516=CARTESIAN_POINT('Ctrl Pts',(17.4506729597229,-1.47894245110775,-5.60662627435704E-15));
#87517=CARTESIAN_POINT('Ctrl Pts',(17.4574660965599,-1.46513188730399,-3.36795545207024E-15));
#87518=CARTESIAN_POINT('Ctrl Pts',(17.4641485246816,-1.45126166531956,-9.50468321427569E-15));
#87519=CARTESIAN_POINT('Ctrl Pts',(17.4707111365409,-1.43734914681016,-1.06581410364015E-14));
#87520=CARTESIAN_POINT('Ctrl Pts',(17.5106942755179,-1.35258622420957,-1.98793348162394E-14));
#87521=CARTESIAN_POINT('Ctrl Pts',(17.5462960054721,-1.26613123171125,-1.32361921656702E-14));
#87522=CARTESIAN_POINT('Ctrl Pts',(17.5772717642454,-1.17821446018303,-2.83106871279415E-15));
#87523=CARTESIAN_POINT('Ctrl Pts',(17.6081064320176,-1.09069813938794,7.52666060535023E-15));
#87524=CARTESIAN_POINT('Ctrl Pts',(17.6343575472885,-1.00173266645316,-3.25504417137631E-15));
#87525=CARTESIAN_POINT('Ctrl Pts',(17.6557334149071,-0.911535908124523,
-8.52096171399808E-15));
#87526=CARTESIAN_POINT('Ctrl Pts',(17.6587134931134,-0.898961288999205,
-8.66732429744353E-15));
#87527=CARTESIAN_POINT('Ctrl Pts',(17.6615987301009,-0.886362732909987,
-3.82633183530923E-15));
#87528=CARTESIAN_POINT('Ctrl Pts',(17.6643882507676,-0.873740826918426,
-1.63757896132211E-15));
#87529=CARTESIAN_POINT('Ctrl Pts',(17.6849564629332,-0.780674644090523,
1.63395851942713E-14));
#87530=CARTESIAN_POINT('Ctrl Pts',(17.7003250436256,-0.686338012910902,
-1.92404708757836E-14));
#87531=CARTESIAN_POINT('Ctrl Pts',(17.7105713114964,-0.591140293501985,
-1.74582570622306E-14));
#87532=CARTESIAN_POINT('Ctrl Pts',(17.7164074023686,-0.536917375625885,
-1.64431399580609E-14));
#87533=CARTESIAN_POINT('Ctrl Pts',(17.7205807502074,-0.482415289412221,
-1.20770545210332E-14));
#87534=CARTESIAN_POINT('Ctrl Pts',(17.7230986015199,-0.427712441435951,
-2.27318164292001E-14));
#87535=CARTESIAN_POINT('Ctrl Pts',(17.7236733846671,-0.415224700415009,
-2.47925753357554E-14));
#87536=CARTESIAN_POINT('Ctrl Pts',(17.7241617587452,-0.402728082302084,
5.67804429951126E-15));
#87537=CARTESIAN_POINT('Ctrl Pts',(17.7245636675657,-0.390232963134124,
7.04991620636974E-15));
#87538=CARTESIAN_POINT('Ctrl Pts',(17.7275525323397,-0.297310838444643,
1.56178684923478E-14));
#87539=CARTESIAN_POINT('Ctrl Pts',(17.7257709900994,-0.204325895882787,
1.14009966214644E-14));
#87540=CARTESIAN_POINT('Ctrl Pts',(17.7193534316054,-0.111650468563709,
-3.89965837399586E-15));
#87541=CARTESIAN_POINT('Ctrl Pts',(17.7129132516647,-0.018648366819267,
-1.92542471124444E-14));
#87542=CARTESIAN_POINT('Ctrl Pts',(17.701803954752,0.074043009764724,-1.90773904346453E-14));
#87543=CARTESIAN_POINT('Ctrl Pts',(17.6861107070086,0.166035470154942,-1.06165076729781E-14));
#87544=CARTESIAN_POINT('Ctrl Pts',(17.6705478903124,0.257263355032181,-2.22594571532359E-15));
#87545=CARTESIAN_POINT('Ctrl Pts',(17.6504765789002,0.347804777454888,-9.29780401233961E-15));
#87546=CARTESIAN_POINT('Ctrl Pts',(17.6259361013488,0.437255629196133,-1.19626530903361E-14));
#87547=CARTESIAN_POINT('Ctrl Pts',(17.6168824130534,0.470256622258459,-1.24188389511132E-14));
#87548=CARTESIAN_POINT('Ctrl Pts',(17.607220033895,0.503108861729303,-1.77227151771264E-14));
#87549=CARTESIAN_POINT('Ctrl Pts',(17.5969495907262,0.535790803903075,-1.23789867245705E-14));
#87550=CARTESIAN_POINT('Ctrl Pts',(17.5906923635436,0.555702148875279,-9.16506532922899E-15));
#87551=CARTESIAN_POINT('Ctrl Pts',(17.5842094210688,0.575550268330647,2.38196241363701E-15));
#87552=CARTESIAN_POINT('Ctrl Pts',(17.5775007819672,0.595330144314736,-1.24206200879939E-14));
#87553=CARTESIAN_POINT('Ctrl Pts',(17.5720344395212,0.611447209792455,-2.43995415110235E-14));
#87554=CARTESIAN_POINT('Ctrl Pts',(17.5664177473268,0.627520100869461,3.28653594930177E-15));
#87555=CARTESIAN_POINT('Ctrl Pts',(17.5606568980948,0.643529501722759,2.28983498828939E-15));
#87556=CARTESIAN_POINT('Ctrl Pts',(17.5300998777373,0.72844746573855,1.8961345380147E-15));
#87557=CARTESIAN_POINT('Ctrl Pts',(17.4954544625937,0.81169001210649,8.70397767353563E-15));
#87558=CARTESIAN_POINT('Ctrl Pts',(17.4567798259733,0.892884379764742,7.42461647718073E-15));
#87559=CARTESIAN_POINT('Ctrl Pts',(17.4252161779729,0.959149784286503,6.38048755973252E-15));
#87560=CARTESIAN_POINT('Ctrl Pts',(17.3909678991583,1.02405068948786,8.96555908749261E-15));
#87561=CARTESIAN_POINT('Ctrl Pts',(17.3540486134849,1.08736649490362,-1.60982338570648E-15));
#87562=CARTESIAN_POINT('Ctrl Pts',(17.3403704993332,1.11082417557878,-5.21161029651093E-15));
#87563=CARTESIAN_POINT('Ctrl Pts',(17.3263256078231,1.13406409955685,1.28764437023275E-14));
#87564=CARTESIAN_POINT('Ctrl Pts',(17.3119141100336,1.15707434952577,-6.28663787693995E-15));
#87565=CARTESIAN_POINT('Ctrl Pts',(17.3022209349234,1.17255104636444,-1.95408450057356E-14));
#87566=CARTESIAN_POINT('Ctrl Pts',(17.2923614563489,1.18792433165914,9.0007685035821E-15));
#87567=CARTESIAN_POINT('Ctrl Pts',(17.2823446805049,1.20317728665099,9.74220704108575E-15));
#87568=CARTESIAN_POINT('Ctrl Pts',(17.2351636329007,1.27502180097183,8.69901979580413E-15));
#87569=CARTESIAN_POINT('Ctrl Pts',(17.1844507000559,1.34427231397538,8.43316798846986E-15));
#87570=CARTESIAN_POINT('Ctrl Pts',(17.1302392162511,1.41057629209039,7.63278329429795E-15));
#87571=CARTESIAN_POINT('Ctrl Pts',(17.0809261548577,1.47088919839622,9.33123635964826E-15));
#87572=CARTESIAN_POINT('Ctrl Pts',(17.0287176381672,1.52876397615804,-5.08825234704773E-15));
#87573=CARTESIAN_POINT('Ctrl Pts',(16.9736175325606,1.58390431335901,8.71091393461754E-15));
#87574=CARTESIAN_POINT('Ctrl Pts',(16.955089701729,1.60244567237107,1.28632355881959E-14));
#87575=CARTESIAN_POINT('Ctrl Pts',(16.9362347568812,1.62067756637814,-1.19777121980603E-15));
#87576=CARTESIAN_POINT('Ctrl Pts',(16.9170623502469,1.63859592449701,9.04051139505313E-15));
#87577=CARTESIAN_POINT('Ctrl Pts',(16.9134659966651,1.63598720337494,6.));
#87578=CARTESIAN_POINT('Ctrl Pts',(16.9755094815351,1.5776815625216,5.99999999999999));
#87579=CARTESIAN_POINT('Ctrl Pts',(17.034139121574,1.51618400144596,5.99999999999998));
#87580=CARTESIAN_POINT('Ctrl Pts',(17.0893566813826,1.45188668377136,5.99999999999998));
#87581=CARTESIAN_POINT('Ctrl Pts',(17.1457272627278,1.38624674624397,5.99999999999998));
#87582=CARTESIAN_POINT('Ctrl Pts',(17.1985421988915,1.31768842238335,6.));
#87583=CARTESIAN_POINT('Ctrl Pts',(17.2477776475324,1.24658007436298,6.00000000000001));
#87584=CARTESIAN_POINT('Ctrl Pts',(17.2982360478219,1.17370547714931,6.00000000000001));
#87585=CARTESIAN_POINT('Ctrl Pts',(17.3449354505362,1.09815203002923,6.00000000000002));
#87586=CARTESIAN_POINT('Ctrl Pts',(17.3878162017473,1.02027348726958,6.));
#87587=CARTESIAN_POINT('Ctrl Pts',(17.4063927730161,0.98653535864483,5.99999999999999));
#87588=CARTESIAN_POINT('Ctrl Pts',(17.4242522071428,0.952360385941308,5.99999999999999));
#87589=CARTESIAN_POINT('Ctrl Pts',(17.4413873608898,0.917775372037375,6.));
#87590=CARTESIAN_POINT('Ctrl Pts',(17.4513051088949,0.897757725407784,6.00000000000001));
#87591=CARTESIAN_POINT('Ctrl Pts',(17.4609801930981,0.877602693578679,5.99999999999999));
#87592=CARTESIAN_POINT('Ctrl Pts',(17.4704109979228,0.8573153278544,6.));
#87593=CARTESIAN_POINT('Ctrl Pts',(17.4789439761822,0.838959349347455,6.00000000000001));
#87594=CARTESIAN_POINT('Ctrl Pts',(17.4872793672599,0.820489262936239,6.00000000000001));
#87595=CARTESIAN_POINT('Ctrl Pts',(17.4954022352014,0.801940725847788,6.00000000000001));
#87596=CARTESIAN_POINT('Ctrl Pts',(17.532082498778,0.718181487821601,5.99999999999999));
#87597=CARTESIAN_POINT('Ctrl Pts',(17.564479455655,0.632730199218269,5.99999999999999));
#87598=CARTESIAN_POINT('Ctrl Pts',(17.5925671692333,0.545988213295408,5.99999999999999));
#87599=CARTESIAN_POINT('Ctrl Pts',(17.6210371396809,0.458065721174328,6.));
#87600=CARTESIAN_POINT('Ctrl Pts',(17.6450802539788,0.368816386817013,5.99999999999999));
#87601=CARTESIAN_POINT('Ctrl Pts',(17.6646303946722,0.278621061222165,5.99999999999998));
#87602=CARTESIAN_POINT('Ctrl Pts',(17.6842040041827,0.18831746133696,5.99999999999998));
#87603=CARTESIAN_POINT('Ctrl Pts',(17.6992742681111,0.0970647054962511,
6.));
#87604=CARTESIAN_POINT('Ctrl Pts',(17.7097292318061,0.00522075650062019,
6.));
#87605=CARTESIAN_POINT('Ctrl Pts',(17.7136173613966,-0.0289353808343625,
6.));
#87606=CARTESIAN_POINT('Ctrl Pts',(17.7168666892977,-0.0631734552839064,
6.));
#87607=CARTESIAN_POINT('Ctrl Pts',(17.7194696669028,-0.09747552158852,5.99999999999999));
#87608=CARTESIAN_POINT('Ctrl Pts',(17.7212325560646,-0.120706893535899,
5.99999999999999));
#87609=CARTESIAN_POINT('Ctrl Pts',(17.722698957133,-0.143967621373419,5.99999999999999));
#87610=CARTESIAN_POINT('Ctrl Pts',(17.7238662552278,-0.167252159912536,
6.));
#87611=CARTESIAN_POINT('Ctrl Pts',(17.7245262789947,-0.180417904726593,
6.));
#87612=CARTESIAN_POINT('Ctrl Pts',(17.7250904489575,-0.193587605540001,
5.99999999999998));
#87613=CARTESIAN_POINT('Ctrl Pts',(17.7255582477108,-0.206751979691985,
5.99999999999998));
#87614=CARTESIAN_POINT('Ctrl Pts',(17.7290248924967,-0.304307196955097,
6.00000000000001));
#87615=CARTESIAN_POINT('Ctrl Pts',(17.7272102314639,-0.401701395411429,
6.));
#87616=CARTESIAN_POINT('Ctrl Pts',(17.7200480989972,-0.4985064694598,6.));
#87617=CARTESIAN_POINT('Ctrl Pts',(17.7128859665305,-0.595311543508181,
6.));
#87618=CARTESIAN_POINT('Ctrl Pts',(17.7003768098819,-0.691528572964534,
6.00000000000001));
#87619=CARTESIAN_POINT('Ctrl Pts',(17.6824005104444,-0.786748819384737,
6.00000000000001));
#87620=CARTESIAN_POINT('Ctrl Pts',(17.665301687038,-0.877321085601708,6.00000000000001));
#87621=CARTESIAN_POINT('Ctrl Pts',(17.6432564988628,-0.966992484953733,
5.99999999999999));
#87622=CARTESIAN_POINT('Ctrl Pts',(17.6165400759011,-1.05552334469227,6.));
#87623=CARTESIAN_POINT('Ctrl Pts',(17.6012165843948,-1.10630117072041,6.));
#87624=CARTESIAN_POINT('Ctrl Pts',(17.5843553947488,-1.15670375619126,6.00000000000001));
#87625=CARTESIAN_POINT('Ctrl Pts',(17.5660009192215,-1.20668470741449,5.99999999999999));
#87626=CARTESIAN_POINT('Ctrl Pts',(17.5600040426582,-1.22301476242238,5.99999999999998));
#87627=CARTESIAN_POINT('Ctrl Pts',(17.5538468430946,-1.23930175643138,6.00000000000002));
#87628=CARTESIAN_POINT('Ctrl Pts',(17.5475394190055,-1.25552261396836,6.00000000000002));
#87629=CARTESIAN_POINT('Ctrl Pts',(17.5132439135909,-1.34372066433486,6.00000000000001));
#87630=CARTESIAN_POINT('Ctrl Pts',(17.4744620559964,-1.43010229333925,6.00000000000001));
#87631=CARTESIAN_POINT('Ctrl Pts',(17.4315373968039,-1.51442487125201,6.));
#87632=CARTESIAN_POINT('Ctrl Pts',(17.3877735627611,-1.60039595116852,5.99999999999999));
#87633=CARTESIAN_POINT('Ctrl Pts',(17.3397030795252,-1.68422740148093,5.99999999999998));
#87634=CARTESIAN_POINT('Ctrl Pts',(17.2876347517893,-1.76565902892484,5.99999999999998));
#87635=CARTESIAN_POINT('Ctrl Pts',(17.2346998347258,-1.84844594820065,5.99999999999999));
#87636=CARTESIAN_POINT('Ctrl Pts',(17.1776325286954,-1.92875332663683,6.));
#87637=CARTESIAN_POINT('Ctrl Pts',(17.1167056749116,-2.006292820283,5.99999999999999));
#87638=CARTESIAN_POINT('Ctrl Pts',(17.0750631441813,-2.05928982482935,5.99999999999998));
#87639=CARTESIAN_POINT('Ctrl Pts',(17.0316165436599,-2.1109935011868,5.99999999999999));
#87640=CARTESIAN_POINT('Ctrl Pts',(16.9864408800736,-2.1613047605532,6.00000000000001));
#87641=CARTESIAN_POINT('Ctrl Pts',(16.9750475422705,-2.17399329964164,6.00000000000001));
#87642=CARTESIAN_POINT('Ctrl Pts',(16.9635434048419,-2.18659396301802,5.99999999999998));
#87643=CARTESIAN_POINT('Ctrl Pts',(16.9519414333288,-2.19909266058292,5.99999999999998));
#87644=CARTESIAN_POINT('Ctrl Pts',(16.8830336246512,-2.27332641124779,6.));
#87645=CARTESIAN_POINT('Ctrl Pts',(16.8105865574123,-2.34406896254778,5.99999999999998));
#87646=CARTESIAN_POINT('Ctrl Pts',(16.7349147382584,-2.4110269921092,5.99999999999999));
#87647=CARTESIAN_POINT('Ctrl Pts',(16.6721145810702,-2.46659556213289,6.));
#87648=CARTESIAN_POINT('Ctrl Pts',(16.6070923153041,-2.51955756893482,6.00000000000001));
#87649=CARTESIAN_POINT('Ctrl Pts',(16.5400041594286,-2.56973166063313,6.00000000000001));
#87650=CARTESIAN_POINT('Ctrl Pts',(16.5180622947882,-2.58614160832257,6.00000000000001));
#87651=CARTESIAN_POINT('Ctrl Pts',(16.4958992912228,-2.60225321472728,6.00000000000001));
#87652=CARTESIAN_POINT('Ctrl Pts',(16.4735201854318,-2.61805974701069,6.00000000000001));
#87653=CARTESIAN_POINT('Ctrl Pts',(16.4507974239471,-2.63410900591904,6.00000000000001));
#87654=CARTESIAN_POINT('Ctrl Pts',(16.4278464912961,-2.6498471559999,6.));
#87655=CARTESIAN_POINT('Ctrl Pts',(16.4047016736817,-2.66524800157915,6.));
#87656=CARTESIAN_POINT('Ctrl Pts',(16.3197414959508,-2.72178154612555,6.));
#87657=CARTESIAN_POINT('Ctrl Pts',(16.2321168885192,-2.77381412681324,6.));
#87658=CARTESIAN_POINT('Ctrl Pts',(16.1421188622891,-2.82103724255303,6.));
#87659=CARTESIAN_POINT('Ctrl Pts',(16.058344827335,-2.86499455044454,6.00000000000001));
#87660=CARTESIAN_POINT('Ctrl Pts',(15.9725134939175,-2.90478489918908,6.00000000000001));
#87661=CARTESIAN_POINT('Ctrl Pts',(15.8848316115121,-2.94013000968632,6.00000000000001));
#87662=CARTESIAN_POINT('Ctrl Pts',(15.8554933457997,-2.9519564465163,6.00000000000001));
#87663=CARTESIAN_POINT('Ctrl Pts',(15.8259477042398,-2.96328493422549,6.00000000000001));
#87664=CARTESIAN_POINT('Ctrl Pts',(15.7962062164482,-2.97411882975737,6.00000000000001));
#87665=CARTESIAN_POINT('Ctrl Pts',(16.9136316953219,1.63579338079708,-0.00127815611057958));
#87666=CARTESIAN_POINT('Ctrl Pts',(16.9051833118704,1.64567671602558,-0.000852104073719735));
#87667=CARTESIAN_POINT('Ctrl Pts',(16.8966583601906,1.65549459987556,-0.000426052036859841));
#87668=CARTESIAN_POINT('Ctrl Pts',(16.8880578635265,1.66524585391345,0.));
#87669=CARTESIAN_POINT('Ctrl Pts',(14.2051896689321,-2.97300480210898,5.99773986754201));
#87670=CARTESIAN_POINT('Ctrl Pts',(13.2212227739548,-2.70994870041619,5.94506481129476));
#87671=CARTESIAN_POINT('Ctrl Pts',(11.5515433528338,-1.13493172195381,5.83971469880028));
#87672=CARTESIAN_POINT('Ctrl Pts',(12.1662514122567,2.27485164275103,5.68168953005853));
#87673=CARTESIAN_POINT('Ctrl Pts',(15.3572450886927,3.61313057072747,5.52366436131681));
#87674=CARTESIAN_POINT('Ctrl Pts',(18.2216707218686,1.67607095050132,5.36563919257506));
#87675=CARTESIAN_POINT('Ctrl Pts',(18.16372112867,-1.78375794773966,5.20761402383333));
#87676=CARTESIAN_POINT('Ctrl Pts',(15.234147542334,-3.62396028172564,5.0495888550916));
#87677=CARTESIAN_POINT('Ctrl Pts',(12.0924097431305,-2.17597071420578,4.89156368634986));
#87678=CARTESIAN_POINT('Ctrl Pts',(11.5890772899766,1.24689941213705,4.73353851760813));
#87679=CARTESIAN_POINT('Ctrl Pts',(14.1811599880455,3.53811546760277,4.57551334886638));
#87680=CARTESIAN_POINT('Ctrl Pts',(17.5162774785844,2.61863872630337,4.41748818012465));
#87681=CARTESIAN_POINT('Ctrl Pts',(18.5679550843236,-0.677222592335036,
4.25946301138291));
#87682=CARTESIAN_POINT('Ctrl Pts',(16.3817870007077,-3.35850399264624,4.10143784264118));
#87683=CARTESIAN_POINT('Ctrl Pts',(12.9416858874442,-2.99203138157406,3.94341267389944));
#87684=CARTESIAN_POINT('Ctrl Pts',(11.3694528936595,0.0896428835206473,
3.78538750515772));
#87685=CARTESIAN_POINT('Ctrl Pts',(13.0918565671579,3.08996613614193,3.62736233641597));
#87686=CARTESIAN_POINT('Ctrl Pts',(16.5458542345706,3.28621976149866,3.46933716767424));
#87687=CARTESIAN_POINT('Ctrl Pts',(18.5970263563853,0.500306538668845,3.3113119989325));
#87688=CARTESIAN_POINT('Ctrl Pts',(17.38398241508,-2.73962267337911,3.15328683019077));
#87689=CARTESIAN_POINT('Ctrl Pts',(14.0075312446594,-3.49340961705167,2.99526166144903));
#87690=CARTESIAN_POINT('Ctrl Pts',(11.5317218080708,-1.07701037592612,2.83723649270729));
#87691=CARTESIAN_POINT('Ctrl Pts',(12.2032923596136,2.31675017147752,2.67921132396556));
#87692=CARTESIAN_POINT('Ctrl Pts',(15.4128085563852,3.60811497096177,2.52118615522382));
#87693=CARTESIAN_POINT('Ctrl Pts',(18.2477108145854,1.62520143551189,2.36316098648209));
#87694=CARTESIAN_POINT('Ctrl Pts',(18.1353927575591,-1.8325441034938,2.20513581774035));
#87695=CARTESIAN_POINT('Ctrl Pts',(15.1777803543678,-3.62729875091689,2.04711064899861));
#87696=CARTESIAN_POINT('Ctrl Pts',(12.0588365095769,-2.13036744730225,1.88908548025688));
#87697=CARTESIAN_POINT('Ctrl Pts',(11.6089285681624,1.29982434138019,1.73106031151514));
#87698=CARTESIAN_POINT('Ctrl Pts',(14.2363372968936,3.55045119102204,1.57303514277341));
#87699=CARTESIAN_POINT('Ctrl Pts',(17.5567517477241,2.57913831033334,1.41500997403167));
#87700=CARTESIAN_POINT('Ctrl Pts',(18.5569748354369,-0.732701268045499,
1.25698480528994));
#87701=CARTESIAN_POINT('Ctrl Pts',(16.3293278072767,-3.3795928169039,1.0989596365482));
#87702=CARTESIAN_POINT('Ctrl Pts',(12.8953475337801,-2.95966043224143,0.940934467806465));
#87703=CARTESIAN_POINT('Ctrl Pts',(11.3712890776038,0.146241897576049,0.782909299064727));
#87704=CARTESIAN_POINT('Ctrl Pts',(13.1401999240478,3.11914361205027,0.624884130322993));
#87705=CARTESIAN_POINT('Ctrl Pts',(16.5968342039323,3.26206136074565,0.466858961581257));
#87706=CARTESIAN_POINT('Ctrl Pts',(18.6043812699741,0.443634682954898,0.30883379283952));
#87707=CARTESIAN_POINT('Ctrl Pts',(17.3410334970383,-2.77522949326083,0.150808624097785));
#87708=CARTESIAN_POINT('Ctrl Pts',(13.9532726620765,-3.47986248795946,-0.00721654464395101));
#87709=CARTESIAN_POINT('Ctrl Pts',(11.5152477272064,-1.01804953619222,-0.165241713385687));
#87710=CARTESIAN_POINT('Ctrl Pts',(11.9990787995815,1.22570074963817,-0.270591825880177));
#87711=CARTESIAN_POINT('Ctrl Pts',(12.660961939353,1.99984548567625,-0.323266882127422));
#87712=CARTESIAN_POINT('Ctrl Pts',(14.2536953592163,-2.79156824484793,6.10617114577956));
#87713=CARTESIAN_POINT('Ctrl Pts',(13.3297780025906,-2.54456593271639,6.05349608953231));
#87714=CARTESIAN_POINT('Ctrl Pts',(11.7619957885252,-1.06566910111593,5.94814597703782));
#87715=CARTESIAN_POINT('Ctrl Pts',(12.3391894403214,2.13602198124237,5.79012080829609));
#87716=CARTESIAN_POINT('Ctrl Pts',(15.3354431329929,3.3926284137103,5.63209563955435));
#87717=CARTESIAN_POINT('Ctrl Pts',(18.0250585791671,1.57378368114728,5.47407047081262));
#87718=CARTESIAN_POINT('Ctrl Pts',(17.9706455341359,-1.67489875558656,5.31604530207088));
#87719=CARTESIAN_POINT('Ctrl Pts',(15.2198579845297,-3.40279720903209,5.15802013332914));
#87720=CARTESIAN_POINT('Ctrl Pts',(12.2698541810803,-2.04317555867616,4.99999496458742));
#87721=CARTESIAN_POINT('Ctrl Pts',(11.7972391042971,1.17080362634199,4.84196979584567));
#87722=CARTESIAN_POINT('Ctrl Pts',(14.2311321618581,3.32219133280872,4.68394462710394));
#87723=CARTESIAN_POINT('Ctrl Pts',(17.3627140795262,2.45882842432408,4.5259194583622));
#87724=CARTESIAN_POINT('Ctrl Pts',(18.3502098971975,-0.635893047369115,
4.36789428962046));
#87725=CARTESIAN_POINT('Ctrl Pts',(16.297459294241,-3.15354118816609,4.20986912087873));
#87726=CARTESIAN_POINT('Ctrl Pts',(13.0673006950891,-2.80943367009216,4.05184395213699));
#87727=CARTESIAN_POINT('Ctrl Pts',(11.5910179471305,0.0841721570161353,
3.89381878339526));
#87728=CARTESIAN_POINT('Ctrl Pts',(13.2083067575408,2.90139166179291,3.73579361465352));
#87729=CARTESIAN_POINT('Ctrl Pts',(16.451513831841,3.08566831956807,3.57776844591179));
#87730=CARTESIAN_POINT('Ctrl Pts',(18.3775070074704,0.469773827827989,3.41974327717005));
#87731=CARTESIAN_POINT('Ctrl Pts',(17.2384927200562,-2.57242896225573,3.26171810842832));
#87732=CARTESIAN_POINT('Ctrl Pts',(14.0680996346029,-3.28021379120878,3.10369293968658));
#87733=CARTESIAN_POINT('Ctrl Pts',(11.7433839131305,-1.01128257938712,2.94566777094485));
#87734=CARTESIAN_POINT('Ctrl Pts',(12.3739698524913,2.17536352627309,2.78764260220311));
#87735=CARTESIAN_POINT('Ctrl Pts',(15.3876156730016,3.38791890600118,2.62961743346137));
#87736=CARTESIAN_POINT('Ctrl Pts',(18.0495094969287,1.52601863126421,2.47159226471964));
#87737=CARTESIAN_POINT('Ctrl Pts',(17.9440459870497,-1.72070758949588,2.3135670959779));
#87738=CARTESIAN_POINT('Ctrl Pts',(15.1669307736936,-3.40593193810287,2.15554192723617));
#87739=CARTESIAN_POINT('Ctrl Pts',(12.2383298550521,-2.00035536825505,1.99751675849443));
#87740=CARTESIAN_POINT('Ctrl Pts',(11.8158788985427,1.22049865264372,1.83949158975269));
#87741=CARTESIAN_POINT('Ctrl Pts',(14.282942109527,3.33377423161536,1.68146642101096));
#87742=CARTESIAN_POINT('Ctrl Pts',(17.400718284694,2.42173864000821,1.52344125226922));
#87743=CARTESIAN_POINT('Ctrl Pts',(18.3398997510145,-0.687985970081409,
1.36541608352749));
#87744=CARTESIAN_POINT('Ctrl Pts',(16.248201580823,-3.17334300351367,1.20739091478575));
#87745=CARTESIAN_POINT('Ctrl Pts',(13.0237902787871,-2.77903825527531,1.04936574604401));
#87746=CARTESIAN_POINT('Ctrl Pts',(11.5927420724286,0.137317046057244,0.891340577302276));
#87747=CARTESIAN_POINT('Ctrl Pts',(13.253699815718,2.92878849450329,0.733315408560539));
#87748=CARTESIAN_POINT('Ctrl Pts',(16.4993825952861,3.06298425786033,0.575290239818805));
#87749=CARTESIAN_POINT('Ctrl Pts',(18.3844130653427,0.416560542509571,0.417265071077067));
#87750=CARTESIAN_POINT('Ctrl Pts',(17.1981648888767,-2.60586276889182,0.259239902335333));
#87751=CARTESIAN_POINT('Ctrl Pts',(14.0171523451665,-3.26749341640285,0.101214733593596));
#87752=CARTESIAN_POINT('Ctrl Pts',(11.7279152125851,-0.955920002181071,
-0.056810435148139));
#87753=CARTESIAN_POINT('Ctrl Pts',(12.1822190389883,1.15089867596211,-0.16216054764263));
#87754=CARTESIAN_POINT('Ctrl Pts',(12.803708770009,1.87779890178989,-0.214835603889875));
#87755=CARTESIAN_POINT('Ctrl Pts',(14.3022010495005,-2.61013168758689,6.2146024240171));
#87756=CARTESIAN_POINT('Ctrl Pts',(13.4383332312262,-2.3791831650166,6.16192736776986));
#87757=CARTESIAN_POINT('Ctrl Pts',(11.9724482242165,-0.996406480278056,
6.05657725527536));
#87758=CARTESIAN_POINT('Ctrl Pts',(12.512127468386,1.99719231973372,5.89855208653363));
#87759=CARTESIAN_POINT('Ctrl Pts',(15.3136411772931,3.17212625669313,5.74052691779189));
#87760=CARTESIAN_POINT('Ctrl Pts',(17.8284464364657,1.47149641179321,5.58250174905016));
#87761=CARTESIAN_POINT('Ctrl Pts',(17.7775699396018,-1.56603956343343,5.42447658030842));
#87762=CARTESIAN_POINT('Ctrl Pts',(15.2055684267254,-3.18163413633856,5.26645141156668));
#87763=CARTESIAN_POINT('Ctrl Pts',(12.44729861903,-1.91038040314654,5.10842624282495));
#87764=CARTESIAN_POINT('Ctrl Pts',(12.0054009186174,1.09470784054693,4.95040107408321));
#87765=CARTESIAN_POINT('Ctrl Pts',(14.2811043356706,3.10626719801468,4.79237590534148));
#87766=CARTESIAN_POINT('Ctrl Pts',(17.2091506804682,2.29901812234478,4.63435073659974));
#87767=CARTESIAN_POINT('Ctrl Pts',(18.1324647100716,-0.594563502403188,
4.47632556785801));
#87768=CARTESIAN_POINT('Ctrl Pts',(16.2131315877742,-2.94857838368594,4.31830039911627));
#87769=CARTESIAN_POINT('Ctrl Pts',(13.1929155027339,-2.62683595861024,4.16027523037453));
#87770=CARTESIAN_POINT('Ctrl Pts',(11.8125830006014,0.0787014305116236,
4.0022500616328));
#87771=CARTESIAN_POINT('Ctrl Pts',(13.3247569479238,2.71281718744388,3.84422489289106));
#87772=CARTESIAN_POINT('Ctrl Pts',(16.3571734291114,2.88511687763747,3.68619972414933));
#87773=CARTESIAN_POINT('Ctrl Pts',(18.1579876585555,0.439241116987135,3.52817455540759));
#87774=CARTESIAN_POINT('Ctrl Pts',(17.0930030250325,-2.40523525113236,3.37014938666586));
#87775=CARTESIAN_POINT('Ctrl Pts',(14.1286680245464,-3.0670179653659,3.21212421792412));
#87776=CARTESIAN_POINT('Ctrl Pts',(11.9550460181903,-0.945554782848137,
3.05409904918239));
#87777=CARTESIAN_POINT('Ctrl Pts',(12.5446473453691,2.03397688106867,2.89607388044065));
#87778=CARTESIAN_POINT('Ctrl Pts',(15.3624227896179,3.16772284104057,2.73804871169891));
#87779=CARTESIAN_POINT('Ctrl Pts',(17.851308179272,1.42683582701653,2.58002354295718));
#87780=CARTESIAN_POINT('Ctrl Pts',(17.7526992165401,-1.60887107549796,2.42199837421544));
#87781=CARTESIAN_POINT('Ctrl Pts',(15.1560811930195,-3.18456512528884,2.26397320547371));
#87782=CARTESIAN_POINT('Ctrl Pts',(12.4178232005272,-1.87034328920784,2.10594803673197));
#87783=CARTESIAN_POINT('Ctrl Pts',(12.0228292289231,1.14117296390725,1.94792286799024));
#87784=CARTESIAN_POINT('Ctrl Pts',(14.3295469221603,3.11709727220868,1.7898976992485));
#87785=CARTESIAN_POINT('Ctrl Pts',(17.2446848216638,2.2643389696831,1.63187253050676));
#87786=CARTESIAN_POINT('Ctrl Pts',(18.1228246665922,-0.643270672117315,
1.47384736176503));
#87787=CARTESIAN_POINT('Ctrl Pts',(16.1670753543694,-2.96709319012346,1.31582219302329));
#87788=CARTESIAN_POINT('Ctrl Pts',(13.1522330237942,-2.5984160783092,1.15779702428156));
#87789=CARTESIAN_POINT('Ctrl Pts',(11.8141950672532,0.128392194538437,0.999771855539822));
#87790=CARTESIAN_POINT('Ctrl Pts',(13.3671997073883,2.73843337695631,0.841746686798087));
#87791=CARTESIAN_POINT('Ctrl Pts',(16.4019309866401,2.86390715497503,0.683721518056352));
#87792=CARTESIAN_POINT('Ctrl Pts',(18.1644448607113,0.389486402064242,0.525696349314615));
#87793=CARTESIAN_POINT('Ctrl Pts',(17.0552962807149,-2.43649604452279,0.367671180572879));
#87794=CARTESIAN_POINT('Ctrl Pts',(14.0810320282566,-3.05512434484625,0.209646011831144));
#87795=CARTESIAN_POINT('Ctrl Pts',(11.9405826979638,-0.893790468169929,
0.051620843089408));
#87796=CARTESIAN_POINT('Ctrl Pts',(12.365359278395,1.07609660228605,-0.0537292694050819));
#87797=CARTESIAN_POINT('Ctrl Pts',(12.9464556006651,1.75575231790353,-0.106404325652328));
#87798=CARTESIAN_POINT('Ctrl Pts',(14.3507067397847,-2.42869513032583,6.32303370225465));
#87799=CARTESIAN_POINT('Ctrl Pts',(13.5468884598619,-2.2138003973168,6.27035864600741));
#87800=CARTESIAN_POINT('Ctrl Pts',(12.1829006599078,-0.927143859440181,
6.16500853351291));
#87801=CARTESIAN_POINT('Ctrl Pts',(12.6850654964508,1.85836265822507,6.00698336477119));
#87802=CARTESIAN_POINT('Ctrl Pts',(15.2918392215932,2.95162409967596,5.84895819602944));
#87803=CARTESIAN_POINT('Ctrl Pts',(17.6318342937641,1.36920914243917,5.69093302728772));
#87804=CARTESIAN_POINT('Ctrl Pts',(17.5844943450677,-1.45718037128031,5.53290785854596));
#87805=CARTESIAN_POINT('Ctrl Pts',(15.1912788689212,-2.96047106364502,5.37488268980425));
#87806=CARTESIAN_POINT('Ctrl Pts',(12.6247430569797,-1.77758524761693,5.21685752106249));
#87807=CARTESIAN_POINT('Ctrl Pts',(12.2135627329378,1.01861205475188,5.05883235232077));
#87808=CARTESIAN_POINT('Ctrl Pts',(14.3310765094832,2.89034306322065,4.90080718357903));
#87809=CARTESIAN_POINT('Ctrl Pts',(17.0555872814102,2.13920782036547,4.7427820148373));
#87810=CARTESIAN_POINT('Ctrl Pts',(17.9147195229455,-0.553233957437266,
4.58475684609556));
#87811=CARTESIAN_POINT('Ctrl Pts',(16.1288038813074,-2.74361557920579,4.42673167735383));
#87812=CARTESIAN_POINT('Ctrl Pts',(13.3185303103786,-2.44423824712834,4.26870650861208));
#87813=CARTESIAN_POINT('Ctrl Pts',(12.0341480540722,0.0732307040071116,
4.11068133987036));
#87814=CARTESIAN_POINT('Ctrl Pts',(13.4412071383069,2.52424271309487,3.95265617112861));
#87815=CARTESIAN_POINT('Ctrl Pts',(16.2628330263819,2.68456543570688,3.79463100238688));
#87816=CARTESIAN_POINT('Ctrl Pts',(17.9384683096406,0.40870840614628,3.63660583364514));
#87817=CARTESIAN_POINT('Ctrl Pts',(16.9475133300087,-2.23804154000899,3.4785806649034));
#87818=CARTESIAN_POINT('Ctrl Pts',(14.18923641449,-2.85382213952302,3.32055549616167));
#87819=CARTESIAN_POINT('Ctrl Pts',(12.1667081232501,-0.879826986309144,
3.16253032741993));
#87820=CARTESIAN_POINT('Ctrl Pts',(12.7153248382468,1.89259023586425,3.0045051586782));
#87821=CARTESIAN_POINT('Ctrl Pts',(15.3372299062344,2.94752677607998,2.84647998993646));
#87822=CARTESIAN_POINT('Ctrl Pts',(17.6531068616151,1.32765302276885,2.68845482119473));
#87823=CARTESIAN_POINT('Ctrl Pts',(17.5613524460306,-1.49703456150004,2.53042965245299));
#87824=CARTESIAN_POINT('Ctrl Pts',(15.1452316123453,-2.96319831247482,2.37240448371126));
#87825=CARTESIAN_POINT('Ctrl Pts',(12.5973165460024,-1.74033121016063,2.21437931496952));
#87826=CARTESIAN_POINT('Ctrl Pts',(12.2297795593035,1.06184727517078,2.05635414622779));
#87827=CARTESIAN_POINT('Ctrl Pts',(14.3761517347936,2.90042031280201,1.89832897748605));
#87828=CARTESIAN_POINT('Ctrl Pts',(17.0886513586337,2.10693929935797,1.74030380874431));
#87829=CARTESIAN_POINT('Ctrl Pts',(17.9057495821698,-0.598555374153223,
1.58227864000258));
#87830=CARTESIAN_POINT('Ctrl Pts',(16.0859491279158,-2.76084337673324,1.42425347126084));
#87831=CARTESIAN_POINT('Ctrl Pts',(13.2806757688012,-2.41779390134308,1.26622830251911));
#87832=CARTESIAN_POINT('Ctrl Pts',(12.0356480620778,0.119467343019631,1.10820313377737));
#87833=CARTESIAN_POINT('Ctrl Pts',(13.4806995990586,2.54807825940933,0.950177965035635));
#87834=CARTESIAN_POINT('Ctrl Pts',(16.3044793779939,2.66483005208971,0.792152796293899));
#87835=CARTESIAN_POINT('Ctrl Pts',(17.94447665608,0.362412261618913,0.634127627552163));
#87836=CARTESIAN_POINT('Ctrl Pts',(16.9124276725532,-2.26712932015377,0.476102458810427));
#87837=CARTESIAN_POINT('Ctrl Pts',(14.1449117113466,-2.84275527328963,0.318077290068692));
#87838=CARTESIAN_POINT('Ctrl Pts',(12.1532501833424,-0.831660934158786,
0.160052121326955));
#87839=CARTESIAN_POINT('Ctrl Pts',(12.5484995178017,1.00129452861,0.0547020088324655));
#87840=CARTESIAN_POINT('Ctrl Pts',(13.0892024313212,1.63370573401717,0.00202695258522012));
#87841=CARTESIAN_POINT('Ctrl Pts',(13.0865340033349,1.6359872033749,-1.11022302462516E-15));
#87842=CARTESIAN_POINT('Ctrl Pts',(13.0246968436933,1.57787545757268,-1.42432143907935E-14));
#87843=CARTESIAN_POINT('Ctrl Pts',(12.9662508181783,1.51659301622886,-1.45896528824685E-14));
#87844=CARTESIAN_POINT('Ctrl Pts',(12.9111941550382,1.45252821261314,-9.15933995315754E-15));
#87845=CARTESIAN_POINT('Ctrl Pts',(12.8541852271874,1.38619172291679,-3.53647252279832E-15));
#87846=CARTESIAN_POINT('Ctrl Pts',(12.800809794498,1.31687166945573,-1.37441483129643E-14));
#87847=CARTESIAN_POINT('Ctrl Pts',(12.7510925676234,1.24494849184277,-1.2712053631958E-14));
#87848=CARTESIAN_POINT('Ctrl Pts',(12.7013753407488,1.17302531422982,-1.16799589509518E-14));
#87849=CARTESIAN_POINT('Ctrl Pts',(12.6553159499066,1.09849829006597,1.01924597636171E-14));
#87850=CARTESIAN_POINT('Ctrl Pts',(12.6129716803907,1.02170689819782,8.54871728961371E-15));
#87851=CARTESIAN_POINT('Ctrl Pts',(12.5833476634006,0.967983702039261,8.28664904516205E-15));
#87852=CARTESIAN_POINT('Ctrl Pts',(12.5555426419577,0.913151367850236,-1.61718727885097E-14));
#87853=CARTESIAN_POINT('Ctrl Pts',(12.5295872014039,0.85731712410759,2.27595720048157E-15));
#87854=CARTESIAN_POINT('Ctrl Pts',(12.5203776154169,0.837505853029321,9.14664374412348E-15));
#87855=CARTESIAN_POINT('Ctrl Pts',(12.5113986372893,0.817562575119292,6.86217500987582E-15));
#87856=CARTESIAN_POINT('Ctrl Pts',(12.5026676497318,0.797529280254451,3.94129173741931E-15));
#87857=CARTESIAN_POINT('Ctrl Pts',(12.4661263202705,0.713685016014067,-8.28332286359483E-15));
#87858=CARTESIAN_POINT('Ctrl Pts',(12.43387109168,0.628155083435122,3.282298611734E-15));
#87859=CARTESIAN_POINT('Ctrl Pts',(12.4059285496426,0.541340460493411,1.01030295240889E-14));
#87860=CARTESIAN_POINT('Ctrl Pts',(12.3776099242671,0.453357385048541,1.7015561792458E-14));
#87861=CARTESIAN_POINT('Ctrl Pts',(12.3537203794151,0.364054027731861,2.19382220206576E-16));
#87862=CARTESIAN_POINT('Ctrl Pts',(12.3343268282525,0.273810866462743,7.21644966006352E-16));
#87863=CARTESIAN_POINT('Ctrl Pts',(12.3149149474258,0.183482412571172,1.22438242153645E-15));
#87864=CARTESIAN_POINT('Ctrl Pts',(12.3000071430258,0.0922114838591795,
4.21376165523926E-15));
#87865=CARTESIAN_POINT('Ctrl Pts',(12.2897162151444,0.00035562118077955,
-6.02295990859147E-15));
#87866=CARTESIAN_POINT('Ctrl Pts',(12.2860706085107,-0.0321847236929611,
-9.6493637150612E-15));
#87867=CARTESIAN_POINT('Ctrl Pts',(12.2830048501706,-0.0647986307443293,
-1.48809799554544E-14));
#87868=CARTESIAN_POINT('Ctrl Pts',(12.2805254843104,-0.0974705972111431,
-1.60704782814491E-14));
#87869=CARTESIAN_POINT('Ctrl Pts',(12.2787625414514,-0.120701864082326,
-1.72889664486694E-14));
#87870=CARTESIAN_POINT('Ctrl Pts',(12.2772960875482,-0.14396248857046,6.72941439601323E-15));
#87871=CARTESIAN_POINT('Ctrl Pts',(12.2761287376726,-0.167246925725108,
1.13242748511766E-14));
#87872=CARTESIAN_POINT('Ctrl Pts',(12.2754686811477,-0.180412682618434,
1.4340930014615E-14));
#87873=CARTESIAN_POINT('Ctrl Pts',(12.2749044797864,-0.193582396115722,
1.77390633662612E-15));
#87874=CARTESIAN_POINT('Ctrl Pts',(12.2744366510455,-0.206746783659478,
-2.77555756156289E-16));
#87875=CARTESIAN_POINT('Ctrl Pts',(12.2709697976906,-0.304301715917482,
-1.83947143932132E-14));
#87876=CARTESIAN_POINT('Ctrl Pts',(12.2727842857417,-0.401695668560479,
-7.28963219131405E-15));
#87877=CARTESIAN_POINT('Ctrl Pts',(12.2799462946648,-0.498500550756148,
2.16493489801906E-15));
#87878=CARTESIAN_POINT('Ctrl Pts',(12.2871083035879,-0.595305432951817,
1.15216481752733E-14));
#87879=CARTESIAN_POINT('Ctrl Pts',(12.2996173861023,-0.691522324483779,
-1.87906254926288E-14));
#87880=CARTESIAN_POINT('Ctrl Pts',(12.3175936746857,-0.786742501729336,
-1.97064586870965E-14));
#87881=CARTESIAN_POINT('Ctrl Pts',(12.3346924509195,-0.877314506963681,
-2.23083733320138E-14));
#87882=CARTESIAN_POINT('Ctrl Pts',(12.3567376278471,-0.966985711385258,
-1.66241219421888E-14));
#87883=CARTESIAN_POINT('Ctrl Pts',(12.3834540669815,-1.05551643358463,-6.52256026967279E-15));
#87884=CARTESIAN_POINT('Ctrl Pts',(12.3924682953621,-1.08538703664647,-2.5035240808304E-15));
#87885=CARTESIAN_POINT('Ctrl Pts',(12.4020147482449,-1.11512776886543,-9.97226500510694E-15));
#87886=CARTESIAN_POINT('Ctrl Pts',(12.4120841660463,-1.14472924022538,-4.16333634234434E-16));
#87887=CARTESIAN_POINT('Ctrl Pts',(12.4191312473773,-1.16544582784787,6.94088720832354E-15));
#87888=CARTESIAN_POINT('Ctrl Pts',(12.4264344851179,-1.18609420448,-2.1092073521417E-14));
#87889=CARTESIAN_POINT('Ctrl Pts',(12.4339908862363,-1.20667110461397,-8.79851747015437E-15));
#87890=CARTESIAN_POINT('Ctrl Pts',(12.4399883408572,-1.22300282428556,6.32926458462707E-16));
#87891=CARTESIAN_POINT('Ctrl Pts',(12.4461461531738,-1.23929147885018,1.7986801302824E-14));
#87892=CARTESIAN_POINT('Ctrl Pts',(12.4524542218356,-1.25551398610641,1.68476343986868E-14));
#87893=CARTESIAN_POINT('Ctrl Pts',(12.4867496980242,-1.34371191817618,1.40459420071657E-14));
#87894=CARTESIAN_POINT('Ctrl Pts',(12.5255315419816,-1.43009348828233,9.21519657422252E-15));
#87895=CARTESIAN_POINT('Ctrl Pts',(12.5684561946922,-1.51441605785902,1.2712053631958E-14));
#87896=CARTESIAN_POINT('Ctrl Pts',(12.6122200752026,-1.60038723354108,1.62772783867871E-14));
#87897=CARTESIAN_POINT('Ctrl Pts',(12.6602906227897,-1.68421882699259,-8.03770240444636E-15));
#87898=CARTESIAN_POINT('Ctrl Pts',(12.712359022737,-1.76565063551856,-6.99440505513849E-15));
#87899=CARTESIAN_POINT('Ctrl Pts',(12.7652941152924,-1.84843789853507,-5.93374173910713E-15));
#87900=CARTESIAN_POINT('Ctrl Pts',(12.8223616208756,-1.92874565038163,9.00741210667174E-15));
#87901=CARTESIAN_POINT('Ctrl Pts',(12.8832886862843,-2.00628553627795,-4.12170297892089E-15));
#87902=CARTESIAN_POINT('Ctrl Pts',(12.9249302016807,-2.05928133265722,-1.30949933271466E-14));
#87903=CARTESIAN_POINT('Ctrl Pts',(12.9683756920542,-2.11098388168042,-1.09972078411733E-14));
#87904=CARTESIAN_POINT('Ctrl Pts',(13.0135501530493,-2.16129409957465,-1.51545442861334E-14));
#87905=CARTESIAN_POINT('Ctrl Pts',(13.0249459289848,-2.1739854290949,-1.58022044252471E-14));
#87906=CARTESIAN_POINT('Ctrl Pts',(13.0364525536874,-2.18658884793829,-6.82249416347656E-15));
#87907=CARTESIAN_POINT('Ctrl Pts',(13.0480570543102,-2.19909025794491,-8.09075029195583E-15));
#87908=CARTESIAN_POINT('Ctrl Pts',(13.1169652321276,-2.27332433416292,-1.62663069842411E-14));
#87909=CARTESIAN_POINT('Ctrl Pts',(13.1894126660034,-2.3440672132455,-1.00541840446858E-14));
#87910=CARTESIAN_POINT('Ctrl Pts',(13.2650848374145,-2.41102556089288,-1.13867248963118E-14));
#87911=CARTESIAN_POINT('Ctrl Pts',(13.3278852605644,-2.46659437155688,-1.24926021003911E-14));
#87912=CARTESIAN_POINT('Ctrl Pts',(13.3929077805362,-2.5195566145235,1.16609985742211E-14));
#87913=CARTESIAN_POINT('Ctrl Pts',(13.4599961723147,-2.56973093141732,1.08524300657109E-14));
#87914=CARTESIAN_POINT('Ctrl Pts',(13.4819381207051,-2.58614095769194,9.9633548728848E-15));
#87915=CARTESIAN_POINT('Ctrl Pts',(13.504101206195,-2.60225264132935,-1.12667630852908E-14));
#87916=CARTESIAN_POINT('Ctrl Pts',(13.5264803918495,-2.61805924925994,-1.21430643318376E-15));
#87917=CARTESIAN_POINT('Ctrl Pts',(13.5510376032739,-2.635404215196,7.9186405249631E-15));
#87918=CARTESIAN_POINT('Ctrl Pts',(13.5758604919219,-2.65238520209721,8.64516985986044E-15));
#87919=CARTESIAN_POINT('Ctrl Pts',(13.6009083282656,-2.66897104610506,4.15639744844043E-15));
#87920=CARTESIAN_POINT('Ctrl Pts',(13.6859725059094,-2.72529771487193,-1.10877828699206E-14));
#87921=CARTESIAN_POINT('Ctrl Pts',(13.7736934061109,-2.77711837429031,-5.52596575509762E-15));
#87922=CARTESIAN_POINT('Ctrl Pts',(13.863781021542,-2.82412395861086,-1.49186218934005E-16));
#87923=CARTESIAN_POINT('Ctrl Pts',(13.9456845295005,-2.86685926946434,4.73913392834114E-15));
#87924=CARTESIAN_POINT('Ctrl Pts',(14.0295451217468,-2.90561477915702,-2.80944019091112E-15));
#87925=CARTESIAN_POINT('Ctrl Pts',(14.1151705147995,-2.94013097355399,3.65939917257307E-15));
#87926=CARTESIAN_POINT('Ctrl Pts',(14.1446077022585,-2.9519973095626,5.89368974534453E-15));
#87927=CARTESIAN_POINT('Ctrl Pts',(14.1742536602921,-2.96336232955947,-4.71883449063881E-15));
#87928=CARTESIAN_POINT('Ctrl Pts',(14.204096742977,-2.97422942397538,-3.61516372393567E-15));
#87929=CARTESIAN_POINT('Ctrl Pts',(14.2062007174671,-2.96922295374569,6.));
#87930=CARTESIAN_POINT('Ctrl Pts',(14.112236572373,-2.93485044973517,6.));
#87931=CARTESIAN_POINT('Ctrl Pts',(14.0203776766673,-2.89562046290185,6.00000000000001));
#87932=CARTESIAN_POINT('Ctrl Pts',(13.9308389508323,-2.8518698079655,6.00000000000001));
#87933=CARTESIAN_POINT('Ctrl Pts',(13.8399807998063,-2.80747445191565,6.00000000000001));
#87934=CARTESIAN_POINT('Ctrl Pts',(13.7515110537651,-2.75842352890383,6.));
#87935=CARTESIAN_POINT('Ctrl Pts',(13.6656836450528,-2.70502293578984,6.));
#87936=CARTESIAN_POINT('Ctrl Pts',(13.579785175186,-2.65157812943612,6.));
#87937=CARTESIAN_POINT('Ctrl Pts',(13.4965328335216,-2.59377566615863,6.00000000000001));
#87938=CARTESIAN_POINT('Ctrl Pts',(13.416219602925,-2.53188766444664,6.00000000000001));
#87939=CARTESIAN_POINT('Ctrl Pts',(13.352988970228,-2.48316322047234,6.00000000000001));
#87940=CARTESIAN_POINT('Ctrl Pts',(13.2915807800382,-2.43190558434592,6.00000000000001));
#87941=CARTESIAN_POINT('Ctrl Pts',(13.2321583210611,-2.37823724421546,6.));
#87942=CARTESIAN_POINT('Ctrl Pts',(13.2181172434773,-2.36555582139089,6.));
#87943=CARTESIAN_POINT('Ctrl Pts',(13.2041844800433,-2.35273716244636,5.99999999999999));
#87944=CARTESIAN_POINT('Ctrl Pts',(13.1903814772932,-2.33980114775681,5.99999999999999));
#87945=CARTESIAN_POINT('Ctrl Pts',(13.1179418149603,-2.27191153322796,6.));
#87946=CARTESIAN_POINT('Ctrl Pts',(13.0489682803957,-2.20070050515602,6.));
#87947=CARTESIAN_POINT('Ctrl Pts',(12.9837009998789,-2.12645785153675,6.));
#87948=CARTESIAN_POINT('Ctrl Pts',(12.9187891629334,-2.05261952109033,6.00000000000001));
#87949=CARTESIAN_POINT('Ctrl Pts',(12.8575428342958,-1.97578170012202,6.));
#87950=CARTESIAN_POINT('Ctrl Pts',(12.8002418733548,-1.8962026816294,6.));
#87951=CARTESIAN_POINT('Ctrl Pts',(12.7442407816496,-1.81842890891738,6.));
#87952=CARTESIAN_POINT('Ctrl Pts',(12.6920077941674,-1.73803615732598,6.00000000000001));
#87953=CARTESIAN_POINT('Ctrl Pts',(12.6438514592926,-1.6552512354046,5.99999999999999));
#87954=CARTESIAN_POINT('Ctrl Pts',(12.6245372121835,-1.62204836722422,5.99999999999999));
#87955=CARTESIAN_POINT('Ctrl Pts',(12.6058793011271,-1.58846059039376,5.99999999999999));
#87956=CARTESIAN_POINT('Ctrl Pts',(12.5879000034355,-1.55450226629581,6.));
#87957=CARTESIAN_POINT('Ctrl Pts',(12.5746716428088,-1.52951725491477,6.00000000000001));
#87958=CARTESIAN_POINT('Ctrl Pts',(12.5618106681902,-1.50433165036472,6.));
#87959=CARTESIAN_POINT('Ctrl Pts',(12.5493264552966,-1.47895116667682,6.));
#87960=CARTESIAN_POINT('Ctrl Pts',(12.5425330890363,-1.46514021014923,6.));
#87961=CARTESIAN_POINT('Ctrl Pts',(12.5358504386754,-1.45126959011197,6.));
#87962=CARTESIAN_POINT('Ctrl Pts',(12.5292876124697,-1.43735666935141,6.));
#87963=CARTESIAN_POINT('Ctrl Pts',(12.4893045010192,-1.3525941228605,6.00000000000002));
#87964=CARTESIAN_POINT('Ctrl Pts',(12.4537027965796,-1.2661394597289,5.99999999999999));
#87965=CARTESIAN_POINT('Ctrl Pts',(12.4227270631163,-1.17822295375644,5.99999999999999));
#87966=CARTESIAN_POINT('Ctrl Pts',(12.3918924146296,-1.09070688053558,6.));
#87967=CARTESIAN_POINT('Ctrl Pts',(12.3656413201946,-1.00174159141967,5.99999999999999));
#87968=CARTESIAN_POINT('Ctrl Pts',(12.3442654767827,-0.911544935711397,
6.00000000000001));
#87969=CARTESIAN_POINT('Ctrl Pts',(12.3412853594997,-0.898970151766612,
6.00000000000001));
#87970=CARTESIAN_POINT('Ctrl Pts',(12.338400086203,-0.886371428596121,6.00000000000002));
#87971=CARTESIAN_POINT('Ctrl Pts',(12.3356105320368,-0.873749353237649,
6.00000000000002));
#87972=CARTESIAN_POINT('Ctrl Pts',(12.3150423389811,-0.780683125706667,
6.00000000000001));
#87973=CARTESIAN_POINT('Ctrl Pts',(12.2996737954968,-0.686346358438301,
6.00000000000002));
#87974=CARTESIAN_POINT('Ctrl Pts',(12.2894275798084,-0.591148428203356,
6.));
#87975=CARTESIAN_POINT('Ctrl Pts',(12.2835915289072,-0.536925485466267,
5.99999999999998));
#87976=CARTESIAN_POINT('Ctrl Pts',(12.2794182200608,-0.482423351119525,
6.));
#87977=CARTESIAN_POINT('Ctrl Pts',(12.2769004062244,-0.427720434386167,
6.00000000000001));
#87978=CARTESIAN_POINT('Ctrl Pts',(12.2763256322878,-0.415232691908223,
6.00000000000001));
#87979=CARTESIAN_POINT('Ctrl Pts',(12.2758372671371,-0.402736071144333,
5.99999999999998));
#87980=CARTESIAN_POINT('Ctrl Pts',(12.275435366957,-0.390240948305382,5.99999999999999));
#87981=CARTESIAN_POINT('Ctrl Pts',(12.2724465583895,-0.297318546064596,
5.99999999999999));
#87982=CARTESIAN_POINT('Ctrl Pts',(12.2742281667087,-0.204333268112907,
6.));
#87983=CARTESIAN_POINT('Ctrl Pts',(12.280645798089,-0.111657463647094,6.));
#87984=CARTESIAN_POINT('Ctrl Pts',(12.2870860503062,-0.0186549959419595,
6.));
#87985=CARTESIAN_POINT('Ctrl Pts',(12.2981954251014,0.0740367887701639,
6.00000000000001));
#87986=CARTESIAN_POINT('Ctrl Pts',(12.3138887533189,0.16602968371911,6.00000000000002));
#87987=CARTESIAN_POINT('Ctrl Pts',(12.3294516393369,0.25725793808997,6.00000000000002));
#87988=CARTESIAN_POINT('Ctrl Pts',(12.3495230165553,0.347799756950362,6.00000000000002));
#87989=CARTESIAN_POINT('Ctrl Pts',(12.3740635534643,0.437251017449185,6.00000000000001));
#87990=CARTESIAN_POINT('Ctrl Pts',(12.3831172052085,0.470251948261792,6.00000000000001));
#87991=CARTESIAN_POINT('Ctrl Pts',(12.3927795390774,0.503104129077211,6.00000000000001));
#87992=CARTESIAN_POINT('Ctrl Pts',(12.4030499280732,0.535786015862936,6.00000000000002));
#87993=CARTESIAN_POINT('Ctrl Pts',(12.4093064823122,0.555695290710277,6.00000000000002));
#87994=CARTESIAN_POINT('Ctrl Pts',(12.4157887023811,0.575541354183405,5.99999999999998));
#87995=CARTESIAN_POINT('Ctrl Pts',(12.422496569579,0.595319189801257,5.99999999999999));
#87996=CARTESIAN_POINT('Ctrl Pts',(12.4279638159807,0.611439112487062,6.00000000000001));
#87997=CARTESIAN_POINT('Ctrl Pts',(12.4335814641443,0.627514847993582,5.99999999999999));
#87998=CARTESIAN_POINT('Ctrl Pts',(12.4393433186991,0.643527071723061,5.99999999999999));
#87999=CARTESIAN_POINT('Ctrl Pts',(12.4699004093487,0.728445385323959,5.99999999999999));
#88000=CARTESIAN_POINT('Ctrl Pts',(12.5045458819893,0.81168828046424,5.99999999999999));
#88001=CARTESIAN_POINT('Ctrl Pts',(12.5432205607682,0.89288298252984,5.99999999999999));
#88002=CARTESIAN_POINT('Ctrl Pts',(12.5747843101636,0.959148800608798,5.99999999999999));
#88003=CARTESIAN_POINT('Ctrl Pts',(12.6090326915418,1.02405010401912,5.99999999999999));
#88004=CARTESIAN_POINT('Ctrl Pts',(12.6459520793395,1.087366283338,6.00000000000001));
#88005=CARTESIAN_POINT('Ctrl Pts',(12.6596302052844,1.11082405787692,6.00000000000002));
#88006=CARTESIAN_POINT('Ctrl Pts',(12.6736751071307,1.1340640732078,6.00000000000002));
#88007=CARTESIAN_POINT('Ctrl Pts',(12.6880866137171,1.15707441161647,6.));
#88008=CARTESIAN_POINT('Ctrl Pts',(12.6977797682187,1.1725511255875,5.99999999999999));
#88009=CARTESIAN_POINT('Ctrl Pts',(12.7076392245588,1.18792442723443,6.));
#88010=CARTESIAN_POINT('Ctrl Pts',(12.7176559765905,1.20317739777071,6.));
#88011=CARTESIAN_POINT('Ctrl Pts',(12.7648369644737,1.27502206516142,5.99999999999999));
#88012=CARTESIAN_POINT('Ctrl Pts',(12.8155498102687,1.34427270741682,6.00000000000001));
#88013=CARTESIAN_POINT('Ctrl Pts',(12.8697611773098,1.41057678007138,6.));
#88014=CARTESIAN_POINT('Ctrl Pts',(12.9190744293929,1.47089013550598,5.99999999999999));
#88015=CARTESIAN_POINT('Ctrl Pts',(12.971283147028,1.52876530435445,6.00000000000001));
#88016=CARTESIAN_POINT('Ctrl Pts',(13.0263834616836,1.58390596072205,6.00000000000001));
#88017=CARTESIAN_POINT('Ctrl Pts',(13.0449113026906,1.60244736689347,6.00000000000001));
#88018=CARTESIAN_POINT('Ctrl Pts',(13.0637662565083,1.62067930192608,5.99999999999999));
#88019=CARTESIAN_POINT('Ctrl Pts',(13.0829386709519,1.63859769523264,5.99999999999999));
#88020=CARTESIAN_POINT('Origin',(0.,0.,6.));
#88021=CARTESIAN_POINT('',(-25.,30.,6.));
#88022=CARTESIAN_POINT('',(-25.,-30.,6.));
#88023=CARTESIAN_POINT('',(-25.,30.,6.));
#88024=CARTESIAN_POINT('',(25.,-30.,6.));
#88025=CARTESIAN_POINT('',(-25.,-30.,6.));
#88026=CARTESIAN_POINT('',(25.,30.,6.));
#88027=CARTESIAN_POINT('',(25.,-30.,6.));
#88028=CARTESIAN_POINT('',(25.,30.,6.));
#88029=CARTESIAN_POINT('Ctrl Pts',(-13.0865340033349,1.63598720337492,6.));
#88030=CARTESIAN_POINT('Ctrl Pts',(-13.0246970130234,1.57787561670136,5.99999999999999));
#88031=CARTESIAN_POINT('Ctrl Pts',(-12.9662511655096,1.51659332338802,5.99999999999999));
#88032=CARTESIAN_POINT('Ctrl Pts',(-12.9111946833098,1.45252865944064,5.99999999999999));
#88033=CARTESIAN_POINT('Ctrl Pts',(-12.854185836343,1.38619219047224,6.));
#88034=CARTESIAN_POINT('Ctrl Pts',(-12.800810501265,1.31687213764253,6.));
#88035=CARTESIAN_POINT('Ctrl Pts',(-12.7510933826585,1.24494894576893,6.));
#88036=CARTESIAN_POINT('Ctrl Pts',(-12.701376264052,1.17302575389534,5.99999999999999));
#88037=CARTESIAN_POINT('Ctrl Pts',(-12.6553169921464,1.09849870057196,5.99999999999999));
#88038=CARTESIAN_POINT('Ctrl Pts',(-12.612972846328,1.02170726964558,6.));
#88039=CARTESIAN_POINT('Ctrl Pts',(-12.5941124949904,0.987503878857991,
6.));
#88040=CARTESIAN_POINT('Ctrl Pts',(-12.575989640936,0.952850788172522,6.00000000000002));
#88041=CARTESIAN_POINT('Ctrl Pts',(-12.5586117249717,0.917775962781449,
6.));
#88042=CARTESIAN_POINT('Ctrl Pts',(-12.5486939802334,0.89775842065026,5.99999999999999));
#88043=CARTESIAN_POINT('Ctrl Pts',(-12.5390188969959,0.877603494962885,
5.99999999999999));
#88044=CARTESIAN_POINT('Ctrl Pts',(-12.5295880909113,0.857316236876344,
5.99999999999999));
#88045=CARTESIAN_POINT('Ctrl Pts',(-12.5210550868119,0.838960302625967,
5.99999999999999));
#88046=CARTESIAN_POINT('Ctrl Pts',(-12.5127196692249,0.820490261091803,
6.00000000000002));
#88047=CARTESIAN_POINT('Ctrl Pts',(-12.5045967742098,0.80194176932807,6.00000000000001));
#88048=CARTESIAN_POINT('Ctrl Pts',(-12.4680063703819,0.718388208340872,
5.99999999999998));
#88049=CARTESIAN_POINT('Ctrl Pts',(-12.4356782866175,0.633150881056809,
6.00000000000001));
#88050=CARTESIAN_POINT('Ctrl Pts',(-12.4076382326647,0.546628236228551,
6.));
#88051=CARTESIAN_POINT('Ctrl Pts',(-12.3790534776866,0.458424818123778,
5.99999999999999));
#88052=CARTESIAN_POINT('Ctrl Pts',(-12.3549244489257,0.368884915467499,
6.));
#88053=CARTESIAN_POINT('Ctrl Pts',(-12.3353178885102,0.278393148285168,
6.00000000000001));
#88054=CARTESIAN_POINT('Ctrl Pts',(-12.3164053528586,0.191104570546898,
6.00000000000002));
#88055=CARTESIAN_POINT('Ctrl Pts',(-12.301700662964,0.102929389819606,6.00000000000001));
#88056=CARTESIAN_POINT('Ctrl Pts',(-12.2913042242818,0.0141911085737902,
6.00000000000001));
#88057=CARTESIAN_POINT('Ctrl Pts',(-12.2869540962369,-0.0229391913018656,
6.));
#88058=CARTESIAN_POINT('Ctrl Pts',(-12.2833587635632,-0.0601682677303705,
6.00000000000001));
#88059=CARTESIAN_POINT('Ctrl Pts',(-12.2805278793397,-0.0974730292652828,
6.00000000000001));
#88060=CARTESIAN_POINT('Ctrl Pts',(-12.2787649629962,-0.120704348035766,
6.));
#88061=CARTESIAN_POINT('Ctrl Pts',(-12.2772985351823,-0.143965023569731,
5.99999999999998));
#88062=CARTESIAN_POINT('Ctrl Pts',(-12.2761312108751,-0.167249510799076,
6.));
#88063=CARTESIAN_POINT('Ctrl Pts',(-12.2754711705252,-0.180415261740913,
6.00000000000002));
#88064=CARTESIAN_POINT('Ctrl Pts',(-12.2749069846676,-0.193584968987863,
6.00000000000001));
#88065=CARTESIAN_POINT('Ctrl Pts',(-12.2744391707337,-0.206749349931413,
6.00000000000001));
#88066=CARTESIAN_POINT('Ctrl Pts',(-12.2709724203682,-0.304304422879126,
6.00000000000002));
#88067=CARTESIAN_POINT('Ctrl Pts',(-12.2727869938187,-0.401698496843062,
5.99999999999999));
#88068=CARTESIAN_POINT('Ctrl Pts',(-12.2799490637078,-0.498503473694779,
5.99999999999999));
#88069=CARTESIAN_POINT('Ctrl Pts',(-12.2871111335968,-0.595308450546486,
6.));
#88070=CARTESIAN_POINT('Ctrl Pts',(-12.299620252658,-0.691525410085519,
6.));
#88071=CARTESIAN_POINT('Ctrl Pts',(-12.3175965465156,-0.78674562136694,
5.99999999999999));
#88072=CARTESIAN_POINT('Ctrl Pts',(-12.3347011817646,-0.877348667534142,
5.99999999999999));
#88073=CARTESIAN_POINT('Ctrl Pts',(-12.3567555739435,-0.967050265529378,
6.00000000000002));
#88074=CARTESIAN_POINT('Ctrl Pts',(-12.3834843158721,-1.05561049186739,
6.00000000000002));
#88075=CARTESIAN_POINT('Ctrl Pts',(-12.3924905257796,-1.08545072864266,
6.00000000000001));
#88076=CARTESIAN_POINT('Ctrl Pts',(-12.4020278760569,-1.11516134375352,
6.));
#88077=CARTESIAN_POINT('Ctrl Pts',(-12.4120871355902,-1.14473297565289,
5.99999999999999));
#88078=CARTESIAN_POINT('Ctrl Pts',(-12.4191345524566,-1.16545056592121,
5.99999999999999));
#88079=CARTESIAN_POINT('Ctrl Pts',(-12.4264381495643,-1.18609993714932,
6.00000000000002));
#88080=CARTESIAN_POINT('Ctrl Pts',(-12.433994933511,-1.20667782341152,6.00000000000001));
#88081=CARTESIAN_POINT('Ctrl Pts',(-12.43999210244,-1.22300872038934,6.));
#88082=CARTESIAN_POINT('Ctrl Pts',(-12.4461496119182,-1.23929655429101,
5.99999999999999));
#88083=CARTESIAN_POINT('Ctrl Pts',(-12.452457362016,-1.25551824623984,5.99999999999999));
#88084=CARTESIAN_POINT('Ctrl Pts',(-12.4867528525614,-1.34371623668614,
6.00000000000001));
#88085=CARTESIAN_POINT('Ctrl Pts',(-12.525534703178,-1.43009783582075,6.00000000000002));
#88086=CARTESIAN_POINT('Ctrl Pts',(-12.5684593590188,-1.51442040944555,
6.00000000000001));
#88087=CARTESIAN_POINT('Ctrl Pts',(-12.6122232164358,-1.60039153762029,
5.99999999999999));
#88088=CARTESIAN_POINT('Ctrl Pts',(-12.6602937320879,-1.68422306016549,
5.99999999999999));
#88089=CARTESIAN_POINT('Ctrl Pts',(-12.7123620962136,-1.76565477904875,
6.00000000000001));
#88090=CARTESIAN_POINT('Ctrl Pts',(-12.765297101908,-1.84844187204008,6.00000000000002));
#88091=CARTESIAN_POINT('Ctrl Pts',(-12.8223645087377,-1.92874943921375,
5.99999999999999));
#88092=CARTESIAN_POINT('Ctrl Pts',(-12.883291469427,-2.00628913114377,5.99999999999999));
#88093=CARTESIAN_POINT('Ctrl Pts',(-12.9249334864398,-2.05928552443159,
6.));
#88094=CARTESIAN_POINT('Ctrl Pts',(-12.9683795252804,-2.11098863042859,
6.00000000000001));
#88095=CARTESIAN_POINT('Ctrl Pts',(-13.0135545804225,-2.1612993628776,6.));
#88096=CARTESIAN_POINT('Ctrl Pts',(-13.0249491514721,-2.17398931341881,
6.));
#88097=CARTESIAN_POINT('Ctrl Pts',(-13.0364545470035,-2.18659137056383,
6.));
#88098=CARTESIAN_POINT('Ctrl Pts',(-13.04805779778,-2.19909144013573,5.99999999999999));
#88099=CARTESIAN_POINT('Ctrl Pts',(-13.1169657930863,-2.27332535543923,
5.99999999999999));
#88100=CARTESIAN_POINT('Ctrl Pts',(-13.1894130456957,-2.34406807252095,
6.00000000000002));
#88101=CARTESIAN_POINT('Ctrl Pts',(-13.2650850429559,-2.4110262629765,6.00000000000001));
#88102=CARTESIAN_POINT('Ctrl Pts',(-13.3278853347565,-2.46659495484805,
6.));
#88103=CARTESIAN_POINT('Ctrl Pts',(-13.3929077292049,-2.51955708123384,
6.00000000000001));
#88104=CARTESIAN_POINT('Ctrl Pts',(-13.459996004521,-2.56973128696733,5.99999999999999));
#88105=CARTESIAN_POINT('Ctrl Pts',(-13.4864139606169,-2.58948883712003,
5.99999999999999));
#88106=CARTESIAN_POINT('Ctrl Pts',(-13.5131517477184,-2.60881342412512,
5.99999999999999));
#88107=CARTESIAN_POINT('Ctrl Pts',(-13.5402031725862,-2.62769502775298,
5.99999999999999));
#88108=CARTESIAN_POINT('Ctrl Pts',(-13.5584328350526,-2.64041913610002,
6.));
#88109=CARTESIAN_POINT('Ctrl Pts',(-13.5768038646028,-2.65294113604551,
6.));
#88110=CARTESIAN_POINT('Ctrl Pts',(-13.5952986555222,-2.66524780668941,
6.));
#88111=CARTESIAN_POINT('Ctrl Pts',(-13.6802589908623,-2.72178150146766,
6.00000000000001));
#88112=CARTESIAN_POINT('Ctrl Pts',(-13.7678837405493,-2.77381421749709,
5.99999999999999));
#88113=CARTESIAN_POINT('Ctrl Pts',(-13.8578818875583,-2.82103744760724,
6.));
#88114=CARTESIAN_POINT('Ctrl Pts',(-13.9416560498191,-2.86499486976769,
6.));
#88115=CARTESIAN_POINT('Ctrl Pts',(-14.027487492673,-2.90478531313897,6.00000000000001));
#88116=CARTESIAN_POINT('Ctrl Pts',(-14.1151694615309,-2.94013049350043,
6.00000000000001));
#88117=CARTESIAN_POINT('Ctrl Pts',(-14.1445077395108,-2.95195694699142,
6.00000000000001));
#88118=CARTESIAN_POINT('Ctrl Pts',(-14.1740533905285,-2.9632854491535,6.));
#88119=CARTESIAN_POINT('Ctrl Pts',(-14.2037948851047,-2.97411935705757,
6.00000000000001));
#88120=CARTESIAN_POINT('Ctrl Pts',(-15.7937992825329,-2.96922295374568,
6.));
#88121=CARTESIAN_POINT('Ctrl Pts',(-15.8877632500353,-2.934850514699,6.));
#88122=CARTESIAN_POINT('Ctrl Pts',(-15.9796219674832,-2.89562055829788,
5.99999999999999));
#88123=CARTESIAN_POINT('Ctrl Pts',(-16.069160517518,-2.85186990831237,5.99999999999999));
#88124=CARTESIAN_POINT('Ctrl Pts',(-16.1600185833041,-2.80747451177071,
6.));
#88125=CARTESIAN_POINT('Ctrl Pts',(-16.2484882417351,-2.75842351247667,
6.00000000000001));
#88126=CARTESIAN_POINT('Ctrl Pts',(-16.334315563103,-2.70502281756701,6.));
#88127=CARTESIAN_POINT('Ctrl Pts',(-16.4202140639116,-2.65157783569215,
6.));
#88128=CARTESIAN_POINT('Ctrl Pts',(-16.5034664294958,-2.59377515931806,
6.));
#88129=CARTESIAN_POINT('Ctrl Pts',(-16.5837796785328,-2.53188691831275,
6.));
#88130=CARTESIAN_POINT('Ctrl Pts',(-16.6470102644641,-2.4831623331671,6.));
#88131=CARTESIAN_POINT('Ctrl Pts',(-16.7084184080196,-2.43190454453287,
5.99999999999999));
#88132=CARTESIAN_POINT('Ctrl Pts',(-16.7678408217129,-2.37823604579948,
6.00000000000001));
#88133=CARTESIAN_POINT('Ctrl Pts',(-16.7818820741009,-2.36555441795637,
6.00000000000001));
#88134=CARTESIAN_POINT('Ctrl Pts',(-16.7958150096753,-2.35273554990402,
6.00000000000001));
#88135=CARTESIAN_POINT('Ctrl Pts',(-16.8096181812999,-2.3397993227231,6.00000000000001));
#88136=CARTESIAN_POINT('Ctrl Pts',(-16.8820533727342,-2.2719136137154,6.00000000000001));
#88137=CARTESIAN_POINT('Ctrl Pts',(-16.9510228592216,-2.20070688840159,
6.00000000000001));
#88138=CARTESIAN_POINT('Ctrl Pts',(-17.0162865616681,-2.12646889315391,
6.00000000000001));
#88139=CARTESIAN_POINT('Ctrl Pts',(-17.0807779367567,-2.05310942659178,
6.00000000000001));
#88140=CARTESIAN_POINT('Ctrl Pts',(-17.1416511471808,-1.97678920349332,
5.99999999999999));
#88141=CARTESIAN_POINT('Ctrl Pts',(-17.1986318998573,-1.89776160004079,
5.99999999999999));
#88142=CARTESIAN_POINT('Ctrl Pts',(-17.2542709860764,-1.82059477728679,
5.99999999999999));
#88143=CARTESIAN_POINT('Ctrl Pts',(-17.3061990346064,-1.74084585335279,
6.00000000000002));
#88144=CARTESIAN_POINT('Ctrl Pts',(-17.3541147728116,-1.65873676591806,
6.));
#88145=CARTESIAN_POINT('Ctrl Pts',(-17.3741535582349,-1.62439801948437,
5.99999999999999));
#88146=CARTESIAN_POINT('Ctrl Pts',(-17.3934900117363,-1.58964637356626,
6.));
#88147=CARTESIAN_POINT('Ctrl Pts',(-17.4120994581939,-1.55449775528887,
6.00000000000001));
#88148=CARTESIAN_POINT('Ctrl Pts',(-17.4253278876833,-1.52951254040944,
6.00000000000002));
#88149=CARTESIAN_POINT('Ctrl Pts',(-17.4381889272245,-1.50432673226678,
6.00000000000001));
#88150=CARTESIAN_POINT('Ctrl Pts',(-17.4506732009798,-1.47894604526973,
6.00000000000001));
#88151=CARTESIAN_POINT('Ctrl Pts',(-17.4574664323557,-1.46513531966157,
6.00000000000001));
#88152=CARTESIAN_POINT('Ctrl Pts',(-17.464148952056,-1.45126493367676,6.));
#88153=CARTESIAN_POINT('Ctrl Pts',(-17.4707116522414,-1.43735224943686,
6.));
#88154=CARTESIAN_POINT('Ctrl Pts',(-17.5106947798987,-1.35258948193268,
6.00000000000002));
#88155=CARTESIAN_POINT('Ctrl Pts',(-17.5462964993568,-1.26613462526213,
6.));
#88156=CARTESIAN_POINT('Ctrl Pts',(-17.5772722477121,-1.1782179632567,5.99999999999999));
#88157=CARTESIAN_POINT('Ctrl Pts',(-17.6081069075101,-1.09070174468405,
5.99999999999999));
#88158=CARTESIAN_POINT('Ctrl Pts',(-17.6343580141732,-1.00173634769329,
6.00000000000001));
#88159=CARTESIAN_POINT('Ctrl Pts',(-17.6557338718008,-0.911539631838522,
5.99999999999999));
#88160=CARTESIAN_POINT('Ctrl Pts',(-17.6587139661113,-0.898964944805013,
5.99999999999998));
#88161=CARTESIAN_POINT('Ctrl Pts',(-17.6615992180624,-0.886366319875325,
5.99999999999998));
#88162=CARTESIAN_POINT('Ctrl Pts',(-17.6643887525347,-0.873744344101168,
5.99999999999998));
#88163=CARTESIAN_POINT('Ctrl Pts',(-17.6849486211246,-0.780715860016505,
6.));
#88164=CARTESIAN_POINT('Ctrl Pts',(-17.7003130610805,-0.686417920490627,
6.00000000000002));
#88165=CARTESIAN_POINT('Ctrl Pts',(-17.7105593084943,-0.591259391971915,
5.99999999999999));
#88166=CARTESIAN_POINT('Ctrl Pts',(-17.7164019038377,-0.53699828025407,
5.99999999999998));
#88167=CARTESIAN_POINT('Ctrl Pts',(-17.7205793832134,-0.482457537922925,
6.00000000000001));
#88168=CARTESIAN_POINT('Ctrl Pts',(-17.72309901058,-0.427715739212653,6.00000000000002));
#88169=CARTESIAN_POINT('Ctrl Pts',(-17.7236737899306,-0.415227997600035,
6.00000000000002));
#88170=CARTESIAN_POINT('Ctrl Pts',(-17.7241621603287,-0.402731378403247,
6.00000000000002));
#88171=CARTESIAN_POINT('Ctrl Pts',(-17.7245640655875,-0.390236257730834,
6.00000000000002));
#88172=CARTESIAN_POINT('Ctrl Pts',(-17.7275529071898,-0.297314018776729,
6.));
#88173=CARTESIAN_POINT('Ctrl Pts',(-17.7257713377121,-0.204328938103657,
6.00000000000001));
#88174=CARTESIAN_POINT('Ctrl Pts',(-17.7193537491782,-0.111653355453281,
6.));
#88175=CARTESIAN_POINT('Ctrl Pts',(-17.7129135394428,-0.0186511028990985,
6.));
#88176=CARTESIAN_POINT('Ctrl Pts',(-17.7018042104191,0.0740404418833223,
5.99999999999997));
#88177=CARTESIAN_POINT('Ctrl Pts',(-17.6861109294909,0.166033081375381,
5.99999999999998));
#88178=CARTESIAN_POINT('Ctrl Pts',(-17.6705480842034,0.257261118556288,
5.99999999999999));
#88179=CARTESIAN_POINT('Ctrl Pts',(-17.6504767456414,0.347802704397206,
6.));
#88180=CARTESIAN_POINT('Ctrl Pts',(-17.6259362435908,0.437253724644228,
6.));
#88181=CARTESIAN_POINT('Ctrl Pts',(-17.6168825703273,0.470254692135947,
6.));
#88182=CARTESIAN_POINT('Ctrl Pts',(-17.6072202097986,0.503106907518295,
6.00000000000001));
#88183=CARTESIAN_POINT('Ctrl Pts',(-17.5969497889173,0.535788826950787,
5.99999999999999));
#88184=CARTESIAN_POINT('Ctrl Pts',(-17.5906928388196,0.555699319553684,
5.99999999999998));
#88185=CARTESIAN_POINT('Ctrl Pts',(-17.5842101937972,0.575546592464114,
5.99999999999998));
#88186=CARTESIAN_POINT('Ctrl Pts',(-17.5775018725303,0.595325628334281,
5.99999999999999));
#88187=CARTESIAN_POINT('Ctrl Pts',(-17.572035158038,0.611443869803769,5.99999999999999));
#88188=CARTESIAN_POINT('Ctrl Pts',(-17.5664180723908,0.627517931614629,
6.));
#88189=CARTESIAN_POINT('Ctrl Pts',(-17.5606568093946,0.643528494331941,
6.));
#88190=CARTESIAN_POINT('Ctrl Pts',(-17.5300997600929,0.728446602500721,
5.99999999999998));
#88191=CARTESIAN_POINT('Ctrl Pts',(-17.4954543212718,0.811689292699246,
5.99999999999999));
#88192=CARTESIAN_POINT('Ctrl Pts',(-17.4567796672896,0.892883798280689,
5.99999999999999));
#88193=CARTESIAN_POINT('Ctrl Pts',(-17.4252159774462,0.959149373464304,
5.99999999999999));
#88194=CARTESIAN_POINT('Ctrl Pts',(-17.3909676562918,1.02405044300496,5.99999999999999));
#88195=CARTESIAN_POINT('Ctrl Pts',(-17.3540483284449,1.08736640274463,5.99999999999999));
#88196=CARTESIAN_POINT('Ctrl Pts',(-17.3403702095884,1.11082412186727,6.));
#88197=CARTESIAN_POINT('Ctrl Pts',(-17.3263253139819,1.13406408326418,6.00000000000001));
#88198=CARTESIAN_POINT('Ctrl Pts',(-17.3119138127385,1.157074369458,5.99999999999999));
#88199=CARTESIAN_POINT('Ctrl Pts',(-17.3022206458985,1.17255107374768,5.99999999999998));
#88200=CARTESIAN_POINT('Ctrl Pts',(-17.2923611762558,1.18792436616809,6.));
#88201=CARTESIAN_POINT('Ctrl Pts',(-17.2823444099864,1.20317732794761,6.));
#88202=CARTESIAN_POINT('Ctrl Pts',(-17.2351633869987,1.27502190542827,6.));
#88203=CARTESIAN_POINT('Ctrl Pts',(-17.1844504900327,1.34427247178924,6.));
#88204=CARTESIAN_POINT('Ctrl Pts',(-17.1302390543522,1.41057648897033,6.00000000000001));
#88205=CARTESIAN_POINT('Ctrl Pts',(-17.0809259142552,1.4708895806124,6.00000000000001));
#88206=CARTESIAN_POINT('Ctrl Pts',(-17.0287173146208,1.52876451979022,5.99999999999998));
#88207=CARTESIAN_POINT('Ctrl Pts',(-16.9736171227159,1.58390498876622,6.));
#88208=CARTESIAN_POINT('Ctrl Pts',(-16.9550892876871,1.60244636724923,6.00000000000001));
#88209=CARTESIAN_POINT('Ctrl Pts',(-16.936234339139,1.62067827820074,6.));
#88210=CARTESIAN_POINT('Ctrl Pts',(-16.9170619292826,1.6385966508594,6.));
#88211=CARTESIAN_POINT('',(-11.,1.34711147906209E-15,6.));
#88212=CARTESIAN_POINT('Origin',(0.,0.,6.));
#88213=CARTESIAN_POINT('Ctrl Pts',(-13.0907445586006,1.63408170136227,5.99751915277646));
#88214=CARTESIAN_POINT('Ctrl Pts',(-12.5496079497899,1.00187089822864,5.9448169085008));
#88215=CARTESIAN_POINT('Ctrl Pts',(-12.1539631618182,-0.831013794683539,
5.83943960797791));
#88216=CARTESIAN_POINT('Ctrl Pts',(-14.1452240851043,-2.84170398134258,
5.68138725120779));
#88217=CARTESIAN_POINT('Ctrl Pts',(-16.911723975924,-2.26629529617324,5.52336208246603));
#88218=CARTESIAN_POINT('Ctrl Pts',(-17.9433901746218,0.362279851730001,
5.36533691372431));
#88219=CARTESIAN_POINT('Ctrl Pts',(-16.303998759699,2.66384669060504,5.20731174498257));
#88220=CARTESIAN_POINT('Ctrl Pts',(-13.4812596174396,2.54713914628003,5.04928657624084));
#88221=CARTESIAN_POINT('Ctrl Pts',(-12.0367412189483,0.119423028973387,
4.8912614074991));
#88222=CARTESIAN_POINT('Ctrl Pts',(-13.2813096887287,-2.41690222892453,
4.73323623875736));
#88223=CARTESIAN_POINT('Ctrl Pts',(-16.0855487290697,-2.75982544810006,
4.57521107001563));
#88224=CARTESIAN_POINT('Ctrl Pts',(-17.9046781218851,-0.59833461826069,
4.41718590127389));
#88225=CARTESIAN_POINT('Ctrl Pts',(-17.0878812104006,2.10616237353801,4.25916073253216));
#88226=CARTESIAN_POINT('Ctrl Pts',(-14.3763817648042,2.89935084640419,4.10113556379042));
#88227=CARTESIAN_POINT('Ctrl Pts',(-12.2308010336203,1.06145572840915,3.94311039504869));
#88228=CARTESIAN_POINT('Ctrl Pts',(-12.5982024944047,-1.73968948755044,
3.78508522630695));
#88229=CARTESIAN_POINT('Ctrl Pts',(-15.1451780611008,-2.96210568514241,
3.62706005756521));
#88230=CARTESIAN_POINT('Ctrl Pts',(-17.5604079898984,-1.49648255368145,
3.46903488882348));
#88231=CARTESIAN_POINT('Ctrl Pts',(-17.652128572941,1.32716347219163,3.31100972008174));
#88232=CARTESIAN_POINT('Ctrl Pts',(-15.3371055582946,2.946439925236,3.15298455134001));
#88233=CARTESIAN_POINT('Ctrl Pts',(-12.7161672740172,1.89189237470017,2.99495938259826));
#88234=CARTESIAN_POINT('Ctrl Pts',(-12.16775285229,-0.879502564808503,2.83693421385654));
#88235=CARTESIAN_POINT('Ctrl Pts',(-14.1895353699199,-2.8527698401918,2.6789090451148));
#88236=CARTESIAN_POINT('Ctrl Pts',(-16.9467952172,-2.23721629994614,2.52088387637306));
#88237=CARTESIAN_POINT('Ctrl Pts',(-17.9373847982726,0.408557702420045,
2.36285870763132));
#88238=CARTESIAN_POINT('Ctrl Pts',(-16.2623673783843,2.68357554583426,2.20483353888959));
#88239=CARTESIAN_POINT('Ctrl Pts',(-13.441781916094,2.52331194313473,2.04680837014785));
#88240=CARTESIAN_POINT('Ctrl Pts',(-12.0352416641978,0.0732036971019031,
1.88878320140612));
#88241=CARTESIAN_POINT('Ctrl Pts',(-13.3191503210149,-2.4433369672288,1.73075803266438));
#88242=CARTESIAN_POINT('Ctrl Pts',(-16.1283876593297,-2.74260393131891,
1.57273286392265));
#88243=CARTESIAN_POINT('Ctrl Pts',(-17.9136447592549,-0.553029935281315,
1.41470769518091));
#88244=CARTESIAN_POINT('Ctrl Pts',(-17.0548293342031,2.13841897542678,1.25668252643918));
#88245=CARTESIAN_POINT('Ctrl Pts',(-14.3313231370429,2.88927738372614,1.09865735769744));
#88246=CARTESIAN_POINT('Ctrl Pts',(-12.2145902278525,1.0182363043339,0.940632188955702));
#88247=CARTESIAN_POINT('Ctrl Pts',(-12.6256188283705,-1.77692951890069,
0.782607020213967));
#88248=CARTESIAN_POINT('Ctrl Pts',(-15.1912084285039,-2.9593799210309,0.62458185147223));
#88249=CARTESIAN_POINT('Ctrl Pts',(-17.5835412498342,-1.45664222331674,
0.466556682730496));
#88250=CARTESIAN_POINT('Ctrl Pts',(-17.6308639198215,1.36870283349263,0.308531513988758));
#88251=CARTESIAN_POINT('Ctrl Pts',(-15.2917317296307,2.95053817591071,0.150506345247024));
#88252=CARTESIAN_POINT('Ctrl Pts',(-12.685918419667,1.85767322794601,-0.00751882349471303));
#88253=CARTESIAN_POINT('Ctrl Pts',(-12.183941158064,-0.926794243668898,
-0.165543992236448));
#88254=CARTESIAN_POINT('Ctrl Pts',(-13.5474245306813,-2.21298369896996,
-0.270894104730938));
#88255=CARTESIAN_POINT('Ctrl Pts',(-14.3509462720988,-2.42779915465415,
-0.323569160978183));
#88256=CARTESIAN_POINT('Ctrl Pts',(-12.9478680952619,1.75636592233901,6.1060964911164));
#88257=CARTESIAN_POINT('Ctrl Pts',(-12.3662362844088,1.07684450708003,6.05339424684075));
#88258=CARTESIAN_POINT('Ctrl Pts',(-11.9409839715256,-0.893201550913282,
5.94801694631786));
#88259=CARTESIAN_POINT('Ctrl Pts',(-14.081258123809,-3.05435892834755,5.78996458954772));
#88260=CARTESIAN_POINT('Ctrl Pts',(-17.0547851685949,-2.4358903381866,5.631939420806));
#88261=CARTESIAN_POINT('Ctrl Pts',(-18.1636546658245,0.389390558255529,
5.47391425206424));
#88262=CARTESIAN_POINT('Ctrl Pts',(-16.4015816849294,2.8631919357605,5.31588908332252));
#88263=CARTESIAN_POINT('Ctrl Pts',(-13.3676068029002,2.73775074542011,5.15786391458077));
#88264=CARTESIAN_POINT('Ctrl Pts',(-11.8149898883439,0.128359884488338,
4.99983874583904));
#88265=CARTESIAN_POINT('Ctrl Pts',(-13.1526939006449,-2.5977677303218,4.84181357709731));
#88266=CARTESIAN_POINT('Ctrl Pts',(-16.1667842514772,-2.96635312947079,
4.68378840835557));
#88267=CARTESIAN_POINT('Ctrl Pts',(-18.1220456507098,-0.643110153422998,
4.52576323961383));
#88268=CARTESIAN_POINT('Ctrl Pts',(-17.2441248835859,2.26377409202425,4.36773807087211));
#88269=CARTESIAN_POINT('Ctrl Pts',(-14.3297141654948,3.11631971601164,4.20971290213036));
#88270=CARTESIAN_POINT('Ctrl Pts',(-12.0235718981058,1.14088828477496,4.05168773338863));
#88271=CARTESIAN_POINT('Ctrl Pts',(-12.4184673338734,-1.86987671965101,
3.89366256464689));
#88272=CARTESIAN_POINT('Ctrl Pts',(-15.15604225846,-3.18377072542555,3.73563739590515));
#88273=CARTESIAN_POINT('Ctrl Pts',(-17.7520125444114,-1.60846973469552,
3.57761222716342));
#88274=CARTESIAN_POINT('Ctrl Pts',(-17.8505969091337,1.42647989631562,3.41958705842168));
#88275=CARTESIAN_POINT('Ctrl Pts',(-15.3623323817446,3.1669326402648,3.26156188967995));
#88276=CARTESIAN_POINT('Ctrl Pts',(-12.5452598429473,2.03346949720218,3.10353672093821));
#88277=CARTESIAN_POINT('Ctrl Pts',(-11.9558055942168,-0.945318910401867,
2.94551155219648));
#88278=CARTESIAN_POINT('Ctrl Pts',(-14.1288853817119,-3.0662528852825,2.78748638345474));
#88279=CARTESIAN_POINT('Ctrl Pts',(-17.0924809172101,-2.40463525590612,
2.62946121471301));
#88280=CARTESIAN_POINT('Ctrl Pts',(-18.157199885527,0.439131547242386,2.47143604597126));
#88281=CARTESIAN_POINT('Ctrl Pts',(-16.3568348773615,2.88439717230558,2.31341087722953));
#88282=CARTESIAN_POINT('Ctrl Pts',(-13.3251748429328,2.7121404668189,2.1553857084878));
#88283=CARTESIAN_POINT('Ctrl Pts',(-11.8133781165089,0.0786817934940617,
1.99736053974606));
#88284=CARTESIAN_POINT('Ctrl Pts',(-13.1933662837771,-2.62618067533236,
1.83933537100432));
#88285=CARTESIAN_POINT('Ctrl Pts',(-16.2128289732284,-2.94784286454329,
1.68131020226259));
#88286=CARTESIAN_POINT('Ctrl Pts',(-18.1316832938591,-0.594415157792721,
1.52328503352085));
#88287=CARTESIAN_POINT('Ctrl Pts',(-17.2085996164135,2.29844457164632,1.36525986477911));
#88288=CARTESIAN_POINT('Ctrl Pts',(-14.2812836382811,3.10549241982875,1.20723469603738));
#88289=CARTESIAN_POINT('Ctrl Pts',(-12.0061479793382,1.09443459548537,1.04920952729564));
#88290=CARTESIAN_POINT('Ctrl Pts',(-12.4479353308854,-1.90990355671544,
0.891184358553913));
#88291=CARTESIAN_POINT('Ctrl Pts',(-15.2055172440938,-3.1808409825652,0.733159189812176));
#88292=CARTESIAN_POINT('Ctrl Pts',(-17.7768769495327,-1.565648008873,0.575134021070441));
#88293=CARTESIAN_POINT('Ctrl Pts',(-17.827740945409,1.47112779768063,0.417108852328704));
#88294=CARTESIAN_POINT('Ctrl Pts',(-15.313563066009,3.17133757780266,0.259083683586969));
#88295=CARTESIAN_POINT('Ctrl Pts',(-12.5127473578457,1.99668960841177,0.101058514845233));
#88296=CARTESIAN_POINT('Ctrl Pts',(-11.973205329235,-0.99614959597368,-0.0569666538965035));
#88297=CARTESIAN_POINT('Ctrl Pts',(-13.4387230749784,-2.37858924209377,
-0.162316766390993));
#88298=CARTESIAN_POINT('Ctrl Pts',(-14.3023752432315,-2.60948011226316,
-0.214991822638238));
#88299=CARTESIAN_POINT('Ctrl Pts',(-12.8049916319232,1.87865014331576,6.21467382945635));
#88300=CARTESIAN_POINT('Ctrl Pts',(-12.1828646190277,1.15181811593143,6.1619715851807));
#88301=CARTESIAN_POINT('Ctrl Pts',(-11.7280047812329,-0.955389307143031,
6.05659428465781));
#88302=CARTESIAN_POINT('Ctrl Pts',(-14.0172921625136,-3.26701387535251,
5.89854192788767));
#88303=CARTESIAN_POINT('Ctrl Pts',(-17.1978463612657,-2.60548538019996,
5.74051675914593));
#88304=CARTESIAN_POINT('Ctrl Pts',(-18.3839191570272,0.416501264781063,
5.5824915904042));
#88305=CARTESIAN_POINT('Ctrl Pts',(-16.4991646101598,3.06253718091595,5.42446642166246));
#88306=CARTESIAN_POINT('Ctrl Pts',(-13.2539539883606,2.9283623445602,5.26644125292072));
#88307=CARTESIAN_POINT('Ctrl Pts',(-11.5932385577395,0.137296740003281,
5.10841608417899));
#88308=CARTESIAN_POINT('Ctrl Pts',(-13.024078112561,-2.77863323171906,4.95039091543725));
#88309=CARTESIAN_POINT('Ctrl Pts',(-16.2480197738846,-3.17288081084153,
4.79236574669552));
#88310=CARTESIAN_POINT('Ctrl Pts',(-18.3394131795346,-0.687885688585299,
4.63434057795378));
#88311=CARTESIAN_POINT('Ctrl Pts',(-17.4003685567714,2.42138581051048,4.47631540921205));
#88312=CARTESIAN_POINT('Ctrl Pts',(-14.2830465661856,3.33328858561909,4.31829024047031));
#88313=CARTESIAN_POINT('Ctrl Pts',(-11.8163427625913,1.22032084114078,4.16026507172857));
#88314=CARTESIAN_POINT('Ctrl Pts',(-12.238732173342,-2.00006395175156,4.00223990298685));
#88315=CARTESIAN_POINT('Ctrl Pts',(-15.1669064558191,-3.40543576570869,
3.8442147342451));
#88316=CARTESIAN_POINT('Ctrl Pts',(-17.9436170989244,-1.72045691570957,
3.68618956550337));
#88317=CARTESIAN_POINT('Ctrl Pts',(-18.0490652453263,1.5257963204396,3.52816439676163));
#88318=CARTESIAN_POINT('Ctrl Pts',(-15.3875592051944,3.38742535529361,3.3701392280199));
#88319=CARTESIAN_POINT('Ctrl Pts',(-12.3743524118776,2.17504661970418,3.21211405927816));
#88320=CARTESIAN_POINT('Ctrl Pts',(-11.7438583361436,-1.01113525599524,
3.05408889053642));
#88321=CARTESIAN_POINT('Ctrl Pts',(-14.0682353935039,-3.27973593037319,
2.89606372179469));
#88322=CARTESIAN_POINT('Ctrl Pts',(-17.2381666172201,-2.57205421186611,
2.73803855305295));
#88323=CARTESIAN_POINT('Ctrl Pts',(-18.3770149727813,0.469705392064734,
2.58001338431122));
#88324=CARTESIAN_POINT('Ctrl Pts',(-16.4513023763387,3.08521879877688,2.42198821556948));
#88325=CARTESIAN_POINT('Ctrl Pts',(-13.2085677697714,2.90096899050306,2.26396304682775));
#88326=CARTESIAN_POINT('Ctrl Pts',(-11.5915145688199,0.0841598898862171,
2.10593787808601));
#88327=CARTESIAN_POINT('Ctrl Pts',(-13.0675822465394,-2.80902438343592,
1.94791270934427));
#88328=CARTESIAN_POINT('Ctrl Pts',(-16.2972702871271,-3.15308179776768,
1.78988754060254));
#88329=CARTESIAN_POINT('Ctrl Pts',(-18.3497218284633,-0.635800380304125,
1.6318623718608));
#88330=CARTESIAN_POINT('Ctrl Pts',(-17.3623698986238,2.45847016786588,1.47383720311907));
#88331=CARTESIAN_POINT('Ctrl Pts',(-14.2312441395194,3.32170745593136,1.31581203437733));
#88332=CARTESIAN_POINT('Ctrl Pts',(-11.7977057308239,1.17063288663686,1.15778686563559));
#88333=CARTESIAN_POINT('Ctrl Pts',(-12.2702518334002,-2.04287759453019,
0.999761696893858));
#88334=CARTESIAN_POINT('Ctrl Pts',(-15.2198260596839,-3.40230204409951,
0.841736528152121));
#88335=CARTESIAN_POINT('Ctrl Pts',(-17.970212649231,-1.67465379442927,0.683711359410386));
#88336=CARTESIAN_POINT('Ctrl Pts',(-18.0246179709966,1.57355276186863,0.525686190668649));
#88337=CARTESIAN_POINT('Ctrl Pts',(-15.3353944023873,3.39213697969462,0.367661021926914));
#88338=CARTESIAN_POINT('Ctrl Pts',(-12.3395762960243,2.13570598887754,0.209635853185178));
#88339=CARTESIAN_POINT('Ctrl Pts',(-11.7624695004062,-1.06550494827847,
0.0516106844434421));
#88340=CARTESIAN_POINT('Ctrl Pts',(-13.3300216192754,-2.54419478521757,
-0.0537394280510476));
#88341=CARTESIAN_POINT('Ctrl Pts',(-14.2538042143642,-2.79116106987219,
-0.106414484298293));
#88342=CARTESIAN_POINT('Ctrl Pts',(-12.6621151685845,2.0009343642925,6.32325116779629));
#88343=CARTESIAN_POINT('Ctrl Pts',(-11.9994929536466,1.22679172478282,6.27054892352065));
#88344=CARTESIAN_POINT('Ctrl Pts',(-11.5150255909403,-1.01757706337277,
6.16517162299776));
#88345=CARTESIAN_POINT('Ctrl Pts',(-13.9533262012184,-3.47966882235748,
6.00711926622762));
#88346=CARTESIAN_POINT('Ctrl Pts',(-17.3409075539365,-2.77508042221333,
5.84909409748589));
#88347=CARTESIAN_POINT('Ctrl Pts',(-18.6041836482299,0.443611971306593,
5.69106892874414));
#88348=CARTESIAN_POINT('Ctrl Pts',(-16.5967475353903,3.2618824260714,5.53304376000242));
#88349=CARTESIAN_POINT('Ctrl Pts',(-13.1403011738212,3.11897394370029,5.37501859126067));
#88350=CARTESIAN_POINT('Ctrl Pts',(-11.3714872271351,0.146233595518226,
5.21699342251894));
#88351=CARTESIAN_POINT('Ctrl Pts',(-12.8954623244772,-2.95949873311632,
5.0589682537772));
#88352=CARTESIAN_POINT('Ctrl Pts',(-16.329255296292,-3.37940849221227,4.90094308503547));
#88353=CARTESIAN_POINT('Ctrl Pts',(-18.5567807083594,-0.732661223747603,
4.74291791629373));
#88354=CARTESIAN_POINT('Ctrl Pts',(-17.5566122299567,2.57899752899671,4.584892747552));
#88355=CARTESIAN_POINT('Ctrl Pts',(-14.2363789668763,3.55025745522654,4.42686757881026));
#88356=CARTESIAN_POINT('Ctrl Pts',(-11.6091136270768,1.2997533975066,4.26884241006853));
#88357=CARTESIAN_POINT('Ctrl Pts',(-12.0589970128107,-2.13025118385213,
4.11081724132679));
#88358=CARTESIAN_POINT('Ctrl Pts',(-15.1777706531783,-3.62710080599184,
3.95279207258505));
#88359=CARTESIAN_POINT('Ctrl Pts',(-18.1352216534374,-1.83244409672364,
3.79476690384331));
#88360=CARTESIAN_POINT('Ctrl Pts',(-18.247533581519,1.6251127445636,3.63674173510157));
#88361=CARTESIAN_POINT('Ctrl Pts',(-15.4127860286444,3.60791807032241,3.47871656635985));
#88362=CARTESIAN_POINT('Ctrl Pts',(-12.2034449808077,2.31662374220618,3.32069139761811));
#88363=CARTESIAN_POINT('Ctrl Pts',(-11.5319110780704,-1.0769516015886,3.16266622887638));
#88364=CARTESIAN_POINT('Ctrl Pts',(-14.0075854052959,-3.49321897546388,
3.00464106013463));
#88365=CARTESIAN_POINT('Ctrl Pts',(-17.3838523172302,-2.73947316782609,
2.8466158913929));
#88366=CARTESIAN_POINT('Ctrl Pts',(-18.5968300600357,0.500279236887077,
2.68859072265117));
#88367=CARTESIAN_POINT('Ctrl Pts',(-16.545769875316,3.28604042524819,2.53056555390943));
#88368=CARTESIAN_POINT('Ctrl Pts',(-13.0919606966101,3.08979751418722,2.37254038516769));
#88369=CARTESIAN_POINT('Ctrl Pts',(-11.3696510211309,0.0896379862783765,
2.21451521642595));
#88370=CARTESIAN_POINT('Ctrl Pts',(-12.9417982093016,-2.99186809153947,
2.05649004768421));
#88371=CARTESIAN_POINT('Ctrl Pts',(-16.3817116010259,-3.35832073099206,
1.89846487894248));
#88372=CARTESIAN_POINT('Ctrl Pts',(-18.5677603630673,-0.677185602815532,
1.74043971020074));
#88373=CARTESIAN_POINT('Ctrl Pts',(-17.5161401808341,2.61849576408543,1.58241454145901));
#88374=CARTESIAN_POINT('Ctrl Pts',(-14.1812046407576,3.53792249203398,1.42438937271727));
#88375=CARTESIAN_POINT('Ctrl Pts',(-11.5892634823095,1.24683117778833,1.26636420397553));
#88376=CARTESIAN_POINT('Ctrl Pts',(-12.0925683359151,-2.17585163234495,
1.1083390352338));
#88377=CARTESIAN_POINT('Ctrl Pts',(-15.2341348752738,-3.62376310563382,
0.950313866492068));
#88378=CARTESIAN_POINT('Ctrl Pts',(-18.1635483489294,-1.78365957998554,
0.792288697750331));
#88379=CARTESIAN_POINT('Ctrl Pts',(-18.2214949965841,1.67597772605664,0.634263529008596));
#88380=CARTESIAN_POINT('Ctrl Pts',(-15.3572257387657,3.61293638158657,0.476238360266859));
#88381=CARTESIAN_POINT('Ctrl Pts',(-12.1664052342031,2.27472236934331,0.318213191525124));
#88382=CARTESIAN_POINT('Ctrl Pts',(-11.5517336715772,-1.13486030058325,
0.160188022783388));
#88383=CARTESIAN_POINT('Ctrl Pts',(-13.2213201635726,-2.70980032834139,
0.0548379102888979));
#88384=CARTESIAN_POINT('Ctrl Pts',(-14.2052331854969,-2.97284202748121,
0.00216285404165282));
#88385=CARTESIAN_POINT('',(-13.0846966603782,1.6372236474585,-0.00127820437379453));
#88386=CARTESIAN_POINT('Ctrl Pts',(-14.2062007174672,-2.96922295374571,
-1.11022302462516E-15));
#88387=CARTESIAN_POINT('Ctrl Pts',(-14.1122367217159,-2.93485050436548,
5.64576421554524E-15));
#88388=CARTESIAN_POINT('Ctrl Pts',(-14.020377975911,-2.89562054314027,4.74471375630515E-15));
#88389=CARTESIAN_POINT('Ctrl Pts',(-13.9308393979082,-2.85186989239737,
-7.7715611723761E-16));
#88390=CARTESIAN_POINT('Ctrl Pts',(-13.8399813184291,-2.80747450226358,
-6.38040002655828E-15));
#88391=CARTESIAN_POINT('Ctrl Pts',(-13.7515116459329,-2.75842351507099,
-1.18049888343227E-15));
#88392=CARTESIAN_POINT('Ctrl Pts',(-13.6656843105487,-2.70502283631973,
1.0547118733939E-15));
#88393=CARTESIAN_POINT('Ctrl Pts',(-13.5797858146085,-2.65157788237369,
3.29177587242458E-15));
#88394=CARTESIAN_POINT('Ctrl Pts',(-13.4965334527781,-2.59377523991115,
7.44663497626135E-15));
#88395=CARTESIAN_POINT('Ctrl Pts',(-13.4162202066268,-2.53188703698736,
4.27435864480685E-15));
#88396=CARTESIAN_POINT('Ctrl Pts',(-13.3529896133675,-2.48316247442576,
1.77682649372841E-15));
#88397=CARTESIAN_POINT('Ctrl Pts',(-13.2915814624985,-2.43190471019256,
-1.27111200054493E-14));
#88398=CARTESIAN_POINT('Ctrl Pts',(-13.2321590416994,-2.37823623684125,
-8.27116153345742E-15));
#88399=CARTESIAN_POINT('Ctrl Pts',(-13.2181178171658,-2.36555464166943,
-7.6289592557529E-15));
#88400=CARTESIAN_POINT('Ctrl Pts',(-13.2041849090213,-2.35273580694004,
-1.00719496978036E-14));
#88401=CARTESIAN_POINT('Ctrl Pts',(-13.1903817643062,-2.33979961362129,
-8.10462807976364E-15));
#88402=CARTESIAN_POINT('Ctrl Pts',(-13.1179465671244,-2.27191394458243,
9.29987229349879E-15));
#88403=CARTESIAN_POINT('Ctrl Pts',(-13.0489770747074,-2.20070726068955,
3.12731471788556E-15));
#88404=CARTESIAN_POINT('Ctrl Pts',(-12.9837133664394,-2.12646930662299,
-7.7715611723761E-15));
#88405=CARTESIAN_POINT('Ctrl Pts',(-12.9192219935262,-2.05310988977285,
-1.8541458991958E-14));
#88406=CARTESIAN_POINT('Ctrl Pts',(-12.8583487844939,-1.97678971688283,
-1.95555689464262E-14));
#88407=CARTESIAN_POINT('Ctrl Pts',(-12.8013680326043,-1.8977621623991,-6.32827124036339E-15));
#88408=CARTESIAN_POINT('Ctrl Pts',(-12.7457289378947,-1.82059537461941,
6.58757920763005E-15));
#88409=CARTESIAN_POINT('Ctrl Pts',(-12.693800881531,-1.74084648362158,1.28239991180334E-14));
#88410=CARTESIAN_POINT('Ctrl Pts',(-12.6458851364556,-1.65873742553322,
-8.04911692853238E-16));
#88411=CARTESIAN_POINT('Ctrl Pts',(-12.6258463528357,-1.62439869938637,
-6.71154134295195E-15));
#88412=CARTESIAN_POINT('Ctrl Pts',(-12.6065099009786,-1.58964707331907,
1.33128856964392E-14));
#88413=CARTESIAN_POINT('Ctrl Pts',(-12.5879004560125,-1.55449847432752,
5.6621374255883E-15));
#88414=CARTESIAN_POINT('Ctrl Pts',(-12.5746720374845,-1.5295132918581,3.79392865924309E-16));
#88415=CARTESIAN_POINT('Ctrl Pts',(-12.5618110082776,-1.50432751614023,
-2.08393312802743E-14));
#88416=CARTESIAN_POINT('Ctrl Pts',(-12.5493267442101,-1.4789468615225,-1.93178806284777E-14));
#88417=CARTESIAN_POINT('Ctrl Pts',(-12.5425334913993,-1.46513609923887,
-1.72001277010202E-14));
#88418=CARTESIAN_POINT('Ctrl Pts',(-12.5358509509352,-1.45126567608035,
1.01097939998197E-14));
#88419=CARTESIAN_POINT('Ctrl Pts',(-12.5292882307234,-1.43735295427421,
6.07847105982273E-15));
#88420=CARTESIAN_POINT('Ctrl Pts',(-12.4893051056442,-1.35259022202115,
-1.96573038807791E-14));
#88421=CARTESIAN_POINT('Ctrl Pts',(-12.4537033885735,-1.26613539622463,
1.45565814917559E-14));
#88422=CARTESIAN_POINT('Ctrl Pts',(-12.4227276425839,-1.1782187591175,7.13318293321663E-15));
#88423=CARTESIAN_POINT('Ctrl Pts',(-12.3918929845728,-1.09070256371739,
-2.56403613302056E-16));
#88424=CARTESIAN_POINT('Ctrl Pts',(-12.3656418798435,-1.00173718392728,
-1.0741215117424E-14));
#88425=CARTESIAN_POINT('Ctrl Pts',(-12.3442660244676,-0.911540477667729,
-1.78190795452338E-14));
#88426=CARTESIAN_POINT('Ctrl Pts',(-12.3412859264738,-0.898965775105114,
-1.85340371603588E-14));
#88427=CARTESIAN_POINT('Ctrl Pts',(-12.3384006710999,-0.886367134434174,
-9.62165260182121E-15));
#88428=CARTESIAN_POINT('Ctrl Pts',(-12.3356111334694,-0.873745142704312,
-6.41153796721028E-15));
#88429=CARTESIAN_POINT('Ctrl Pts',(-12.315042930982,-0.780678937448357,
1.40106201757014E-14));
#88430=CARTESIAN_POINT('Ctrl Pts',(-12.299674369116,-0.686342237612556,
1.44936159865722E-14));
#88431=CARTESIAN_POINT('Ctrl Pts',(-12.28942812764,-0.591144411737914,-8.82627304576999E-15));
#88432=CARTESIAN_POINT('Ctrl Pts',(-12.2835920569734,-0.536921481269743,
-2.21088528726585E-14));
#88433=CARTESIAN_POINT('Ctrl Pts',(-12.2794187288502,-0.48241937068935,
-1.00134788350089E-14));
#88434=CARTESIAN_POINT('Ctrl Pts',(-12.2769008964915,-0.427716487911291,
1.80966353013901E-14));
#88435=CARTESIAN_POINT('Ctrl Pts',(-12.2763261180039,-0.415228746175687,
2.45270756093043E-14));
#88436=CARTESIAN_POINT('Ctrl Pts',(-12.2758377484422,-0.402732126744129,
2.70255838552933E-15));
#88437=CARTESIAN_POINT('Ctrl Pts',(-12.2754358439927,-0.390237005741378,
3.5527136788005E-15));
#88438=CARTESIAN_POINT('Ctrl Pts',(-12.2724426926483,-0.297180588281585,
8.8744226101631E-15));
#88439=CARTESIAN_POINT('Ctrl Pts',(-12.274233724762,-0.204061140642064,
2.30567975120578E-14));
#88440=CARTESIAN_POINT('Ctrl Pts',(-12.2806740030689,-0.111252623398913,
1.59594559789866E-14));
#88441=CARTESIAN_POINT('Ctrl Pts',(-12.2871453671104,-0.0179961408968059,
8.82785721896908E-15));
#88442=CARTESIAN_POINT('Ctrl Pts',(-12.2983113204397,0.0749473924486998,
2.19278460780688E-14));
#88443=CARTESIAN_POINT('Ctrl Pts',(-12.3140861273615,0.167186518104898,
1.25177646026486E-14));
#88444=CARTESIAN_POINT('Ctrl Pts',(-12.3296305385394,0.258078463914099,
3.24512016419198E-15));
#88445=CARTESIAN_POINT('Ctrl Pts',(-12.349650625959,0.348287277575547,-7.24335738920225E-15));
#88446=CARTESIAN_POINT('Ctrl Pts',(-12.3741075834303,0.4374131430529,-1.5404344466674E-15));
#88447=CARTESIAN_POINT('Ctrl Pts',(-12.3831485976605,0.470360340961913,
5.6776758695313E-16));
#88448=CARTESIAN_POINT('Ctrl Pts',(-12.392796332953,0.503159232797977,-2.0625677205409E-15));
#88449=CARTESIAN_POINT('Ctrl Pts',(-12.4030501659707,0.535788378267512,
-5.60662627435704E-15));
#88450=CARTESIAN_POINT('Ctrl Pts',(-12.4093070529646,0.555698676743727,
-7.86954492739309E-15));
#88451=CARTESIAN_POINT('Ctrl Pts',(-12.415789630245,0.575545756853617,2.60155169675598E-14));
#88452=CARTESIAN_POINT('Ctrl Pts',(-12.4224978791286,0.595324601387584,
2.53685961126848E-14));
#88453=CARTESIAN_POINT('Ctrl Pts',(-12.4279646784057,0.611443110834228,
2.47251388076511E-14));
#88454=CARTESIAN_POINT('Ctrl Pts',(-12.4335818537163,0.627517439423588,
-7.68104876148795E-15));
#88455=CARTESIAN_POINT('Ctrl Pts',(-12.4393432110049,0.643528266897872,
-6.0507154842071E-15));
#88456=CARTESIAN_POINT('Ctrl Pts',(-12.4710550424473,0.731655532172561,
3.64288882194921E-16));
#88457=CARTESIAN_POINT('Ctrl Pts',(-12.5071698359129,0.817978578845512,
1.73303171070469E-14));
#88458=CARTESIAN_POINT('Ctrl Pts',(-12.5476222825399,0.902080078937405,
1.96509475358653E-14));
#88459=CARTESIAN_POINT('Ctrl Pts',(-12.5779616175101,0.965156204006325,
2.14637817750454E-14));
#88460=CARTESIAN_POINT('Ctrl Pts',(-12.6107419363143,1.02698221352591,-5.06122749809775E-15));
#88461=CARTESIAN_POINT('Ctrl Pts',(-12.6459517365208,1.0873663829419,1.00891517362811E-14));
#88462=CARTESIAN_POINT('Ctrl Pts',(-12.6596298565035,1.11082411088935,1.63169981023069E-14));
#88463=CARTESIAN_POINT('Ctrl Pts',(-12.6736747531009,1.13406408087531,4.30095806415684E-15));
#88464=CARTESIAN_POINT('Ctrl Pts',(-12.6880862551922,1.15707437538469,2.73392419813945E-15));
#88465=CARTESIAN_POINT('Ctrl Pts',(-12.6997302261644,1.17566585874512,9.13452452349396E-16));
#88466=CARTESIAN_POINT('Ctrl Pts',(-12.7116130981113,1.19410637782525,-1.36214186568185E-15));
#88467=CARTESIAN_POINT('Ctrl Pts',(-12.723722803297,1.2123723319515,-2.56045185054177E-15));
#88468=CARTESIAN_POINT('Ctrl Pts',(-12.7711778313141,1.28395222192633,-7.25634105945887E-15));
#88469=CARTESIAN_POINT('Ctrl Pts',(-12.8221585037883,1.35292687972583,9.32156199594571E-15));
#88470=CARTESIAN_POINT('Ctrl Pts',(-12.8766328873954,1.41894276037641,4.6525283625698E-15));
#88471=CARTESIAN_POINT('Ctrl Pts',(-12.923917575018,1.47624566291498,5.99728087757576E-16));
#88472=CARTESIAN_POINT('Ctrl Pts',(-12.9738352609869,1.53131901243648,2.71861438742187E-14));
#88473=CARTESIAN_POINT('Ctrl Pts',(-13.0263829703992,1.58390514293349,1.23694457454526E-14));
#88474=CARTESIAN_POINT('Ctrl Pts',(-13.044910806381,1.60244652583416,6.24075109223694E-15));
#88475=CARTESIAN_POINT('Ctrl Pts',(-13.0637657557693,1.62067844062891,7.06479597108194E-15));
#88476=CARTESIAN_POINT('Ctrl Pts',(-13.0829381663571,1.63859681658414,2.10378589549087E-14));
#88477=CARTESIAN_POINT('Ctrl Pts',(-13.0863689594075,1.63579414673148,-0.00127820437379467));
#88478=CARTESIAN_POINT('Ctrl Pts',(-13.094817760828,1.64567796291114,-0.000852136249196398));
#88479=CARTESIAN_POINT('Ctrl Pts',(-13.1033431379554,1.65549632126644,-0.000426068124598269));
#88480=CARTESIAN_POINT('Ctrl Pts',(-13.1119440673944,1.66524804319138,0.));
#88481=CARTESIAN_POINT('Ctrl Pts',(-15.7948103993656,-2.97300505757792,
5.99773971486702));
#88482=CARTESIAN_POINT('Ctrl Pts',(-16.7787773788947,-2.70994893328083,
5.94506465861977));
#88483=CARTESIAN_POINT('Ctrl Pts',(-18.448455143976,-1.13492077598002,5.83971454612528));
#88484=CARTESIAN_POINT('Ctrl Pts',(-17.8337504113313,2.2748462209877,5.68168937738353));
#88485=CARTESIAN_POINT('Ctrl Pts',(-14.6427546314668,3.61313520212619,5.52366420864182));
#88486=CARTESIAN_POINT('Ctrl Pts',(-11.7783282110555,1.6760693608975,5.36563903990007));
#88487=CARTESIAN_POINT('Ctrl Pts',(-11.8362780796478,-1.78375726249727,
5.20761387115834));
#88488=CARTESIAN_POINT('Ctrl Pts',(-14.7658522558612,-3.62396206689039,
5.04958870241659));
#88489=CARTESIAN_POINT('Ctrl Pts',(-17.9075912210902,-2.17597096634872,
4.89156353367486));
#88490=CARTESIAN_POINT('Ctrl Pts',(-18.4109236680194,1.24689956054639,4.73353836493312));
#88491=CARTESIAN_POINT('Ctrl Pts',(-15.8188402958995,3.5381166513751,4.5755131961914));
#88492=CARTESIAN_POINT('Ctrl Pts',(-12.483721745114,2.6186394399734,4.41748802744966));
#88493=CARTESIAN_POINT('Ctrl Pts',(-11.4320438624152,-0.677222756500938,
4.25946285870792));
#88494=CARTESIAN_POINT('Ctrl Pts',(-13.6182125778512,-3.35850501831769,
4.10143768996618));
#88495=CARTESIAN_POINT('Ctrl Pts',(-17.05831473289,-2.99203226502705,3.94341252122444));
#88496=CARTESIAN_POINT('Ctrl Pts',(-18.6305481896681,0.0896429040657021,
3.78538735248272));
#88497=CARTESIAN_POINT('Ctrl Pts',(-16.9081440050834,3.08996706380467,3.62736218374098));
#88498=CARTESIAN_POINT('Ctrl Pts',(-13.4541453022121,3.28622074264122,3.46933701499924));
#88499=CARTESIAN_POINT('Ctrl Pts',(-11.4029725681304,0.500306689286977,
3.3113118462575));
#88500=CARTESIAN_POINT('Ctrl Pts',(-12.6160168715814,-2.7396234933372,3.15328667751578));
#88501=CARTESIAN_POINT('Ctrl Pts',(-15.9924690523316,-3.49341066179973,
2.99526150877404));
#88502=CARTESIAN_POINT('Ctrl Pts',(-18.4682792293058,-1.07701069806446,
2.8372363400323));
#88503=CARTESIAN_POINT('Ctrl Pts',(-17.7967084769259,2.31675086422845,2.67921117129056));
#88504=CARTESIAN_POINT('Ctrl Pts',(-14.5871913202092,3.60811605075546,2.52118600254882));
#88505=CARTESIAN_POINT('Ctrl Pts',(-11.7522882137895,1.62520192058609,2.3631608338071));
#88506=CARTESIAN_POINT('Ctrl Pts',(-11.8646063049427,-1.8325446496698,2.20513566506536));
#88507=CARTESIAN_POINT('Ctrl Pts',(-14.8222195917507,-3.62729983954678,
2.04711049632362));
#88508=CARTESIAN_POINT('Ctrl Pts',(-17.9411643715581,-2.1303680778752,1.88908532758189));
#88509=CARTESIAN_POINT('Ctrl Pts',(-18.3910724434807,1.29982471805251,1.73106015884016));
#88510=CARTESIAN_POINT('Ctrl Pts',(-15.7636629367787,3.55045227500164,1.57303499009842));
#88511=CARTESIAN_POINT('Ctrl Pts',(-12.4432474772716,2.57913904223364,1.41500982135668));
#88512=CARTESIAN_POINT('Ctrl Pts',(-11.4430241205592,-0.732701416452974,
1.25698465261494));
#88513=CARTESIAN_POINT('Ctrl Pts',(-13.6706717561852,-3.3795939532912,1.09895948387321));
#88514=CARTESIAN_POINT('Ctrl Pts',(-17.1046531716412,-2.95966109719462,
0.940934315131468));
#88515=CARTESIAN_POINT('Ctrl Pts',(-18.6287118598364,0.146241559192967,
0.782909146389736));
#88516=CARTESIAN_POINT('Ctrl Pts',(-16.8598009208359,3.11914519751865,0.624883977647998));
#88517=CARTESIAN_POINT('Ctrl Pts',(-13.4031647554911,3.26206124447765,0.466858808906264));
#88518=CARTESIAN_POINT('Ctrl Pts',(-11.3956187510643,0.443636597386532,
0.308833640164527));
#88519=CARTESIAN_POINT('Ctrl Pts',(-12.658963648928,-2.77523315149222,0.150808471422791));
#88520=CARTESIAN_POINT('Ctrl Pts',(-16.0467319118579,-3.47985905282973,
-0.00721669731894459));
#88521=CARTESIAN_POINT('Ctrl Pts',(-18.4847448337578,-1.01805770532123,
-0.16524186606068));
#88522=CARTESIAN_POINT('Ctrl Pts',(-18.0009214582863,1.22570085496208,-0.27059197855517));
#88523=CARTESIAN_POINT('Ctrl Pts',(-17.3390382616395,1.99984565752206,-0.323267034802415));
#88524=CARTESIAN_POINT('Ctrl Pts',(-15.7463046910186,-2.79156843275239,
6.10617103348288));
#88525=CARTESIAN_POINT('Ctrl Pts',(-16.6702221098346,-2.54456610399477,
6.05349597723563));
#88526=CARTESIAN_POINT('Ctrl Pts',(-18.238002739736,-1.06565880331255,5.94814586474115));
#88527=CARTESIAN_POINT('Ctrl Pts',(-17.6608122224375,2.13601685058987,5.7901206959994));
#88528=CARTESIAN_POINT('Ctrl Pts',(-14.6645566104899,3.39263269929958,5.63209552725768));
#88529=CARTESIAN_POINT('Ctrl Pts',(-11.9749404751994,1.57378215925296,5.47407035851593));
#88530=CARTESIAN_POINT('Ctrl Pts',(-12.0293537778045,-1.67489808097969,
5.31604518977421));
#88531=CARTESIAN_POINT('Ctrl Pts',(-14.7801418300746,-3.40279882189813,
5.15802002103245));
#88532=CARTESIAN_POINT('Ctrl Pts',(-17.7301466734657,-2.04317575739126,
4.99999485229074));
#88533=CARTESIAN_POINT('Ctrl Pts',(-18.2027617356052,1.17080374389605,4.84196968354898));
#88534=CARTESIAN_POINT('Ctrl Pts',(-15.7688680904435,3.32219238248486,4.68394451480727));
#88535=CARTESIAN_POINT('Ctrl Pts',(-12.6372852355376,2.45882904866149,4.52591934606551));
#88536=CARTESIAN_POINT('Ctrl Pts',(-11.6497891761942,-0.635893189677169,
4.36789417732379));
#88537=CARTESIAN_POINT('Ctrl Pts',(-13.7025403341938,-3.15354209252986,
4.20986900858204));
#88538=CARTESIAN_POINT('Ctrl Pts',(-16.9326998514042,-2.80943444732343,
4.05184383984032));
#88539=CARTESIAN_POINT('Ctrl Pts',(-18.4089830066151,0.0841721747402409,
3.89381867109857));
#88540=CARTESIAN_POINT('Ctrl Pts',(-16.7916937464197,2.9013924788238,3.73579350235685));
#88541=CARTESIAN_POINT('Ctrl Pts',(-13.5484857602353,3.08566918338413,3.57776833361511));
#88542=CARTESIAN_POINT('Ctrl Pts',(-11.6224920455628,0.469773960507896,
3.41974316487337));
#88543=CARTESIAN_POINT('Ctrl Pts',(-12.7615066518153,-2.57242968427965,
3.26171799613163));
#88544=CARTESIAN_POINT('Ctrl Pts',(-15.9319006269131,-3.28021471112657,
3.1036928273899));
#88545=CARTESIAN_POINT('Ctrl Pts',(-18.2566170003051,-1.01128286303783,
2.94566765864816));
#88546=CARTESIAN_POINT('Ctrl Pts',(-17.626030884104,2.17536413624566,2.78764248990643));
#88547=CARTESIAN_POINT('Ctrl Pts',(-14.6123842183408,3.38791985682055,2.62961732116469));
#88548=CARTESIAN_POINT('Ctrl Pts',(-11.9504896475187,1.52601905832371,2.47159215242296));
#88549=CARTESIAN_POINT('Ctrl Pts',(-12.0559531874784,-1.72070807030351,
2.31356698368122));
#88550=CARTESIAN_POINT('Ctrl Pts',(-14.8330691788211,-3.40593289688381,
2.15554181493948));
#88551=CARTESIAN_POINT('Ctrl Pts',(-17.7616709208919,-2.00035592310254,
1.99751664619775));
#88552=CARTESIAN_POINT('Ctrl Pts',(-18.1841219920795,1.22049898360509,1.83949147745601));
#88553=CARTESIAN_POINT('Ctrl Pts',(-15.7170580965346,3.33377518737326,1.68146630871428));
#88554=CARTESIAN_POINT('Ctrl Pts',(-12.5992810322955,2.4217392821539,1.52344113997254));
#88555=CARTESIAN_POINT('Ctrl Pts',(-11.6600993308776,-0.687986096622873,
1.3654159712308));
#88556=CARTESIAN_POINT('Ctrl Pts',(-13.751798032519,-3.17334401146786,1.20739080248907));
#88557=CARTESIAN_POINT('Ctrl Pts',(-16.9762103467904,-2.77903882790729,
1.04936563374733));
#88558=CARTESIAN_POINT('Ctrl Pts',(-18.4072587443651,0.137316725768431,
0.891340465005602));
#88559=CARTESIAN_POINT('Ctrl Pts',(-16.7463009450912,2.92878992868517,0.733315296263867));
#88560=CARTESIAN_POINT('Ctrl Pts',(-13.5006164555573,3.06298409166098,0.57529012752213));
#88561=CARTESIAN_POINT('Ctrl Pts',(-11.615587017423,0.416562332351654,0.417264958780395));
#88562=CARTESIAN_POINT('Ctrl Pts',(-12.8018324721914,-2.60586615535233,
0.259239790038659));
#88563=CARTESIAN_POINT('Ctrl Pts',(-15.9828519313309,-3.26749013007776,
0.101214621296923));
#88564=CARTESIAN_POINT('Ctrl Pts',(-18.2720777414488,-0.955927654966856,
-0.0568105474448126));
#88565=CARTESIAN_POINT('Ctrl Pts',(-17.8177811506805,1.15089875343075,-0.162160659939302));
#88566=CARTESIAN_POINT('Ctrl Pts',(-17.1962913778265,1.87779902818723,-0.214835716186548));
#88567=CARTESIAN_POINT('Ctrl Pts',(-15.6977989826716,-2.61013180792686,
6.21460235209875));
#88568=CARTESIAN_POINT('Ctrl Pts',(-16.5616668407743,-2.3791832747087,6.16192729585151));
#88569=CARTESIAN_POINT('Ctrl Pts',(-18.0275503354958,-0.996396830645096,
6.05657718335701));
#88570=CARTESIAN_POINT('Ctrl Pts',(-17.4878740335435,1.99718748019203,5.89855201461528));
#88571=CARTESIAN_POINT('Ctrl Pts',(-14.6863585895132,3.17213019647298,5.74052684587355));
#88572=CARTESIAN_POINT('Ctrl Pts',(-12.1715527393434,1.47149495760841,5.5825016771318));
#88573=CARTESIAN_POINT('Ctrl Pts',(-12.2224294759612,-1.56603889946212,
5.42447650839008));
#88574=CARTESIAN_POINT('Ctrl Pts',(-14.7944314042879,-3.18163557690586,
5.26645133964833));
#88575=CARTESIAN_POINT('Ctrl Pts',(-17.5527021258414,-1.9103805484338,5.10842617090661));
#88576=CARTESIAN_POINT('Ctrl Pts',(-17.9945998031909,1.09470792724571,4.95040100216485));
#88577=CARTESIAN_POINT('Ctrl Pts',(-15.7188958849874,3.10626811359462,4.79237583342314));
#88578=CARTESIAN_POINT('Ctrl Pts',(-12.7908487259611,2.29901865734959,4.63435066468138));
#88579=CARTESIAN_POINT('Ctrl Pts',(-11.8675344899732,-0.594563622853398,
4.47632549593967));
#88580=CARTESIAN_POINT('Ctrl Pts',(-13.7868680905366,-2.94857916674204,
4.31830032719791));
#88581=CARTESIAN_POINT('Ctrl Pts',(-16.8070849699184,-2.62683662961979,
4.16027515845619));
#88582=CARTESIAN_POINT('Ctrl Pts',(-18.1874178235621,0.0787014454147784,
4.00224998971444));
#88583=CARTESIAN_POINT('Ctrl Pts',(-16.675243487756,2.71281789384293,3.84422482097272));
#88584=CARTESIAN_POINT('Ctrl Pts',(-13.6428262182586,2.88511762412704,3.68619965223097));
#88585=CARTESIAN_POINT('Ctrl Pts',(-11.8420115229951,0.439241231728813,
3.52817448348925));
#88586=CARTESIAN_POINT('Ctrl Pts',(-12.9069964320492,-2.40523587522208,
3.3701493147475));
#88587=CARTESIAN_POINT('Ctrl Pts',(-15.8713322014946,-3.0670187604534,3.21212414600578));
#88588=CARTESIAN_POINT('Ctrl Pts',(-18.0449547713042,-0.945555028011206,
3.05409897726403));
#88589=CARTESIAN_POINT('Ctrl Pts',(-17.4553532912823,2.03397740826286,2.8960738085223));
#88590=CARTESIAN_POINT('Ctrl Pts',(-14.6375771164722,3.16772366288563,2.73804863978056));
#88591=CARTESIAN_POINT('Ctrl Pts',(-12.1486910812479,1.42683619606133,2.58002347103883));
#88592=CARTESIAN_POINT('Ctrl Pts',(-12.2473000700141,-1.60887149093723,
2.42199830229709));
#88593=CARTESIAN_POINT('Ctrl Pts',(-14.8439187658915,-3.18456595422084,
2.26397313355535));
#88594=CARTESIAN_POINT('Ctrl Pts',(-17.5821774702257,-1.87034376832987,
2.10594796481362));
#88595=CARTESIAN_POINT('Ctrl Pts',(-17.9771715406782,1.14117324915768,1.94792279607189));
#88596=CARTESIAN_POINT('Ctrl Pts',(-15.6704532562904,3.11709809974488,1.78989762733015));
#88597=CARTESIAN_POINT('Ctrl Pts',(-12.7553145873195,2.26433952207416,1.63187245858841));
#88598=CARTESIAN_POINT('Ctrl Pts',(-11.8771745411961,-0.643270776792767,
1.47384728984667));
#88599=CARTESIAN_POINT('Ctrl Pts',(-13.8329243088529,-2.96709406964454,
1.31582212110494));
#88600=CARTESIAN_POINT('Ctrl Pts',(-16.8477675219395,-2.59841655861997,
1.1577969523632));
#88601=CARTESIAN_POINT('Ctrl Pts',(-18.1858056288936,0.128391892343889,
0.999771783621469));
#88602=CARTESIAN_POINT('Ctrl Pts',(-16.6328009693466,2.73843465985169,0.841746614879735));
#88603=CARTESIAN_POINT('Ctrl Pts',(-13.5980681556234,2.8639069388443,0.683721446137999));
#88604=CARTESIAN_POINT('Ctrl Pts',(-11.8355552837818,0.389488067316777,
0.525696277396263));
#88605=CARTESIAN_POINT('Ctrl Pts',(-12.9447012954548,-2.43649915921244,
0.367671108654526));
#88606=CARTESIAN_POINT('Ctrl Pts',(-15.9189719508039,-3.05512120732578,
0.209645939912791));
#88607=CARTESIAN_POINT('Ctrl Pts',(-18.0594106491397,-0.893797604612488,
0.0516207711710548));
#88608=CARTESIAN_POINT('Ctrl Pts',(-17.6346408430749,1.07609665189943,-0.0537293413234345));
#88609=CARTESIAN_POINT('Ctrl Pts',(-17.0535444940135,1.7557523988524,-0.10640439757068));
#88610=CARTESIAN_POINT('Ctrl Pts',(-15.6492932743244,-2.42869518310133,
6.32303367071462));
#88611=CARTESIAN_POINT('Ctrl Pts',(-16.4531115717142,-2.21380044542264,
6.27035861446738));
#88612=CARTESIAN_POINT('Ctrl Pts',(-17.8170979312557,-0.927134857977634,
6.16500850197289));
#88613=CARTESIAN_POINT('Ctrl Pts',(-17.3149358446497,1.85835810979419,6.00698333323115));
#88614=CARTESIAN_POINT('Ctrl Pts',(-14.7081605685364,2.95162769364637,5.84895816448941));
#88615=CARTESIAN_POINT('Ctrl Pts',(-12.3681650034873,1.36920775596387,5.69093299574768));
#88616=CARTESIAN_POINT('Ctrl Pts',(-12.4155051741179,-1.45717971794455,
5.53290782700594));
#88617=CARTESIAN_POINT('Ctrl Pts',(-14.8087209785013,-2.96047233191359,
5.3748826582642));
#88618=CARTESIAN_POINT('Ctrl Pts',(-17.375257578217,-1.77758533947633,5.21685748952248));
#88619=CARTESIAN_POINT('Ctrl Pts',(-17.7864378707766,1.01861211059538,5.05883232078073));
#88620=CARTESIAN_POINT('Ctrl Pts',(-15.6689236795314,2.89034384470437,4.90080715203901));
#88621=CARTESIAN_POINT('Ctrl Pts',(-12.9444122163845,2.1392082660377,4.74278198329726));
#88622=CARTESIAN_POINT('Ctrl Pts',(-12.0852798037522,-0.55323405602963,
4.58475681455553));
#88623=CARTESIAN_POINT('Ctrl Pts',(-13.8711958468793,-2.74361624095422,
4.42673164581379));
#88624=CARTESIAN_POINT('Ctrl Pts',(-16.6814700884327,-2.44423881191615,
4.26870647707206));
#88625=CARTESIAN_POINT('Ctrl Pts',(-17.965852640509,0.0732307160893165,
4.11068130833032));
#88626=CARTESIAN_POINT('Ctrl Pts',(-16.5587932290923,2.52424330886206,3.95265613958859));
#88627=CARTESIAN_POINT('Ctrl Pts',(-13.7371666762818,2.68456606486995,3.79463097084684));
#88628=CARTESIAN_POINT('Ctrl Pts',(-12.0615310004275,0.408708502949732,
3.63660580210512));
#88629=CARTESIAN_POINT('Ctrl Pts',(-13.052486212283,-2.23804206616453,3.47858063336337));
#88630=CARTESIAN_POINT('Ctrl Pts',(-15.8107637760761,-2.85382280978022,
3.32055546462165));
#88631=CARTESIAN_POINT('Ctrl Pts',(-17.8332925423033,-0.879827192984582,
3.1625302958799));
#88632=CARTESIAN_POINT('Ctrl Pts',(-17.2846756984605,1.89259068028007,3.00450512713817));
#88633=CARTESIAN_POINT('Ctrl Pts',(-14.6627700146037,2.94752746895072,2.84647995839643));
#88634=CARTESIAN_POINT('Ctrl Pts',(-12.3468925149772,1.32765333379895,2.6884547896547));
#88635=CARTESIAN_POINT('Ctrl Pts',(-12.4386469525498,-1.49703491157095,
2.53042962091296));
#88636=CARTESIAN_POINT('Ctrl Pts',(-14.8547683529619,-2.96319901155788,
2.37240445217123));
#88637=CARTESIAN_POINT('Ctrl Pts',(-17.4026840195596,-1.74033161355722,
2.21437928342949));
#88638=CARTESIAN_POINT('Ctrl Pts',(-17.7702210892769,1.06184751471027,2.05635411468776));
#88639=CARTESIAN_POINT('Ctrl Pts',(-15.6238484160462,2.9004210121165,1.89832894594602));
#88640=CARTESIAN_POINT('Ctrl Pts',(-12.9113481423434,2.10693976199442,1.74030377720429));
#88641=CARTESIAN_POINT('Ctrl Pts',(-12.0942497515145,-0.598555456962666,
1.58227860846254));
#88642=CARTESIAN_POINT('Ctrl Pts',(-13.9140505851867,-2.7608441278212,1.42425343972081));
#88643=CARTESIAN_POINT('Ctrl Pts',(-16.7193246970888,-2.41779428933264,
1.26622827097907));
#88644=CARTESIAN_POINT('Ctrl Pts',(-17.9643525134221,0.119467058919352,
1.10820310223734));
#88645=CARTESIAN_POINT('Ctrl Pts',(-16.5193009936019,2.54807939101821,0.950177933495602));
#88646=CARTESIAN_POINT('Ctrl Pts',(-13.6955198556895,2.66482978602762,0.792152764753866));
#88647=CARTESIAN_POINT('Ctrl Pts',(-12.0555235501407,0.3624138022819,0.634127596012131));
#88648=CARTESIAN_POINT('Ctrl Pts',(-13.0875701187183,-2.26713216307256,
0.476102427270394));
#88649=CARTESIAN_POINT('Ctrl Pts',(-15.855091970277,-2.84275228457381,0.318077258528659));
#88650=CARTESIAN_POINT('Ctrl Pts',(-17.8467435568307,-0.831667554258123,
0.160052089786923));
#88651=CARTESIAN_POINT('Ctrl Pts',(-17.4515005354693,1.00129455036811,0.0547019772924332));
#88652=CARTESIAN_POINT('Ctrl Pts',(-16.9107976102004,1.63370576951757,0.00202692104518772));
#88653=CARTESIAN_POINT('Ctrl Pts',(-16.913465996665,1.63598720337497,0.));
#88654=CARTESIAN_POINT('Ctrl Pts',(-16.9753029548724,1.57787564687154,-1.79744279815451E-14));
#88655=CARTESIAN_POINT('Ctrl Pts',(-17.0337487686381,1.5165933816238,-6.03303120349772E-15));
#88656=CARTESIAN_POINT('Ctrl Pts',(-17.0888052165326,1.45252874415618,5.55111512312578E-16));
#88657=CARTESIAN_POINT('Ctrl Pts',(-17.1458140481676,1.38619227911315,7.37687959281939E-15));
#88658=CARTESIAN_POINT('Ctrl Pts',(-17.1991893647422,1.31687222639765,2.56418979808053E-15));
#88659=CARTESIAN_POINT('Ctrl Pts',(-17.248906462824,1.2449490318139,4.32986979603811E-15));
#88660=CARTESIAN_POINT('Ctrl Pts',(-17.2986235609058,1.17302583723014,6.09554979399569E-15));
#88661=CARTESIAN_POINT('Ctrl Pts',(-17.3446828102636,1.0984987783709,-1.52152896675314E-14));
#88662=CARTESIAN_POINT('Ctrl Pts',(-17.3870269326305,1.02170734003083,3.60822483003176E-15));
#88663=CARTESIAN_POINT('Ctrl Pts',(-17.4058873037742,0.987503891079739,
1.2409471833211E-14));
#88664=CARTESIAN_POINT('Ctrl Pts',(-17.4240101750898,0.952850740415537,
3.4423633586001E-15));
#88665=CARTESIAN_POINT('Ctrl Pts',(-17.4413881058322,0.917775853446501,
5.38458166943201E-15));
#88666=CARTESIAN_POINT('Ctrl Pts',(-17.4513058511744,0.897758291976046,
5.60200919146819E-15));
#88667=CARTESIAN_POINT('Ctrl Pts',(-17.46098093459,0.877603346645284,-6.31318460618514E-15));
#88668=CARTESIAN_POINT('Ctrl Pts',(-17.4704117404408,0.857316068638549,
9.10382880192628E-15));
#88669=CARTESIAN_POINT('Ctrl Pts',(-17.4789447397411,0.838960126232735,
2.33069113036751E-14));
#88670=CARTESIAN_POINT('Ctrl Pts',(-17.487280152406,0.820490076428732,2.08670932036952E-15));
#88671=CARTESIAN_POINT('Ctrl Pts',(-17.4954030423954,0.801941576312626,
1.94289029309402E-15));
#88672=CARTESIAN_POINT('Ctrl Pts',(-17.5319934072411,0.718388015021337,
5.95226537027127E-15));
#88673=CARTESIAN_POINT('Ctrl Pts',(-17.5643214537022,0.633150687238601,
-2.25382967220231E-15));
#88674=CARTESIAN_POINT('Ctrl Pts',(-17.5923614732256,0.546628042515336,
-3.60822483003176E-16));
#88675=CARTESIAN_POINT('Ctrl Pts',(-17.620946200851,0.45842460061771,1.56895844496494E-15));
#88676=CARTESIAN_POINT('Ctrl Pts',(-17.6450752028303,0.368884674071994,
1.05952475446301E-14));
#88677=CARTESIAN_POINT('Ctrl Pts',(-17.6646817382536,0.27839288405896,-2.4980018054066E-15));
#88678=CARTESIAN_POINT('Ctrl Pts',(-17.6835942516363,0.191104275812135,
-1.51277830599129E-14));
#88679=CARTESIAN_POINT('Ctrl Pts',(-17.6982989201074,0.102929065387191,
2.12943541496529E-15));
#88680=CARTESIAN_POINT('Ctrl Pts',(-17.7086953392783,0.0141907563767871,
1.85129689356245E-14));
#88681=CARTESIAN_POINT('Ctrl Pts',(-17.7130454620842,-0.0229395800818436,
2.51856927009412E-14));
#88682=CARTESIAN_POINT('Ctrl Pts',(-17.7166407888389,-0.0601686928876673,
-1.4138599521916E-14));
#88683=CARTESIAN_POINT('Ctrl Pts',(-17.7194716665222,-0.097473490465065,
-9.43689570931383E-16));
#88684=CARTESIAN_POINT('Ctrl Pts',(-17.7212345778386,-0.120704819105844,
8.3900268464302E-15));
#88685=CARTESIAN_POINT('Ctrl Pts',(-17.7227010007055,-0.143965504348453,
-8.36712539882551E-16));
#88686=CARTESIAN_POINT('Ctrl Pts',(-17.7238683201636,-0.167250001102472,
-1.55431223447522E-15));
#88687=CARTESIAN_POINT('Ctrl Pts',(-17.7245283574458,-0.180415750931591,
-1.24461677816766E-15));
#88688=CARTESIAN_POINT('Ctrl Pts',(-17.7250925403628,-0.193585457009226,
2.21190068117789E-14));
#88689=CARTESIAN_POINT('Ctrl Pts',(-17.725560351488,-0.206749836717094,
1.77913239696181E-14));
#88690=CARTESIAN_POINT('Ctrl Pts',(-17.7290270823131,-0.304304936341103,
-1.4429952586954E-14));
#88691=CARTESIAN_POINT('Ctrl Pts',(-17.727212492657,-0.401699033310844,
1.01779328159474E-14));
#88692=CARTESIAN_POINT('Ctrl Pts',(-17.7200504111944,-0.49850402811495,
1.18793863634892E-14));
#88693=CARTESIAN_POINT('Ctrl Pts',(-17.7128883297318,-0.595309022919056,
1.35808399110309E-14));
#88694=CARTESIAN_POINT('Ctrl Pts',(-17.7003792037265,-0.691525995360089,
-4.23206517640884E-15));
#88695=CARTESIAN_POINT('Ctrl Pts',(-17.6824029088532,-0.786746213105208,
8.96505092384814E-15));
#88696=CARTESIAN_POINT('Ctrl Pts',(-17.6653041049695,-0.877318371632217,
2.12372231272733E-14));
#88697=CARTESIAN_POINT('Ctrl Pts',(-17.6432589215089,-0.966989690521659,
-1.54789734783363E-14));
#88698=CARTESIAN_POINT('Ctrl Pts',(-17.6165424919579,-1.05552049345646,
-7.16093850883226E-15));
#88699=CARTESIAN_POINT('Ctrl Pts',(-17.6075282349669,-1.08539122928037,
-4.33697939639551E-15));
#88700=CARTESIAN_POINT('Ctrl Pts',(-17.597981751549,-1.11513208950027,7.51971478766754E-15));
#88701=CARTESIAN_POINT('Ctrl Pts',(-17.5879123011937,-1.14473368418595,
1.20459198171829E-14));
#88702=CARTESIAN_POINT('Ctrl Pts',(-17.5808648207303,-1.16545146448869,
1.54804001547866E-14));
#88703=CARTESIAN_POINT('Ctrl Pts',(-17.5735611555087,-1.1861010242255,9.98355734190746E-15));
#88704=CARTESIAN_POINT('Ctrl Pts',(-17.5660042990016,-1.20667909739138,
3.21964677141295E-15));
#88705=CARTESIAN_POINT('Ctrl Pts',(-17.5600071842001,-1.22300983849439,
-7.11688844300461E-16));
#88706=CARTESIAN_POINT('Ctrl Pts',(-17.5538497320983,-1.23929751690581,
-1.68476118315156E-14));
#88707=CARTESIAN_POINT('Ctrl Pts',(-17.5475420423564,-1.25551905437909,
-1.72917236085368E-14));
#88708=CARTESIAN_POINT('Ctrl Pts',(-17.5132465490965,-1.34371705584084,
-1.96380407135397E-14));
#88709=CARTESIAN_POINT('Ctrl Pts',(-17.4744646972321,-1.43009866043064,
1.43722529900561E-14));
#88710=CARTESIAN_POINT('Ctrl Pts',(-17.43154004082,-1.51442123477835,-1.56819002228303E-15));
#88711=CARTESIAN_POINT('Ctrl Pts',(-17.3877761877647,-1.60039235397788,
-1.78202759780103E-14));
#88712=CARTESIAN_POINT('Ctrl Pts',(-17.33970567815,-1.68422386311186,1.23918828811253E-14));
#88713=CARTESIAN_POINT('Ctrl Pts',(-17.287637320799,-1.76565556503101,1.47937218031302E-14));
#88714=CARTESIAN_POINT('Ctrl Pts',(-17.2347023313771,-1.84844262609836,
1.72355372241975E-14));
#88715=CARTESIAN_POINT('Ctrl Pts',(-17.1776349430471,-1.92875015855361,
-1.93269493324719E-14));
#88716=CARTESIAN_POINT('Ctrl Pts',(-17.1167080019645,-2.00628981398242,
-3.01147995429574E-15));
#88717=CARTESIAN_POINT('Ctrl Pts',(-17.0750658899882,-2.05928632023397,
8.13975447041079E-15));
#88718=CARTESIAN_POINT('Ctrl Pts',(-17.0316197473168,-2.11098953163262,
1.7035584047563E-14));
#88719=CARTESIAN_POINT('Ctrl Pts',(-16.9864445796982,-2.16130036145114,
-7.91033905045424E-15));
#88720=CARTESIAN_POINT('Ctrl Pts',(-16.9750502370955,-2.1739900505392,-1.38695344460067E-14));
#88721=CARTESIAN_POINT('Ctrl Pts',(-16.9635450746152,-2.18659184950728,
8.43307920884399E-15));
#88722=CARTESIAN_POINT('Ctrl Pts',(-16.9519420608097,-2.19909166493364,
7.02216063075412E-15));
#88723=CARTESIAN_POINT('Ctrl Pts',(-16.8830341001199,-2.27332554972167,
5.36559748977514E-15));
#88724=CARTESIAN_POINT('Ctrl Pts',(-16.8105868818959,-2.34406823608281,
-1.1330177174295E-14));
#88725=CARTESIAN_POINT('Ctrl Pts',(-16.7349149176776,-2.41102639673002,
9.5062846483529E-16));
#88726=CARTESIAN_POINT('Ctrl Pts',(-16.6721146507219,-2.46659506614334,
1.11424859187091E-14));
#88727=CARTESIAN_POINT('Ctrl Pts',(-16.6070922800123,-2.51955717048407,
-1.28803071769255E-14));
#88728=CARTESIAN_POINT('Ctrl Pts',(-16.540004026716,-2.56973135519324,-2.81719092498633E-15));
#88729=CARTESIAN_POINT('Ctrl Pts',(-16.5180621279249,-2.58614133501416,
7.74249547919683E-16));
#88730=CARTESIAN_POINT('Ctrl Pts',(-16.4958990909677,-2.60225297300387,
-1.44049204168221E-14));
#88731=CARTESIAN_POINT('Ctrl Pts',(-16.4735199526406,-2.6180595362301,-9.70751257156621E-15));
#88732=CARTESIAN_POINT('Ctrl Pts',(-16.4507971782547,-2.63410881233516,
-4.9290554849159E-15));
#88733=CARTESIAN_POINT('Ctrl Pts',(-16.4278462339836,-2.6498469795081,-7.75945777818769E-15));
#88734=CARTESIAN_POINT('Ctrl Pts',(-16.4047014060989,-2.665247841993,-4.21190859967169E-15));
#88735=CARTESIAN_POINT('Ctrl Pts',(-16.3197410998749,-2.72178150901134,
4.39253025563897E-15));
#88736=CARTESIAN_POINT('Ctrl Pts',(-16.2321163764551,-2.77381420003328,
7.07843165188934E-15));
#88737=CARTESIAN_POINT('Ctrl Pts',(-16.1421182517312,-2.82103740901375,
4.30211422042248E-15));
#88738=CARTESIAN_POINT('Ctrl Pts',(-16.0583441130202,-2.86499481003348,
3.70832056865613E-15));
#88739=CARTESIAN_POINT('Ctrl Pts',(-15.972512690405,-2.90478523590151,6.95277630882711E-15));
#88740=CARTESIAN_POINT('Ctrl Pts',(-15.8848307375281,-2.94013040334526,
1.80411241501588E-15));
#88741=CARTESIAN_POINT('Ctrl Pts',(-15.8553931216106,-2.95199689844043,
-3.55731478892838E-16));
#88742=CARTESIAN_POINT('Ctrl Pts',(-15.8257467255492,-2.96336206503325,
5.1534732236655E-15));
#88743=CARTESIAN_POINT('Ctrl Pts',(-15.7959031959514,-2.9742292935539,1.50227053019591E-15));
#88744=CARTESIAN_POINT('Origin',(0.,0.,3.));
#88745=CARTESIAN_POINT('',(-11.,1.34711147906209E-15,0.));
#88746=CARTESIAN_POINT('',(-11.,1.34711147906209E-15,3.));
#88747=CARTESIAN_POINT('Origin',(0.,0.,0.));
#88748=CARTESIAN_POINT('Origin',(25.,30.,0.));
#88749=CARTESIAN_POINT('',(25.,30.,0.));
#88750=CARTESIAN_POINT('',(-25.,30.,0.));
#88751=CARTESIAN_POINT('',(25.,30.,0.));
#88752=CARTESIAN_POINT('',(-25.,30.,0.));
#88753=CARTESIAN_POINT('',(25.,30.,0.));
#88754=CARTESIAN_POINT('Origin',(25.,-30.,0.));
#88755=CARTESIAN_POINT('',(25.,-30.,0.));
#88756=CARTESIAN_POINT('',(25.,-30.,0.));
#88757=CARTESIAN_POINT('',(25.,-30.,0.));
#88758=CARTESIAN_POINT('Origin',(-25.,-30.,0.));
#88759=CARTESIAN_POINT('',(-25.,-30.,0.));
#88760=CARTESIAN_POINT('',(-25.,-30.,0.));
#88761=CARTESIAN_POINT('',(-25.,-30.,0.));
#88762=CARTESIAN_POINT('Origin',(-25.,30.,0.));
#88763=CARTESIAN_POINT('',(-25.,30.,0.));
#88764=CARTESIAN_POINT('Origin',(0.,0.,0.));
#105786=UNCERTAINTY_MEASURE_WITH_UNIT(LENGTH_MEASURE(0.01),#105807,
'DISTANCE_ACCURACY_VALUE',
'Maximum model space distance between geometric entities at asserted c
onnectivities');
#105792=UNCERTAINTY_MEASURE_WITH_UNIT(LENGTH_MEASURE(0.01),#105807,
'DISTANCE_ACCURACY_VALUE',
'Maximum model space distance between geometric entities at asserted c
onnectivities');
#105800=(
GEOMETRIC_REPRESENTATION_CONTEXT(3)
GLOBAL_UNCERTAINTY_ASSIGNED_CONTEXT((#105786))
GLOBAL_UNIT_ASSIGNED_CONTEXT((#105807,#105809,#105810))
REPRESENTATION_CONTEXT('','3D')
);
#105806=(
GEOMETRIC_REPRESENTATION_CONTEXT(3)
GLOBAL_UNCERTAINTY_ASSIGNED_CONTEXT((#105792))
GLOBAL_UNIT_ASSIGNED_CONTEXT((#105807,#105809,#105810))
REPRESENTATION_CONTEXT('','3D')
);
#105807=(
LENGTH_UNIT()
NAMED_UNIT(*)
SI_UNIT(.MILLI.,.METRE.)
);
#105809=(
NAMED_UNIT(*)
PLANE_ANGLE_UNIT()
SI_UNIT($,.RADIAN.)
);
#105810=(
NAMED_UNIT(*)
SI_UNIT($,.STERADIAN.)
SOLID_ANGLE_UNIT()
);
#105818=SHAPE_DEFINITION_REPRESENTATION(#105831,#105865);
#105831=PRODUCT_DEFINITION_SHAPE('',$,#105879);
#105865=SHAPE_REPRESENTATION('',(#7583),#105800);
#105871=PRODUCT_DEFINITION_CONTEXT('part definition',#105912,'design');
#105879=PRODUCT_DEFINITION('Jaw pad','Jaw pad',#105892,#105871);
#105892=PRODUCT_DEFINITION_FORMATION('',$,#105921);
#105912=APPLICATION_CONTEXT(
'Core Data for Automotive Mechanical Design Process');
#105913=PRODUCT_CONTEXT('part definition',#105912,'mechanical');
#105921=PRODUCT('Jaw pad','Jaw pad',$,(#105913));
#105930=PRESENTATION_STYLE_ASSIGNMENT((#105936));
#105936=SURFACE_STYLE_USAGE(.BOTH.,#105942);
#105942=SURFACE_SIDE_STYLE('',(#105948));
#105948=SURFACE_STYLE_FILL_AREA(#105954);
#105954=FILL_AREA_STYLE('Opaque(185,192,202)',(#105960));
#105960=FILL_AREA_STYLE_COLOUR('Opaque(185,192,202)',#105966);
#105966=COLOUR_RGB('Opaque(185,192,202)',0.725490196078431,0.752941176470588,
0.792156862745098);
ENDSEC;
END-ISO-10303-21;
